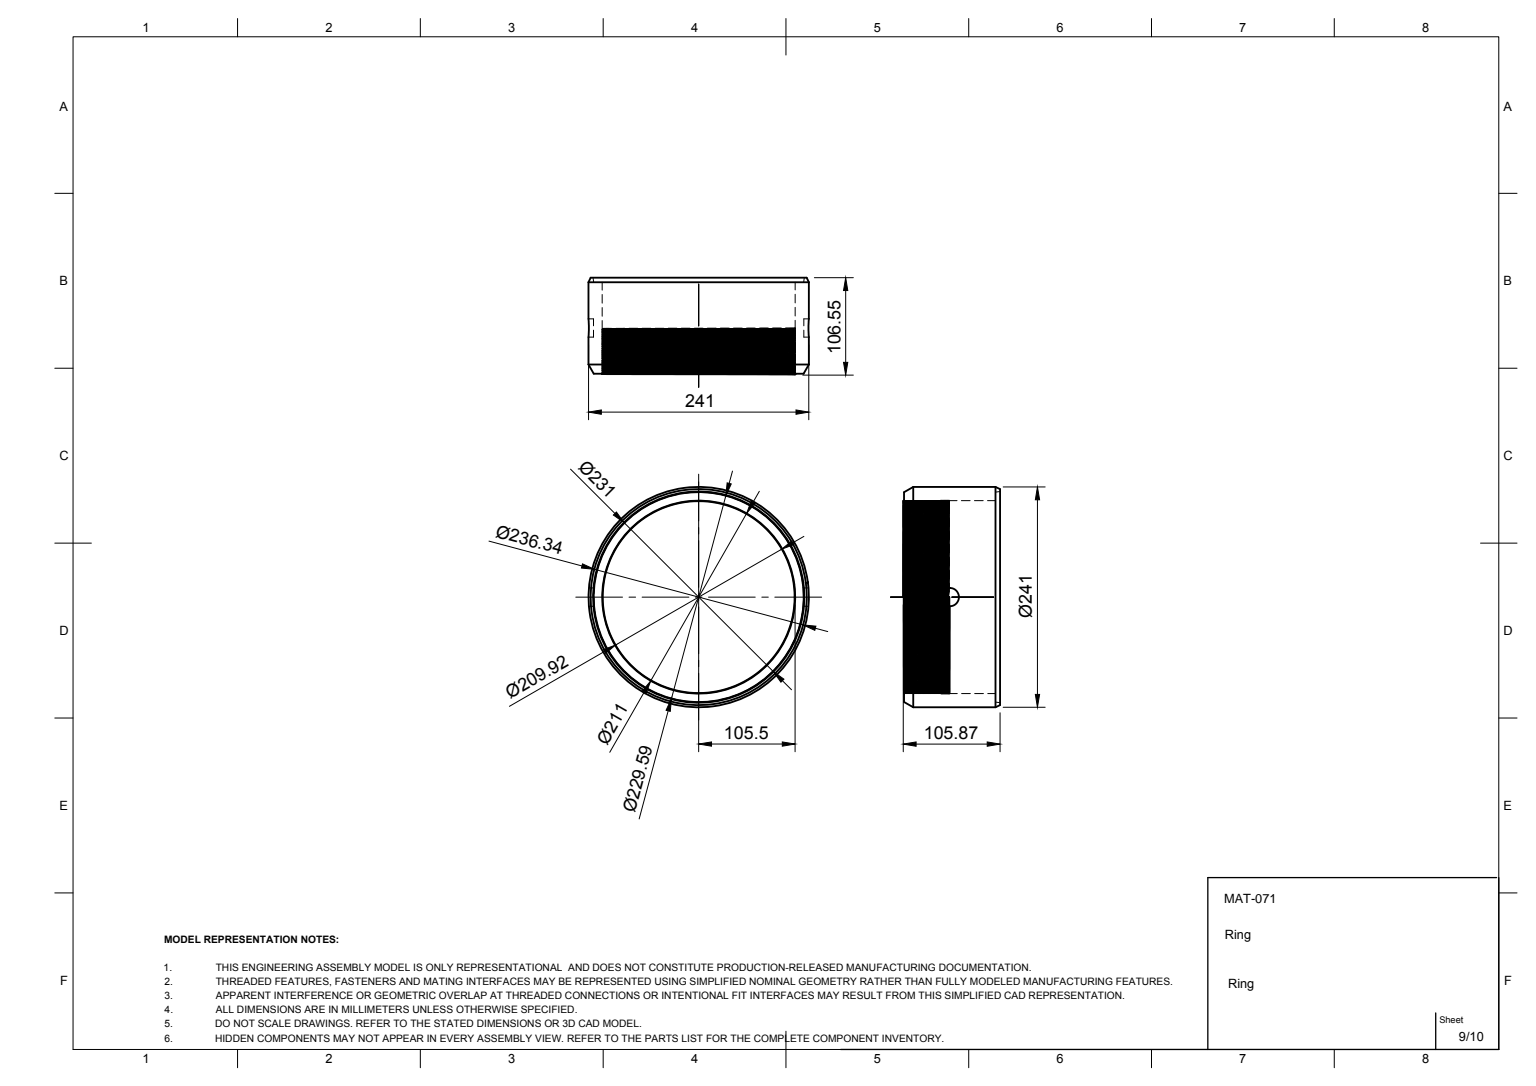
ISO-10303-21;
HEADER;
/* Generated by software containing ST-Developer
 * from STEP Tools, Inc. (www.steptools.com) 
 */

FILE_DESCRIPTION(
/* description */ (''),
/* implementation_level */ '2;1');

FILE_NAME(
/* name */ 'Ring.step',
/* time_stamp */ '2026-10-24T12:24:47-07:00',
/* author */ (''),
/* organization */ (''),
/* preprocessor_version */ 'ST-DEVELOPER v20.2',
/* originating_system */ 'Autodesk Translation Framework v15.15.0.0',
/* authorisation */ '');

FILE_SCHEMA (('AUTOMOTIVE_DESIGN { 1 0 10303 214 3 1 1 }'));
ENDSEC;

DATA;
#10=MECHANICAL_DESIGN_GEOMETRIC_PRESENTATION_REPRESENTATION('',(#57),#13594);
#45=SHAPE_REPRESENTATION_RELATIONSHIP('SRR','None',#13625,#51);
#51=ADVANCED_BREP_SHAPE_REPRESENTATION('',(#63),#13588);
#57=STYLED_ITEM('',(#13667),#63);
#63=MANIFOLD_SOLID_BREP('Ring',#2964);
#69=(
BOUNDED_SURFACE()
B_SPLINE_SURFACE(1,2,((#7782,#7783,#7784,#7785,#7786,#7787,#7788,#7789,
#7790,#7791,#7792,#7793,#7794,#7795,#7796,#7797,#7798,#7799,#7800,#7801,
#7802,#7803,#7804,#7805,#7806,#7807,#7808,#7809,#7810,#7811,#7812,#7813,
#7814,#7815,#7816,#7817,#7818,#7819,#7820,#7821,#7822,#7823,#7824,#7825,
#7826,#7827,#7828,#7829,#7830,#7831,#7832,#7833,#7834,#7835,#7836,#7837,
#7838,#7839,#7840,#7841,#7842,#7843,#7844,#7845,#7846,#7847,#7848,#7849,
#7850,#7851,#7852,#7853,#7854,#7855,#7856,#7857,#7858,#7859,#7860,#7861,
#7862,#7863,#7864,#7865,#7866,#7867,#7868,#7869,#7870,#7871,#7872,#7873,
#7874,#7875,#7876,#7877,#7878,#7879,#7880,#7881,#7882,#7883,#7884,#7885,
#7886,#7887,#7888,#7889,#7890,#7891,#7892,#7893,#7894,#7895,#7896,#7897,
#7898,#7899,#7900,#7901,#7902,#7903,#7904,#7905,#7906,#7907,#7908,#7909,
#7910,#7911,#7912,#7913,#7914,#7915,#7916,#7917,#7918,#7919,#7920,#7921,
#7922,#7923,#7924,#7925,#7926,#7927,#7928,#7929,#7930,#7931,#7932,#7933,
#7934,#7935,#7936,#7937,#7938,#7939,#7940,#7941,#7942,#7943,#7944,#7945,
#7946,#7947,#7948,#7949,#7950,#7951,#7952,#7953,#7954,#7955,#7956,#7957,
#7958,#7959,#7960,#7961,#7962,#7963,#7964,#7965,#7966,#7967,#7968,#7969,
#7970,#7971,#7972,#7973,#7974,#7975,#7976,#7977,#7978,#7979,#7980,#7981,
#7982,#7983,#7984,#7985,#7986,#7987,#7988,#7989,#7990,#7991,#7992,#7993,
#7994,#7995,#7996,#7997,#7998,#7999,#8000,#8001,#8002,#8003,#8004,#8005,
#8006,#8007,#8008,#8009,#8010,#8011,#8012,#8013,#8014,#8015,#8016,#8017,
#8018,#8019,#8020,#8021,#8022,#8023,#8024,#8025,#8026,#8027,#8028,#8029,
#8030,#8031,#8032,#8033,#8034,#8035,#8036,#8037,#8038,#8039,#8040,#8041,
#8042,#8043,#8044,#8045,#8046,#8047,#8048,#8049,#8050,#8051,#8052,#8053,
#8054,#8055,#8056,#8057,#8058,#8059,#8060,#8061,#8062,#8063,#8064,#8065,
#8066,#8067,#8068,#8069,#8070,#8071,#8072,#8073,#8074,#8075,#8076,#8077,
#8078,#8079,#8080,#8081,#8082,#8083,#8084,#8085,#8086,#8087,#8088,#8089,
#8090,#8091,#8092,#8093,#8094,#8095,#8096,#8097,#8098,#8099,#8100,#8101,
#8102,#8103,#8104,#8105,#8106,#8107,#8108,#8109,#8110,#8111,#8112,#8113,
#8114,#8115,#8116,#8117,#8118,#8119,#8120,#8121,#8122,#8123,#8124,#8125,
#8126,#8127,#8128,#8129,#8130,#8131,#8132,#8133,#8134,#8135,#8136,#8137,
#8138,#8139,#8140,#8141,#8142,#8143,#8144,#8145,#8146,#8147,#8148,#8149,
#8150,#8151,#8152,#8153,#8154,#8155,#8156,#8157,#8158,#8159,#8160,#8161,
#8162,#8163,#8164,#8165,#8166,#8167,#8168,#8169,#8170,#8171,#8172,#8173,
#8174,#8175,#8176,#8177,#8178,#8179,#8180,#8181,#8182,#8183,#8184,#8185,
#8186,#8187,#8188,#8189,#8190,#8191,#8192,#8193,#8194,#8195,#8196,#8197,
#8198,#8199,#8200,#8201,#8202,#8203,#8204,#8205,#8206,#8207,#8208,#8209,
#8210,#8211,#8212,#8213,#8214,#8215,#8216,#8217,#8218,#8219,#8220,#8221,
#8222,#8223,#8224,#8225,#8226,#8227,#8228,#8229,#8230,#8231,#8232,#8233,
#8234,#8235,#8236,#8237,#8238,#8239,#8240,#8241,#8242,#8243,#8244,#8245,
#8246,#8247,#8248,#8249,#8250,#8251,#8252,#8253,#8254,#8255,#8256,#8257,
#8258,#8259,#8260,#8261,#8262,#8263,#8264,#8265,#8266,#8267,#8268,#8269,
#8270,#8271,#8272,#8273,#8274,#8275,#8276,#8277,#8278,#8279,#8280,#8281,
#8282,#8283,#8284,#8285,#8286,#8287,#8288,#8289,#8290,#8291,#8292,#8293,
#8294,#8295,#8296,#8297,#8298,#8299,#8300,#8301,#8302,#8303,#8304,#8305,
#8306,#8307,#8308,#8309,#8310,#8311,#8312,#8313,#8314,#8315,#8316,#8317,
#8318,#8319,#8320,#8321,#8322,#8323,#8324,#8325,#8326,#8327,#8328,#8329,
#8330,#8331,#8332,#8333,#8334,#8335,#8336,#8337,#8338,#8339,#8340,#8341,
#8342,#8343,#8344,#8345,#8346,#8347,#8348,#8349,#8350,#8351,#8352,#8353,
#8354,#8355,#8356,#8357,#8358,#8359,#8360,#8361,#8362,#8363,#8364,#8365,
#8366,#8367,#8368,#8369,#8370,#8371,#8372,#8373,#8374,#8375,#8376,#8377,
#8378,#8379,#8380,#8381,#8382,#8383,#8384,#8385,#8386,#8387,#8388,#8389,
#8390,#8391,#8392,#8393,#8394,#8395,#8396,#8397,#8398,#8399,#8400,#8401,
#8402,#8403,#8404,#8405,#8406,#8407,#8408,#8409,#8410,#8411,#8412,#8413,
#8414,#8415,#8416,#8417,#8418,#8419,#8420,#8421,#8422,#8423,#8424,#8425,
#8426,#8427,#8428,#8429,#8430,#8431,#8432,#8433,#8434,#8435,#8436,#8437,
#8438,#8439,#8440,#8441,#8442,#8443,#8444,#8445,#8446,#8447,#8448,#8449,
#8450,#8451,#8452,#8453,#8454,#8455,#8456,#8457,#8458,#8459,#8460,#8461,
#8462,#8463,#8464,#8465,#8466,#8467,#8468,#8469,#8470,#8471,#8472,#8473,
#8474,#8475,#8476,#8477,#8478,#8479,#8480,#8481,#8482,#8483,#8484,#8485,
#8486,#8487,#8488,#8489,#8490,#8491,#8492,#8493,#8494,#8495,#8496,#8497,
#8498,#8499,#8500,#8501,#8502,#8503,#8504,#8505,#8506,#8507,#8508,#8509,
#8510,#8511,#8512,#8513,#8514,#8515,#8516,#8517,#8518,#8519,#8520,#8521,
#8522,#8523,#8524,#8525,#8526,#8527,#8528,#8529,#8530,#8531,#8532,#8533,
#8534,#8535,#8536,#8537,#8538,#8539,#8540,#8541,#8542,#8543,#8544,#8545,
#8546,#8547,#8548,#8549,#8550,#8551,#8552,#8553,#8554,#8555,#8556,#8557,
#8558,#8559,#8560,#8561,#8562,#8563,#8564,#8565,#8566,#8567,#8568,#8569,
#8570,#8571,#8572,#8573,#8574,#8575,#8576,#8577,#8578,#8579,#8580,#8581,
#8582),(#8583,#8584,#8585,#8586,#8587,#8588,#8589,#8590,#8591,#8592,#8593,
#8594,#8595,#8596,#8597,#8598,#8599,#8600,#8601,#8602,#8603,#8604,#8605,
#8606,#8607,#8608,#8609,#8610,#8611,#8612,#8613,#8614,#8615,#8616,#8617,
#8618,#8619,#8620,#8621,#8622,#8623,#8624,#8625,#8626,#8627,#8628,#8629,
#8630,#8631,#8632,#8633,#8634,#8635,#8636,#8637,#8638,#8639,#8640,#8641,
#8642,#8643,#8644,#8645,#8646,#8647,#8648,#8649,#8650,#8651,#8652,#8653,
#8654,#8655,#8656,#8657,#8658,#8659,#8660,#8661,#8662,#8663,#8664,#8665,
#8666,#8667,#8668,#8669,#8670,#8671,#8672,#8673,#8674,#8675,#8676,#8677,
#8678,#8679,#8680,#8681,#8682,#8683,#8684,#8685,#8686,#8687,#8688,#8689,
#8690,#8691,#8692,#8693,#8694,#8695,#8696,#8697,#8698,#8699,#8700,#8701,
#8702,#8703,#8704,#8705,#8706,#8707,#8708,#8709,#8710,#8711,#8712,#8713,
#8714,#8715,#8716,#8717,#8718,#8719,#8720,#8721,#8722,#8723,#8724,#8725,
#8726,#8727,#8728,#8729,#8730,#8731,#8732,#8733,#8734,#8735,#8736,#8737,
#8738,#8739,#8740,#8741,#8742,#8743,#8744,#8745,#8746,#8747,#8748,#8749,
#8750,#8751,#8752,#8753,#8754,#8755,#8756,#8757,#8758,#8759,#8760,#8761,
#8762,#8763,#8764,#8765,#8766,#8767,#8768,#8769,#8770,#8771,#8772,#8773,
#8774,#8775,#8776,#8777,#8778,#8779,#8780,#8781,#8782,#8783,#8784,#8785,
#8786,#8787,#8788,#8789,#8790,#8791,#8792,#8793,#8794,#8795,#8796,#8797,
#8798,#8799,#8800,#8801,#8802,#8803,#8804,#8805,#8806,#8807,#8808,#8809,
#8810,#8811,#8812,#8813,#8814,#8815,#8816,#8817,#8818,#8819,#8820,#8821,
#8822,#8823,#8824,#8825,#8826,#8827,#8828,#8829,#8830,#8831,#8832,#8833,
#8834,#8835,#8836,#8837,#8838,#8839,#8840,#8841,#8842,#8843,#8844,#8845,
#8846,#8847,#8848,#8849,#8850,#8851,#8852,#8853,#8854,#8855,#8856,#8857,
#8858,#8859,#8860,#8861,#8862,#8863,#8864,#8865,#8866,#8867,#8868,#8869,
#8870,#8871,#8872,#8873,#8874,#8875,#8876,#8877,#8878,#8879,#8880,#8881,
#8882,#8883,#8884,#8885,#8886,#8887,#8888,#8889,#8890,#8891,#8892,#8893,
#8894,#8895,#8896,#8897,#8898,#8899,#8900,#8901,#8902,#8903,#8904,#8905,
#8906,#8907,#8908,#8909,#8910,#8911,#8912,#8913,#8914,#8915,#8916,#8917,
#8918,#8919,#8920,#8921,#8922,#8923,#8924,#8925,#8926,#8927,#8928,#8929,
#8930,#8931,#8932,#8933,#8934,#8935,#8936,#8937,#8938,#8939,#8940,#8941,
#8942,#8943,#8944,#8945,#8946,#8947,#8948,#8949,#8950,#8951,#8952,#8953,
#8954,#8955,#8956,#8957,#8958,#8959,#8960,#8961,#8962,#8963,#8964,#8965,
#8966,#8967,#8968,#8969,#8970,#8971,#8972,#8973,#8974,#8975,#8976,#8977,
#8978,#8979,#8980,#8981,#8982,#8983,#8984,#8985,#8986,#8987,#8988,#8989,
#8990,#8991,#8992,#8993,#8994,#8995,#8996,#8997,#8998,#8999,#9000,#9001,
#9002,#9003,#9004,#9005,#9006,#9007,#9008,#9009,#9010,#9011,#9012,#9013,
#9014,#9015,#9016,#9017,#9018,#9019,#9020,#9021,#9022,#9023,#9024,#9025,
#9026,#9027,#9028,#9029,#9030,#9031,#9032,#9033,#9034,#9035,#9036,#9037,
#9038,#9039,#9040,#9041,#9042,#9043,#9044,#9045,#9046,#9047,#9048,#9049,
#9050,#9051,#9052,#9053,#9054,#9055,#9056,#9057,#9058,#9059,#9060,#9061,
#9062,#9063,#9064,#9065,#9066,#9067,#9068,#9069,#9070,#9071,#9072,#9073,
#9074,#9075,#9076,#9077,#9078,#9079,#9080,#9081,#9082,#9083,#9084,#9085,
#9086,#9087,#9088,#9089,#9090,#9091,#9092,#9093,#9094,#9095,#9096,#9097,
#9098,#9099,#9100,#9101,#9102,#9103,#9104,#9105,#9106,#9107,#9108,#9109,
#9110,#9111,#9112,#9113,#9114,#9115,#9116,#9117,#9118,#9119,#9120,#9121,
#9122,#9123,#9124,#9125,#9126,#9127,#9128,#9129,#9130,#9131,#9132,#9133,
#9134,#9135,#9136,#9137,#9138,#9139,#9140,#9141,#9142,#9143,#9144,#9145,
#9146,#9147,#9148,#9149,#9150,#9151,#9152,#9153,#9154,#9155,#9156,#9157,
#9158,#9159,#9160,#9161,#9162,#9163,#9164,#9165,#9166,#9167,#9168,#9169,
#9170,#9171,#9172,#9173,#9174,#9175,#9176,#9177,#9178,#9179,#9180,#9181,
#9182,#9183,#9184,#9185,#9186,#9187,#9188,#9189,#9190,#9191,#9192,#9193,
#9194,#9195,#9196,#9197,#9198,#9199,#9200,#9201,#9202,#9203,#9204,#9205,
#9206,#9207,#9208,#9209,#9210,#9211,#9212,#9213,#9214,#9215,#9216,#9217,
#9218,#9219,#9220,#9221,#9222,#9223,#9224,#9225,#9226,#9227,#9228,#9229,
#9230,#9231,#9232,#9233,#9234,#9235,#9236,#9237,#9238,#9239,#9240,#9241,
#9242,#9243,#9244,#9245,#9246,#9247,#9248,#9249,#9250,#9251,#9252,#9253,
#9254,#9255,#9256,#9257,#9258,#9259,#9260,#9261,#9262,#9263,#9264,#9265,
#9266,#9267,#9268,#9269,#9270,#9271,#9272,#9273,#9274,#9275,#9276,#9277,
#9278,#9279,#9280,#9281,#9282,#9283,#9284,#9285,#9286,#9287,#9288,#9289,
#9290,#9291,#9292,#9293,#9294,#9295,#9296,#9297,#9298,#9299,#9300,#9301,
#9302,#9303,#9304,#9305,#9306,#9307,#9308,#9309,#9310,#9311,#9312,#9313,
#9314,#9315,#9316,#9317,#9318,#9319,#9320,#9321,#9322,#9323,#9324,#9325,
#9326,#9327,#9328,#9329,#9330,#9331,#9332,#9333,#9334,#9335,#9336,#9337,
#9338,#9339,#9340,#9341,#9342,#9343,#9344,#9345,#9346,#9347,#9348,#9349,
#9350,#9351,#9352,#9353,#9354,#9355,#9356,#9357,#9358,#9359,#9360,#9361,
#9362,#9363,#9364,#9365,#9366,#9367,#9368,#9369,#9370,#9371,#9372,#9373,
#9374,#9375,#9376,#9377,#9378,#9379,#9380,#9381,#9382,#9383)),
 .UNSPECIFIED.,.F.,.F.,.F.)
B_SPLINE_SURFACE_WITH_KNOTS((2,2),(3,2,2,2,2,2,2,2,2,2,2,2,2,2,2,2,2,2,
2,2,2,2,2,2,2,2,2,2,2,2,2,2,2,2,2,2,2,2,2,2,2,2,2,2,2,2,2,2,2,2,2,2,2,2,
2,2,2,2,2,2,2,2,2,2,2,2,2,2,2,2,2,2,2,2,2,2,2,2,2,2,2,2,2,2,2,2,2,2,2,2,
2,2,2,2,2,2,2,2,2,2,2,2,2,2,2,2,2,2,2,2,2,2,2,2,2,2,2,2,2,2,2,2,2,2,2,2,
2,2,2,2,2,2,2,2,2,2,2,2,2,2,2,2,2,2,2,2,2,2,2,2,2,2,2,2,2,2,2,2,2,2,2,2,
2,2,2,2,2,2,2,2,2,2,2,2,2,2,2,2,2,2,2,2,2,2,2,2,2,2,2,2,2,2,2,2,2,2,2,2,
2,2,2,2,2,2,2,2,2,2,2,2,2,2,2,2,2,2,2,2,2,2,2,2,2,2,2,2,2,2,2,2,2,2,2,2,
2,2,2,2,2,2,2,2,2,2,2,2,2,2,2,2,2,2,2,2,2,2,2,2,2,2,2,2,2,2,2,2,2,2,2,2,
2,2,2,2,2,2,2,2,2,2,2,2,2,2,2,2,2,2,2,2,2,2,2,2,2,2,2,2,2,2,2,2,2,2,2,2,
2,2,2,2,2,2,2,2,2,2,2,2,2,2,2,2,2,2,2,2,2,2,2,2,2,2,2,2,2,2,2,2,2,2,2,2,
2,2,2,2,2,2,2,2,2,2,2,2,2,2,2,2,2,2,2,2,2,2,2,2,2,2,2,2,2,2,2,2,2,2,2,2,
2,2,2,2,2,2,2,2,2,2,2,2,2,2,2,2,2,2,2,2,2,2,3),(0.,1.),(0.,0.0025,0.005,
0.0075,0.01,0.0125,0.015,0.0175,0.02,0.0225,0.025,0.0275,0.03,0.0325,0.035,
0.0375,0.04,0.0425,0.045,0.0475,0.05,0.0525,0.055,0.0575,0.06,0.0625,0.065,
0.0675,0.07,0.0725,0.075,0.0775,0.08,0.0825,0.085,0.0875,0.09,0.0925,0.095,
0.0975,0.1,0.1025,0.105,0.1075,0.11,0.1125,0.115,0.1175,0.12,0.1225,0.125,
0.1275,0.13,0.1325,0.135,0.1375,0.14,0.1425,0.145,0.1475,0.15,0.1525,0.155,
0.1575,0.16,0.1625,0.165,0.1675,0.17,0.1725,0.175,0.1775,0.18,0.1825,0.185,
0.1875,0.19,0.1925,0.195,0.1975,0.2,0.2025,0.205,0.2075,0.21,0.2125,0.215,
0.2175,0.22,0.2225,0.225,0.2275,0.23,0.2325,0.235,0.2375,0.24,0.2425,0.245,
0.2475,0.25,0.2525,0.255,0.2575,0.26,0.2625,0.265,0.2675,0.27,0.2725,0.275,
0.2775,0.28,0.2825,0.285,0.2875,0.29,0.2925,0.295,0.2975,0.3,0.3025,0.305,
0.3075,0.31,0.3125,0.315,0.3175,0.32,0.3225,0.325,0.3275,0.33,0.3325,0.335,
0.3375,0.34,0.3425,0.345,0.3475,0.35,0.3525,0.355,0.3575,0.36,0.3625,0.365,
0.3675,0.37,0.3725,0.375,0.3775,0.38,0.3825,0.385,0.3875,0.39,0.3925,0.395,
0.3975,0.4,0.4025,0.405,0.4075,0.41,0.4125,0.415,0.4175,0.42,0.4225,0.425,
0.4275,0.43,0.4325,0.435,0.4375,0.44,0.4425,0.445,0.4475,0.45,0.4525,0.455,
0.4575,0.46,0.4625,0.465,0.4675,0.47,0.4725,0.475,0.4775,0.48,0.4825,0.485,
0.4875,0.49,0.4925,0.495,0.4975,0.5,0.5025,0.505,0.5075,0.51,0.5125,0.515,
0.5175,0.52,0.5225,0.525,0.5275,0.53,0.5325,0.535,0.5375,0.54,0.5425,0.545,
0.5475,0.55,0.5525,0.555,0.5575,0.56,0.5625,0.565,0.5675,0.57,0.5725,0.575,
0.5775,0.58,0.5825,0.585,0.5875,0.59,0.5925,0.595,0.5975,0.6,0.6025,0.605,
0.6075,0.61,0.6125,0.615,0.6175,0.62,0.6225,0.625,0.6275,0.63,0.6325,0.635,
0.6375,0.64,0.6425,0.645,0.6475,0.65,0.6525,0.655,0.6575,0.66,0.6625,0.665,
0.6675,0.67,0.6725,0.675,0.6775,0.68,0.6825,0.685,0.6875,0.69,0.6925,0.695,
0.6975,0.7,0.7025,0.705,0.7075,0.71,0.7125,0.715,0.7175,0.72,0.7225,0.725,
0.7275,0.73,0.7325,0.735,0.7375,0.74,0.7425,0.745,0.7475,0.75,0.7525,0.755,
0.7575,0.76,0.7625,0.765,0.7675,0.77,0.7725,0.775,0.7775,0.78,0.7825,0.785,
0.7875,0.79,0.7925,0.795,0.7975,0.8,0.8025,0.805,0.8075,0.81,0.8125,0.815,
0.8175,0.82,0.8225,0.825,0.8275,0.83,0.8325,0.835,0.8375,0.84,0.8425,0.845,
0.8475,0.85,0.8525,0.855,0.8575,0.86,0.8625,0.865,0.8675,0.87,0.8725,0.875,
0.8775,0.88,0.8825,0.885,0.8875,0.89,0.8925,0.895,0.8975,0.9,0.9025,0.905,
0.9075,0.91,0.9125,0.915,0.9175,0.92,0.9225,0.925,0.9275,0.93,0.9325,0.935,
0.9375,0.94,0.9425,0.945,0.9475,0.95,0.9525,0.955,0.9575,0.96,0.9625,0.965,
0.9675,0.97,0.9725,0.975,0.9775,0.98,0.9825,0.985,0.9875,0.99,0.9925,0.995,
0.9975,1.),.UNSPECIFIED.)
GEOMETRIC_REPRESENTATION_ITEM()
RATIONAL_B_SPLINE_SURFACE(((1.,0.923879532511287,1.,0.923879532511287,1.,
0.923879532511287,1.,0.923879532511287,1.,0.923879532511287,1.,0.923879532511287,
1.,0.923879532511287,1.,0.923879532511287,1.,0.923879532511287,1.,0.923879532511287,
1.,0.923879532511287,1.,0.923879532511287,1.,0.923879532511287,1.,0.923879532511287,
1.,0.923879532511287,1.,0.923879532511287,1.,0.923879532511287,1.,0.923879532511287,
1.,0.923879532511287,1.,0.923879532511287,1.,0.923879532511287,1.,0.923879532511287,
1.,0.923879532511287,1.,0.923879532511287,1.,0.923879532511287,1.,0.923879532511287,
1.,0.923879532511287,1.,0.923879532511287,1.,0.923879532511287,1.,0.923879532511287,
1.,0.923879532511287,1.,0.923879532511287,1.,0.923879532511287,1.,0.923879532511287,
1.,0.923879532511287,1.,0.923879532511287,1.,0.923879532511287,1.,0.923879532511287,
1.,0.923879532511287,1.,0.923879532511287,1.,0.923879532511287,1.,0.923879532511287,
1.,0.923879532511287,1.,0.923879532511287,1.,0.923879532511287,1.,0.923879532511287,
1.,0.923879532511287,1.,0.923879532511287,1.,0.923879532511287,1.,0.923879532511287,
1.,0.923879532511287,1.,0.923879532511287,1.,0.923879532511287,1.,0.923879532511287,
1.,0.923879532511287,1.,0.923879532511287,1.,0.923879532511287,1.,0.923879532511287,
1.,0.923879532511287,1.,0.923879532511287,1.,0.923879532511287,1.,0.923879532511287,
1.,0.923879532511287,1.,0.923879532511287,1.,0.923879532511287,1.,0.923879532511287,
1.,0.923879532511287,1.,0.923879532511287,1.,0.923879532511287,1.,0.923879532511287,
1.,0.923879532511287,1.,0.923879532511287,1.,0.923879532511287,1.,0.923879532511287,
1.,0.923879532511287,1.,0.923879532511287,1.,0.923879532511287,1.,0.923879532511287,
1.,0.923879532511287,1.,0.923879532511287,1.,0.923879532511287,1.,0.923879532511287,
1.,0.923879532511287,1.,0.923879532511287,1.,0.923879532511287,1.,0.923879532511287,
1.,0.923879532511287,1.,0.923879532511287,1.,0.923879532511287,1.,0.923879532511287,
1.,0.923879532511287,1.,0.923879532511287,1.,0.923879532511287,1.,0.923879532511287,
1.,0.923879532511287,1.,0.923879532511287,1.,0.923879532511287,1.,0.923879532511287,
1.,0.923879532511287,1.,0.923879532511287,1.,0.923879532511287,1.,0.923879532511287,
1.,0.923879532511287,1.,0.923879532511287,1.,0.923879532511287,1.,0.923879532511287,
1.,0.923879532511287,1.,0.923879532511287,1.,0.923879532511287,1.,0.923879532511287,
1.,0.923879532511287,1.,0.923879532511287,1.,0.923879532511287,1.,0.923879532511287,
1.,0.923879532511287,1.,0.923879532511287,1.,0.923879532511287,1.,0.923879532511287,
1.,0.923879532511287,1.,0.923879532511287,1.,0.923879532511287,1.,0.923879532511287,
1.,0.923879532511287,1.,0.923879532511287,1.,0.923879532511287,1.,0.923879532511287,
1.,0.923879532511287,1.,0.923879532511287,1.,0.923879532511287,1.,0.923879532511287,
1.,0.923879532511287,1.,0.923879532511287,1.,0.923879532511287,1.,0.923879532511287,
1.,0.923879532511287,1.,0.923879532511287,1.,0.923879532511287,1.,0.923879532511287,
1.,0.923879532511287,1.,0.923879532511287,1.,0.923879532511287,1.,0.923879532511287,
1.,0.923879532511287,1.,0.923879532511287,1.,0.923879532511287,1.,0.923879532511287,
1.,0.923879532511287,1.,0.923879532511287,1.,0.923879532511287,1.,0.923879532511287,
1.,0.923879532511287,1.,0.923879532511287,1.,0.923879532511287,1.,0.923879532511287,
1.,0.923879532511287,1.,0.923879532511287,1.,0.923879532511287,1.,0.923879532511287,
1.,0.923879532511287,1.,0.923879532511287,1.,0.923879532511287,1.,0.923879532511287,
1.,0.923879532511287,1.,0.923879532511287,1.,0.923879532511287,1.,0.923879532511287,
1.,0.923879532511287,1.,0.923879532511287,1.,0.923879532511287,1.,0.923879532511287,
1.,0.923879532511287,1.,0.923879532511287,1.,0.923879532511287,1.,0.923879532511287,
1.,0.923879532511287,1.,0.923879532511287,1.,0.923879532511287,1.,0.923879532511287,
1.,0.923879532511287,1.,0.923879532511287,1.,0.923879532511287,1.,0.923879532511287,
1.,0.923879532511287,1.,0.923879532511287,1.,0.923879532511287,1.,0.923879532511287,
1.,0.923879532511287,1.,0.923879532511287,1.,0.923879532511287,1.,0.923879532511287,
1.,0.923879532511287,1.,0.923879532511287,1.,0.923879532511287,1.,0.923879532511287,
1.,0.923879532511287,1.,0.923879532511287,1.,0.923879532511287,1.,0.923879532511287,
1.,0.923879532511287,1.,0.923879532511287,1.,0.923879532511287,1.,0.923879532511287,
1.,0.923879532511287,1.,0.923879532511287,1.,0.923879532511287,1.,0.923879532511287,
1.,0.923879532511287,1.,0.923879532511287,1.,0.923879532511287,1.,0.923879532511287,
1.,0.923879532511287,1.,0.923879532511287,1.,0.923879532511287,1.,0.923879532511287,
1.,0.923879532511287,1.,0.923879532511287,1.,0.923879532511287,1.,0.923879532511287,
1.,0.923879532511287,1.,0.923879532511287,1.,0.923879532511287,1.,0.923879532511287,
1.,0.923879532511287,1.,0.923879532511287,1.,0.923879532511287,1.,0.923879532511287,
1.,0.923879532511287,1.,0.923879532511287,1.,0.923879532511287,1.,0.923879532511287,
1.,0.923879532511287,1.,0.923879532511287,1.,0.923879532511287,1.,0.923879532511287,
1.,0.923879532511287,1.,0.923879532511287,1.,0.923879532511287,1.,0.923879532511287,
1.,0.923879532511287,1.,0.923879532511287,1.,0.923879532511287,1.,0.923879532511287,
1.,0.923879532511287,1.,0.923879532511287,1.,0.923879532511287,1.,0.923879532511287,
1.,0.923879532511287,1.,0.923879532511287,1.,0.923879532511287,1.,0.923879532511287,
1.,0.923879532511287,1.,0.923879532511287,1.,0.923879532511287,1.,0.923879532511287,
1.,0.923879532511287,1.,0.923879532511287,1.,0.923879532511287,1.,0.923879532511287,
1.,0.923879532511287,1.,0.923879532511287,1.,0.923879532511287,1.,0.923879532511287,
1.,0.923879532511287,1.,0.923879532511287,1.,0.923879532511287,1.,0.923879532511287,
1.,0.923879532511287,1.,0.923879532511287,1.,0.923879532511287,1.,0.923879532511287,
1.,0.923879532511287,1.,0.923879532511287,1.,0.923879532511287,1.,0.923879532511287,
1.,0.923879532511287,1.,0.923879532511287,1.,0.923879532511287,1.,0.923879532511287,
1.,0.923879532511287,1.,0.923879532511287,1.,0.923879532511287,1.,0.923879532511287,
1.,0.923879532511287,1.,0.923879532511287,1.,0.923879532511287,1.,0.923879532511287,
1.,0.923879532511287,1.,0.923879532511287,1.,0.923879532511287,1.,0.923879532511287,
1.,0.923879532511287,1.,0.923879532511287,1.,0.923879532511287,1.,0.923879532511287,
1.,0.923879532511287,1.,0.923879532511287,1.,0.923879532511287,1.,0.923879532511287,
1.,0.923879532511287,1.,0.923879532511287,1.,0.923879532511287,1.,0.923879532511287,
1.,0.923879532511287,1.,0.923879532511287,1.,0.923879532511287,1.,0.923879532511287,
1.,0.923879532511287,1.,0.923879532511287,1.,0.923879532511287,1.,0.923879532511287,
1.,0.923879532511287,1.,0.923879532511287,1.,0.923879532511287,1.,0.923879532511287,
1.,0.923879532511287,1.,0.923879532511287,1.,0.923879532511287,1.,0.923879532511287,
1.,0.923879532511287,1.,0.923879532511287,1.,0.923879532511287,1.,0.923879532511287,
1.,0.923879532511287,1.,0.923879532511287,1.,0.923879532511287,1.,0.923879532511287,
1.,0.923879532511287,1.,0.923879532511287,1.,0.923879532511287,1.,0.923879532511287,
1.,0.923879532511287,1.,0.923879532511287,1.,0.923879532511287,1.,0.923879532511287,
1.,0.923879532511287,1.,0.923879532511287,1.,0.923879532511287,1.,0.923879532511287,
1.,0.923879532511287,1.,0.923879532511287,1.,0.923879532511287,1.,0.923879532511287,
1.,0.923879532511287,1.,0.923879532511287,1.,0.923879532511287,1.,0.923879532511287,
1.,0.923879532511287,1.,0.923879532511287,1.,0.923879532511287,1.,0.923879532511287,
1.,0.923879532511287,1.,0.923879532511287,1.,0.923879532511287,1.,0.923879532511287,
1.,0.923879532511287,1.,0.923879532511287,1.,0.923879532511287,1.,0.923879532511287,
1.,0.923879532511287,1.,0.923879532511287,1.,0.923879532511287,1.,0.923879532511287,
1.,0.923879532511287,1.,0.923879532511287,1.,0.923879532511287,1.,0.923879532511287,
1.,0.923879532511287,1.,0.923879532511287,1.,0.923879532511287,1.,0.923879532511287,
1.,0.923879532511287,1.,0.923879532511287,1.,0.923879532511287,1.,0.923879532511287,
1.,0.923879532511287,1.,0.923879532511287,1.,0.923879532511287,1.,0.923879532511287,
1.,0.923879532511287,1.,0.923879532511287,1.,0.923879532511287,1.,0.923879532511287,
1.,0.923879532511287,1.,0.923879532511287,1.,0.923879532511287,1.,0.923879532511287,
1.,0.923879532511287,1.,0.923879532511287,1.,0.923879532511287,1.,0.923879532511287,
1.,0.923879532511287,1.,0.923879532511287,1.,0.923879532511287,1.,0.923879532511287,
1.,0.923879532511287,1.,0.923879532511287,1.,0.923879532511287,1.,0.923879532511287,
1.,0.923879532511287,1.,0.923879532511287,1.),(1.,0.923879532511287,1.,
0.923879532511287,1.,0.923879532511287,1.,0.923879532511287,1.,0.923879532511287,
1.,0.923879532511287,1.,0.923879532511287,1.,0.923879532511287,1.,0.923879532511287,
1.,0.923879532511287,1.,0.923879532511287,1.,0.923879532511287,1.,0.923879532511287,
1.,0.923879532511287,1.,0.923879532511287,1.,0.923879532511287,1.,0.923879532511287,
1.,0.923879532511287,1.,0.923879532511287,1.,0.923879532511287,1.,0.923879532511287,
1.,0.923879532511287,1.,0.923879532511287,1.,0.923879532511287,1.,0.923879532511287,
1.,0.923879532511287,1.,0.923879532511287,1.,0.923879532511287,1.,0.923879532511287,
1.,0.923879532511287,1.,0.923879532511287,1.,0.923879532511287,1.,0.923879532511287,
1.,0.923879532511287,1.,0.923879532511287,1.,0.923879532511287,1.,0.923879532511287,
1.,0.923879532511287,1.,0.923879532511287,1.,0.923879532511287,1.,0.923879532511287,
1.,0.923879532511287,1.,0.923879532511287,1.,0.923879532511287,1.,0.923879532511287,
1.,0.923879532511287,1.,0.923879532511287,1.,0.923879532511287,1.,0.923879532511287,
1.,0.923879532511287,1.,0.923879532511287,1.,0.923879532511287,1.,0.923879532511287,
1.,0.923879532511287,1.,0.923879532511287,1.,0.923879532511287,1.,0.923879532511287,
1.,0.923879532511287,1.,0.923879532511287,1.,0.923879532511287,1.,0.923879532511287,
1.,0.923879532511287,1.,0.923879532511287,1.,0.923879532511287,1.,0.923879532511287,
1.,0.923879532511287,1.,0.923879532511287,1.,0.923879532511287,1.,0.923879532511287,
1.,0.923879532511287,1.,0.923879532511287,1.,0.923879532511287,1.,0.923879532511287,
1.,0.923879532511287,1.,0.923879532511287,1.,0.923879532511287,1.,0.923879532511287,
1.,0.923879532511287,1.,0.923879532511287,1.,0.923879532511287,1.,0.923879532511287,
1.,0.923879532511287,1.,0.923879532511287,1.,0.923879532511287,1.,0.923879532511287,
1.,0.923879532511287,1.,0.923879532511287,1.,0.923879532511287,1.,0.923879532511287,
1.,0.923879532511287,1.,0.923879532511287,1.,0.923879532511287,1.,0.923879532511287,
1.,0.923879532511287,1.,0.923879532511287,1.,0.923879532511287,1.,0.923879532511287,
1.,0.923879532511287,1.,0.923879532511287,1.,0.923879532511287,1.,0.923879532511287,
1.,0.923879532511287,1.,0.923879532511287,1.,0.923879532511287,1.,0.923879532511287,
1.,0.923879532511287,1.,0.923879532511287,1.,0.923879532511287,1.,0.923879532511287,
1.,0.923879532511287,1.,0.923879532511287,1.,0.923879532511287,1.,0.923879532511287,
1.,0.923879532511287,1.,0.923879532511287,1.,0.923879532511287,1.,0.923879532511287,
1.,0.923879532511287,1.,0.923879532511287,1.,0.923879532511287,1.,0.923879532511287,
1.,0.923879532511287,1.,0.923879532511287,1.,0.923879532511287,1.,0.923879532511287,
1.,0.923879532511287,1.,0.923879532511287,1.,0.923879532511287,1.,0.923879532511287,
1.,0.923879532511287,1.,0.923879532511287,1.,0.923879532511287,1.,0.923879532511287,
1.,0.923879532511287,1.,0.923879532511287,1.,0.923879532511287,1.,0.923879532511287,
1.,0.923879532511287,1.,0.923879532511287,1.,0.923879532511287,1.,0.923879532511287,
1.,0.923879532511287,1.,0.923879532511287,1.,0.923879532511287,1.,0.923879532511287,
1.,0.923879532511287,1.,0.923879532511287,1.,0.923879532511287,1.,0.923879532511287,
1.,0.923879532511287,1.,0.923879532511287,1.,0.923879532511287,1.,0.923879532511287,
1.,0.923879532511287,1.,0.923879532511287,1.,0.923879532511287,1.,0.923879532511287,
1.,0.923879532511287,1.,0.923879532511287,1.,0.923879532511287,1.,0.923879532511287,
1.,0.923879532511287,1.,0.923879532511287,1.,0.923879532511287,1.,0.923879532511287,
1.,0.923879532511287,1.,0.923879532511287,1.,0.923879532511287,1.,0.923879532511287,
1.,0.923879532511287,1.,0.923879532511287,1.,0.923879532511287,1.,0.923879532511287,
1.,0.923879532511287,1.,0.923879532511287,1.,0.923879532511287,1.,0.923879532511287,
1.,0.923879532511287,1.,0.923879532511287,1.,0.923879532511287,1.,0.923879532511287,
1.,0.923879532511287,1.,0.923879532511287,1.,0.923879532511287,1.,0.923879532511287,
1.,0.923879532511287,1.,0.923879532511287,1.,0.923879532511287,1.,0.923879532511287,
1.,0.923879532511287,1.,0.923879532511287,1.,0.923879532511287,1.,0.923879532511287,
1.,0.923879532511287,1.,0.923879532511287,1.,0.923879532511287,1.,0.923879532511287,
1.,0.923879532511287,1.,0.923879532511287,1.,0.923879532511287,1.,0.923879532511287,
1.,0.923879532511287,1.,0.923879532511287,1.,0.923879532511287,1.,0.923879532511287,
1.,0.923879532511287,1.,0.923879532511287,1.,0.923879532511287,1.,0.923879532511287,
1.,0.923879532511287,1.,0.923879532511287,1.,0.923879532511287,1.,0.923879532511287,
1.,0.923879532511287,1.,0.923879532511287,1.,0.923879532511287,1.,0.923879532511287,
1.,0.923879532511287,1.,0.923879532511287,1.,0.923879532511287,1.,0.923879532511287,
1.,0.923879532511287,1.,0.923879532511287,1.,0.923879532511287,1.,0.923879532511287,
1.,0.923879532511287,1.,0.923879532511287,1.,0.923879532511287,1.,0.923879532511287,
1.,0.923879532511287,1.,0.923879532511287,1.,0.923879532511287,1.,0.923879532511287,
1.,0.923879532511287,1.,0.923879532511287,1.,0.923879532511287,1.,0.923879532511287,
1.,0.923879532511287,1.,0.923879532511287,1.,0.923879532511287,1.,0.923879532511287,
1.,0.923879532511287,1.,0.923879532511287,1.,0.923879532511287,1.,0.923879532511287,
1.,0.923879532511287,1.,0.923879532511287,1.,0.923879532511287,1.,0.923879532511287,
1.,0.923879532511287,1.,0.923879532511287,1.,0.923879532511287,1.,0.923879532511287,
1.,0.923879532511287,1.,0.923879532511287,1.,0.923879532511287,1.,0.923879532511287,
1.,0.923879532511287,1.,0.923879532511287,1.,0.923879532511287,1.,0.923879532511287,
1.,0.923879532511287,1.,0.923879532511287,1.,0.923879532511287,1.,0.923879532511287,
1.,0.923879532511287,1.,0.923879532511287,1.,0.923879532511287,1.,0.923879532511287,
1.,0.923879532511287,1.,0.923879532511287,1.,0.923879532511287,1.,0.923879532511287,
1.,0.923879532511287,1.,0.923879532511287,1.,0.923879532511287,1.,0.923879532511287,
1.,0.923879532511287,1.,0.923879532511287,1.,0.923879532511287,1.,0.923879532511287,
1.,0.923879532511287,1.,0.923879532511287,1.,0.923879532511287,1.,0.923879532511287,
1.,0.923879532511287,1.,0.923879532511287,1.,0.923879532511287,1.,0.923879532511287,
1.,0.923879532511287,1.,0.923879532511287,1.,0.923879532511287,1.,0.923879532511287,
1.,0.923879532511287,1.,0.923879532511287,1.,0.923879532511287,1.,0.923879532511287,
1.,0.923879532511287,1.,0.923879532511287,1.,0.923879532511287,1.,0.923879532511287,
1.,0.923879532511287,1.,0.923879532511287,1.,0.923879532511287,1.,0.923879532511287,
1.,0.923879532511287,1.,0.923879532511287,1.,0.923879532511287,1.,0.923879532511287,
1.,0.923879532511287,1.,0.923879532511287,1.,0.923879532511287,1.,0.923879532511287,
1.,0.923879532511287,1.,0.923879532511287,1.,0.923879532511287,1.,0.923879532511287,
1.,0.923879532511287,1.,0.923879532511287,1.,0.923879532511287,1.,0.923879532511287,
1.,0.923879532511287,1.,0.923879532511287,1.,0.923879532511287,1.,0.923879532511287,
1.,0.923879532511287,1.,0.923879532511287,1.,0.923879532511287,1.,0.923879532511287,
1.,0.923879532511287,1.,0.923879532511287,1.,0.923879532511287,1.,0.923879532511287,
1.,0.923879532511287,1.,0.923879532511287,1.,0.923879532511287,1.,0.923879532511287,
1.,0.923879532511287,1.,0.923879532511287,1.,0.923879532511287,1.,0.923879532511287,
1.,0.923879532511287,1.,0.923879532511287,1.,0.923879532511287,1.,0.923879532511287,
1.,0.923879532511287,1.,0.923879532511287,1.,0.923879532511287,1.,0.923879532511287,
1.,0.923879532511287,1.,0.923879532511287,1.,0.923879532511287,1.,0.923879532511287,
1.,0.923879532511287,1.,0.923879532511287,1.,0.923879532511287,1.,0.923879532511287,
1.,0.923879532511287,1.,0.923879532511287,1.,0.923879532511287,1.,0.923879532511287,
1.,0.923879532511287,1.,0.923879532511287,1.,0.923879532511287,1.,0.923879532511287,
1.,0.923879532511287,1.,0.923879532511287,1.,0.923879532511287,1.,0.923879532511287,
1.,0.923879532511287,1.,0.923879532511287,1.,0.923879532511287,1.,0.923879532511287,
1.,0.923879532511287,1.,0.923879532511287,1.,0.923879532511287,1.,0.923879532511287,
1.,0.923879532511287,1.,0.923879532511287,1.,0.923879532511287,1.,0.923879532511287,
1.,0.923879532511287,1.,0.923879532511287,1.,0.923879532511287,1.,0.923879532511287,
1.,0.923879532511287,1.,0.923879532511287,1.,0.923879532511287,1.,0.923879532511287,
1.,0.923879532511287,1.,0.923879532511287,1.,0.923879532511287,1.,0.923879532511287,
1.,0.923879532511287,1.,0.923879532511287,1.,0.923879532511287,1.,0.923879532511287,
1.,0.923879532511287,1.,0.923879532511287,1.,0.923879532511287,1.)))
REPRESENTATION_ITEM('')
SURFACE()
);
#70=(
BOUNDED_SURFACE()
B_SPLINE_SURFACE(1,2,((#9419,#9420,#9421,#9422,#9423,#9424,#9425,#9426,
#9427,#9428,#9429,#9430,#9431,#9432,#9433,#9434,#9435,#9436,#9437,#9438,
#9439,#9440,#9441,#9442,#9443,#9444,#9445,#9446,#9447,#9448,#9449,#9450,
#9451,#9452,#9453,#9454,#9455,#9456,#9457,#9458,#9459,#9460,#9461,#9462,
#9463,#9464,#9465,#9466,#9467,#9468,#9469,#9470,#9471,#9472,#9473,#9474,
#9475,#9476,#9477,#9478,#9479,#9480,#9481,#9482,#9483,#9484,#9485,#9486,
#9487,#9488,#9489,#9490,#9491,#9492,#9493,#9494,#9495,#9496,#9497,#9498,
#9499,#9500,#9501,#9502,#9503,#9504,#9505,#9506,#9507,#9508,#9509,#9510,
#9511,#9512,#9513,#9514,#9515,#9516,#9517,#9518,#9519,#9520,#9521,#9522,
#9523,#9524,#9525,#9526,#9527,#9528,#9529,#9530,#9531,#9532,#9533,#9534,
#9535,#9536,#9537,#9538,#9539,#9540,#9541,#9542,#9543,#9544,#9545,#9546,
#9547,#9548,#9549,#9550,#9551,#9552,#9553,#9554,#9555,#9556,#9557,#9558,
#9559,#9560,#9561,#9562,#9563,#9564,#9565,#9566,#9567,#9568,#9569,#9570,
#9571,#9572,#9573,#9574,#9575,#9576,#9577,#9578,#9579,#9580,#9581,#9582,
#9583,#9584,#9585,#9586,#9587,#9588,#9589,#9590,#9591,#9592,#9593,#9594,
#9595,#9596,#9597,#9598,#9599,#9600,#9601,#9602,#9603,#9604,#9605,#9606,
#9607,#9608,#9609,#9610,#9611,#9612,#9613,#9614,#9615,#9616,#9617,#9618,
#9619,#9620,#9621,#9622,#9623,#9624,#9625,#9626,#9627,#9628,#9629,#9630,
#9631,#9632,#9633,#9634,#9635,#9636,#9637,#9638,#9639,#9640,#9641,#9642,
#9643,#9644,#9645,#9646,#9647,#9648,#9649,#9650,#9651,#9652,#9653,#9654,
#9655,#9656,#9657,#9658,#9659,#9660,#9661,#9662,#9663,#9664,#9665,#9666,
#9667,#9668,#9669,#9670,#9671,#9672,#9673,#9674,#9675,#9676,#9677,#9678,
#9679,#9680,#9681,#9682,#9683,#9684,#9685,#9686,#9687,#9688,#9689,#9690,
#9691,#9692,#9693,#9694,#9695,#9696,#9697,#9698,#9699,#9700,#9701,#9702,
#9703,#9704,#9705,#9706,#9707,#9708,#9709,#9710,#9711,#9712,#9713,#9714,
#9715,#9716,#9717,#9718,#9719,#9720,#9721,#9722,#9723,#9724,#9725,#9726,
#9727,#9728,#9729,#9730,#9731,#9732,#9733,#9734,#9735,#9736,#9737,#9738,
#9739,#9740,#9741,#9742,#9743,#9744,#9745,#9746,#9747,#9748,#9749,#9750,
#9751,#9752,#9753,#9754,#9755,#9756,#9757,#9758,#9759,#9760,#9761,#9762,
#9763,#9764,#9765,#9766,#9767,#9768,#9769,#9770,#9771,#9772,#9773,#9774,
#9775,#9776,#9777,#9778,#9779,#9780,#9781,#9782,#9783,#9784,#9785,#9786,
#9787,#9788,#9789,#9790,#9791,#9792,#9793,#9794,#9795,#9796,#9797,#9798,
#9799,#9800,#9801,#9802,#9803,#9804,#9805,#9806,#9807,#9808,#9809,#9810,
#9811,#9812,#9813,#9814,#9815,#9816,#9817,#9818,#9819,#9820,#9821,#9822,
#9823,#9824,#9825,#9826,#9827,#9828,#9829,#9830,#9831,#9832,#9833,#9834,
#9835,#9836,#9837,#9838,#9839,#9840,#9841,#9842,#9843,#9844,#9845,#9846,
#9847,#9848,#9849,#9850,#9851,#9852,#9853,#9854,#9855,#9856,#9857,#9858,
#9859,#9860,#9861,#9862,#9863,#9864,#9865,#9866,#9867,#9868,#9869,#9870,
#9871,#9872,#9873,#9874,#9875,#9876,#9877,#9878,#9879,#9880,#9881,#9882,
#9883,#9884,#9885,#9886,#9887,#9888,#9889,#9890,#9891,#9892,#9893,#9894,
#9895,#9896,#9897,#9898,#9899,#9900,#9901,#9902,#9903,#9904,#9905,#9906,
#9907,#9908,#9909,#9910,#9911,#9912,#9913,#9914,#9915,#9916,#9917,#9918,
#9919,#9920,#9921,#9922,#9923,#9924,#9925,#9926,#9927,#9928,#9929,#9930,
#9931,#9932,#9933,#9934,#9935,#9936,#9937,#9938,#9939,#9940,#9941,#9942,
#9943,#9944,#9945,#9946,#9947,#9948,#9949,#9950,#9951,#9952,#9953,#9954,
#9955,#9956,#9957,#9958,#9959,#9960,#9961,#9962,#9963,#9964,#9965,#9966,
#9967,#9968,#9969,#9970,#9971,#9972,#9973,#9974,#9975,#9976,#9977,#9978,
#9979,#9980,#9981,#9982,#9983,#9984,#9985,#9986,#9987,#9988,#9989,#9990,
#9991,#9992,#9993,#9994,#9995,#9996,#9997,#9998,#9999,#10000,#10001,#10002,
#10003,#10004,#10005,#10006,#10007,#10008,#10009,#10010,#10011,#10012,#10013,
#10014,#10015,#10016,#10017,#10018,#10019,#10020,#10021,#10022,#10023,#10024,
#10025,#10026,#10027,#10028,#10029,#10030,#10031,#10032,#10033,#10034,#10035,
#10036,#10037,#10038,#10039,#10040,#10041,#10042,#10043,#10044,#10045,#10046,
#10047,#10048,#10049,#10050,#10051,#10052,#10053,#10054,#10055,#10056,#10057,
#10058,#10059,#10060,#10061,#10062,#10063,#10064,#10065,#10066,#10067,#10068,
#10069,#10070,#10071,#10072,#10073,#10074,#10075,#10076,#10077,#10078,#10079,
#10080,#10081,#10082,#10083,#10084,#10085,#10086,#10087,#10088,#10089,#10090,
#10091,#10092,#10093,#10094,#10095,#10096,#10097,#10098,#10099,#10100,#10101,
#10102,#10103,#10104,#10105,#10106,#10107,#10108,#10109,#10110,#10111,#10112,
#10113,#10114,#10115,#10116,#10117,#10118,#10119,#10120,#10121,#10122,#10123,
#10124,#10125,#10126,#10127,#10128,#10129,#10130,#10131,#10132,#10133,#10134,
#10135,#10136,#10137,#10138,#10139,#10140,#10141,#10142,#10143,#10144,#10145,
#10146,#10147,#10148,#10149,#10150,#10151,#10152,#10153,#10154,#10155,#10156,
#10157,#10158,#10159,#10160,#10161,#10162,#10163,#10164,#10165,#10166,#10167,
#10168,#10169,#10170,#10171,#10172,#10173,#10174,#10175,#10176,#10177,#10178,
#10179,#10180,#10181,#10182,#10183,#10184,#10185,#10186,#10187,#10188,#10189,
#10190,#10191,#10192,#10193,#10194,#10195,#10196,#10197,#10198,#10199,#10200,
#10201,#10202,#10203,#10204,#10205,#10206,#10207,#10208,#10209,#10210,#10211,
#10212,#10213,#10214,#10215,#10216,#10217,#10218,#10219),(#10220,#10221,
#10222,#10223,#10224,#10225,#10226,#10227,#10228,#10229,#10230,#10231,#10232,
#10233,#10234,#10235,#10236,#10237,#10238,#10239,#10240,#10241,#10242,#10243,
#10244,#10245,#10246,#10247,#10248,#10249,#10250,#10251,#10252,#10253,#10254,
#10255,#10256,#10257,#10258,#10259,#10260,#10261,#10262,#10263,#10264,#10265,
#10266,#10267,#10268,#10269,#10270,#10271,#10272,#10273,#10274,#10275,#10276,
#10277,#10278,#10279,#10280,#10281,#10282,#10283,#10284,#10285,#10286,#10287,
#10288,#10289,#10290,#10291,#10292,#10293,#10294,#10295,#10296,#10297,#10298,
#10299,#10300,#10301,#10302,#10303,#10304,#10305,#10306,#10307,#10308,#10309,
#10310,#10311,#10312,#10313,#10314,#10315,#10316,#10317,#10318,#10319,#10320,
#10321,#10322,#10323,#10324,#10325,#10326,#10327,#10328,#10329,#10330,#10331,
#10332,#10333,#10334,#10335,#10336,#10337,#10338,#10339,#10340,#10341,#10342,
#10343,#10344,#10345,#10346,#10347,#10348,#10349,#10350,#10351,#10352,#10353,
#10354,#10355,#10356,#10357,#10358,#10359,#10360,#10361,#10362,#10363,#10364,
#10365,#10366,#10367,#10368,#10369,#10370,#10371,#10372,#10373,#10374,#10375,
#10376,#10377,#10378,#10379,#10380,#10381,#10382,#10383,#10384,#10385,#10386,
#10387,#10388,#10389,#10390,#10391,#10392,#10393,#10394,#10395,#10396,#10397,
#10398,#10399,#10400,#10401,#10402,#10403,#10404,#10405,#10406,#10407,#10408,
#10409,#10410,#10411,#10412,#10413,#10414,#10415,#10416,#10417,#10418,#10419,
#10420,#10421,#10422,#10423,#10424,#10425,#10426,#10427,#10428,#10429,#10430,
#10431,#10432,#10433,#10434,#10435,#10436,#10437,#10438,#10439,#10440,#10441,
#10442,#10443,#10444,#10445,#10446,#10447,#10448,#10449,#10450,#10451,#10452,
#10453,#10454,#10455,#10456,#10457,#10458,#10459,#10460,#10461,#10462,#10463,
#10464,#10465,#10466,#10467,#10468,#10469,#10470,#10471,#10472,#10473,#10474,
#10475,#10476,#10477,#10478,#10479,#10480,#10481,#10482,#10483,#10484,#10485,
#10486,#10487,#10488,#10489,#10490,#10491,#10492,#10493,#10494,#10495,#10496,
#10497,#10498,#10499,#10500,#10501,#10502,#10503,#10504,#10505,#10506,#10507,
#10508,#10509,#10510,#10511,#10512,#10513,#10514,#10515,#10516,#10517,#10518,
#10519,#10520,#10521,#10522,#10523,#10524,#10525,#10526,#10527,#10528,#10529,
#10530,#10531,#10532,#10533,#10534,#10535,#10536,#10537,#10538,#10539,#10540,
#10541,#10542,#10543,#10544,#10545,#10546,#10547,#10548,#10549,#10550,#10551,
#10552,#10553,#10554,#10555,#10556,#10557,#10558,#10559,#10560,#10561,#10562,
#10563,#10564,#10565,#10566,#10567,#10568,#10569,#10570,#10571,#10572,#10573,
#10574,#10575,#10576,#10577,#10578,#10579,#10580,#10581,#10582,#10583,#10584,
#10585,#10586,#10587,#10588,#10589,#10590,#10591,#10592,#10593,#10594,#10595,
#10596,#10597,#10598,#10599,#10600,#10601,#10602,#10603,#10604,#10605,#10606,
#10607,#10608,#10609,#10610,#10611,#10612,#10613,#10614,#10615,#10616,#10617,
#10618,#10619,#10620,#10621,#10622,#10623,#10624,#10625,#10626,#10627,#10628,
#10629,#10630,#10631,#10632,#10633,#10634,#10635,#10636,#10637,#10638,#10639,
#10640,#10641,#10642,#10643,#10644,#10645,#10646,#10647,#10648,#10649,#10650,
#10651,#10652,#10653,#10654,#10655,#10656,#10657,#10658,#10659,#10660,#10661,
#10662,#10663,#10664,#10665,#10666,#10667,#10668,#10669,#10670,#10671,#10672,
#10673,#10674,#10675,#10676,#10677,#10678,#10679,#10680,#10681,#10682,#10683,
#10684,#10685,#10686,#10687,#10688,#10689,#10690,#10691,#10692,#10693,#10694,
#10695,#10696,#10697,#10698,#10699,#10700,#10701,#10702,#10703,#10704,#10705,
#10706,#10707,#10708,#10709,#10710,#10711,#10712,#10713,#10714,#10715,#10716,
#10717,#10718,#10719,#10720,#10721,#10722,#10723,#10724,#10725,#10726,#10727,
#10728,#10729,#10730,#10731,#10732,#10733,#10734,#10735,#10736,#10737,#10738,
#10739,#10740,#10741,#10742,#10743,#10744,#10745,#10746,#10747,#10748,#10749,
#10750,#10751,#10752,#10753,#10754,#10755,#10756,#10757,#10758,#10759,#10760,
#10761,#10762,#10763,#10764,#10765,#10766,#10767,#10768,#10769,#10770,#10771,
#10772,#10773,#10774,#10775,#10776,#10777,#10778,#10779,#10780,#10781,#10782,
#10783,#10784,#10785,#10786,#10787,#10788,#10789,#10790,#10791,#10792,#10793,
#10794,#10795,#10796,#10797,#10798,#10799,#10800,#10801,#10802,#10803,#10804,
#10805,#10806,#10807,#10808,#10809,#10810,#10811,#10812,#10813,#10814,#10815,
#10816,#10817,#10818,#10819,#10820,#10821,#10822,#10823,#10824,#10825,#10826,
#10827,#10828,#10829,#10830,#10831,#10832,#10833,#10834,#10835,#10836,#10837,
#10838,#10839,#10840,#10841,#10842,#10843,#10844,#10845,#10846,#10847,#10848,
#10849,#10850,#10851,#10852,#10853,#10854,#10855,#10856,#10857,#10858,#10859,
#10860,#10861,#10862,#10863,#10864,#10865,#10866,#10867,#10868,#10869,#10870,
#10871,#10872,#10873,#10874,#10875,#10876,#10877,#10878,#10879,#10880,#10881,
#10882,#10883,#10884,#10885,#10886,#10887,#10888,#10889,#10890,#10891,#10892,
#10893,#10894,#10895,#10896,#10897,#10898,#10899,#10900,#10901,#10902,#10903,
#10904,#10905,#10906,#10907,#10908,#10909,#10910,#10911,#10912,#10913,#10914,
#10915,#10916,#10917,#10918,#10919,#10920,#10921,#10922,#10923,#10924,#10925,
#10926,#10927,#10928,#10929,#10930,#10931,#10932,#10933,#10934,#10935,#10936,
#10937,#10938,#10939,#10940,#10941,#10942,#10943,#10944,#10945,#10946,#10947,
#10948,#10949,#10950,#10951,#10952,#10953,#10954,#10955,#10956,#10957,#10958,
#10959,#10960,#10961,#10962,#10963,#10964,#10965,#10966,#10967,#10968,#10969,
#10970,#10971,#10972,#10973,#10974,#10975,#10976,#10977,#10978,#10979,#10980,
#10981,#10982,#10983,#10984,#10985,#10986,#10987,#10988,#10989,#10990,#10991,
#10992,#10993,#10994,#10995,#10996,#10997,#10998,#10999,#11000,#11001,#11002,
#11003,#11004,#11005,#11006,#11007,#11008,#11009,#11010,#11011,#11012,#11013,
#11014,#11015,#11016,#11017,#11018,#11019,#11020)),.UNSPECIFIED.,.F.,.F.,
 .F.)
B_SPLINE_SURFACE_WITH_KNOTS((2,2),(3,2,2,2,2,2,2,2,2,2,2,2,2,2,2,2,2,2,
2,2,2,2,2,2,2,2,2,2,2,2,2,2,2,2,2,2,2,2,2,2,2,2,2,2,2,2,2,2,2,2,2,2,2,2,
2,2,2,2,2,2,2,2,2,2,2,2,2,2,2,2,2,2,2,2,2,2,2,2,2,2,2,2,2,2,2,2,2,2,2,2,
2,2,2,2,2,2,2,2,2,2,2,2,2,2,2,2,2,2,2,2,2,2,2,2,2,2,2,2,2,2,2,2,2,2,2,2,
2,2,2,2,2,2,2,2,2,2,2,2,2,2,2,2,2,2,2,2,2,2,2,2,2,2,2,2,2,2,2,2,2,2,2,2,
2,2,2,2,2,2,2,2,2,2,2,2,2,2,2,2,2,2,2,2,2,2,2,2,2,2,2,2,2,2,2,2,2,2,2,2,
2,2,2,2,2,2,2,2,2,2,2,2,2,2,2,2,2,2,2,2,2,2,2,2,2,2,2,2,2,2,2,2,2,2,2,2,
2,2,2,2,2,2,2,2,2,2,2,2,2,2,2,2,2,2,2,2,2,2,2,2,2,2,2,2,2,2,2,2,2,2,2,2,
2,2,2,2,2,2,2,2,2,2,2,2,2,2,2,2,2,2,2,2,2,2,2,2,2,2,2,2,2,2,2,2,2,2,2,2,
2,2,2,2,2,2,2,2,2,2,2,2,2,2,2,2,2,2,2,2,2,2,2,2,2,2,2,2,2,2,2,2,2,2,2,2,
2,2,2,2,2,2,2,2,2,2,2,2,2,2,2,2,2,2,2,2,2,2,2,2,2,2,2,2,2,2,2,2,2,2,2,2,
2,2,2,2,2,2,2,2,2,2,2,2,2,2,2,2,2,2,2,2,2,2,3),(0.,1.),(0.,0.0025,0.005,
0.0075,0.01,0.0125,0.015,0.0175,0.02,0.0225,0.025,0.0275,0.03,0.0325,0.035,
0.0375,0.04,0.0425,0.045,0.0475,0.05,0.0525,0.055,0.0575,0.06,0.0625,0.065,
0.0675,0.07,0.0725,0.075,0.0775,0.08,0.0825,0.085,0.0875,0.09,0.0925,0.095,
0.0975,0.1,0.1025,0.105,0.1075,0.11,0.1125,0.115,0.1175,0.12,0.1225,0.125,
0.1275,0.13,0.1325,0.135,0.1375,0.14,0.1425,0.145,0.1475,0.15,0.1525,0.155,
0.1575,0.16,0.1625,0.165,0.1675,0.17,0.1725,0.175,0.1775,0.18,0.1825,0.185,
0.1875,0.19,0.1925,0.195,0.1975,0.2,0.2025,0.205,0.2075,0.21,0.2125,0.215,
0.2175,0.22,0.2225,0.225,0.2275,0.23,0.2325,0.235,0.2375,0.24,0.2425,0.245,
0.2475,0.25,0.2525,0.255,0.2575,0.26,0.2625,0.265,0.2675,0.27,0.2725,0.275,
0.2775,0.28,0.2825,0.285,0.2875,0.29,0.2925,0.295,0.2975,0.3,0.3025,0.305,
0.3075,0.31,0.3125,0.315,0.3175,0.32,0.3225,0.325,0.3275,0.33,0.3325,0.335,
0.3375,0.34,0.3425,0.345,0.3475,0.35,0.3525,0.355,0.3575,0.36,0.3625,0.365,
0.3675,0.37,0.3725,0.375,0.3775,0.38,0.3825,0.385,0.3875,0.39,0.3925,0.395,
0.3975,0.4,0.4025,0.405,0.4075,0.41,0.4125,0.415,0.4175,0.42,0.4225,0.425,
0.4275,0.43,0.4325,0.435,0.4375,0.44,0.4425,0.445,0.4475,0.45,0.4525,0.455,
0.4575,0.46,0.4625,0.465,0.4675,0.47,0.4725,0.475,0.4775,0.48,0.4825,0.485,
0.4875,0.49,0.4925,0.495,0.4975,0.5,0.5025,0.505,0.5075,0.51,0.5125,0.515,
0.5175,0.52,0.5225,0.525,0.5275,0.53,0.5325,0.535,0.5375,0.54,0.5425,0.545,
0.5475,0.55,0.5525,0.555,0.5575,0.56,0.5625,0.565,0.5675,0.57,0.5725,0.575,
0.5775,0.58,0.5825,0.585,0.5875,0.59,0.5925,0.595,0.5975,0.6,0.6025,0.605,
0.6075,0.61,0.6125,0.615,0.6175,0.62,0.6225,0.625,0.6275,0.63,0.6325,0.635,
0.6375,0.64,0.6425,0.645,0.6475,0.65,0.6525,0.655,0.6575,0.66,0.6625,0.665,
0.6675,0.67,0.6725,0.675,0.6775,0.68,0.6825,0.685,0.6875,0.69,0.6925,0.695,
0.6975,0.7,0.7025,0.705,0.7075,0.71,0.7125,0.715,0.7175,0.72,0.7225,0.725,
0.7275,0.73,0.7325,0.735,0.7375,0.74,0.7425,0.745,0.7475,0.75,0.7525,0.755,
0.7575,0.76,0.7625,0.765,0.7675,0.77,0.7725,0.775,0.7775,0.78,0.7825,0.785,
0.7875,0.79,0.7925,0.795,0.7975,0.8,0.8025,0.805,0.8075,0.81,0.8125,0.815,
0.8175,0.82,0.8225,0.825,0.8275,0.83,0.8325,0.835,0.8375,0.84,0.8425,0.845,
0.8475,0.85,0.8525,0.855,0.8575,0.86,0.8625,0.865,0.8675,0.87,0.8725,0.875,
0.8775,0.88,0.8825,0.885,0.8875,0.89,0.8925,0.895,0.8975,0.9,0.9025,0.905,
0.9075,0.91,0.9125,0.915,0.9175,0.92,0.9225,0.925,0.9275,0.93,0.9325,0.935,
0.9375,0.94,0.9425,0.945,0.9475,0.95,0.9525,0.955,0.9575,0.96,0.9625,0.965,
0.9675,0.97,0.9725,0.975,0.9775,0.98,0.9825,0.985,0.9875,0.99,0.9925,0.995,
0.9975,1.),.UNSPECIFIED.)
GEOMETRIC_REPRESENTATION_ITEM()
RATIONAL_B_SPLINE_SURFACE(((1.,0.923879532511287,1.,0.923879532511287,1.,
0.923879532511287,1.,0.923879532511287,1.,0.923879532511287,1.,0.923879532511287,
1.,0.923879532511287,1.,0.923879532511287,1.,0.923879532511287,1.,0.923879532511287,
1.,0.923879532511287,1.,0.923879532511287,1.,0.923879532511287,1.,0.923879532511287,
1.,0.923879532511287,1.,0.923879532511287,1.,0.923879532511287,1.,0.923879532511287,
1.,0.923879532511287,1.,0.923879532511287,1.,0.923879532511287,1.,0.923879532511287,
1.,0.923879532511287,1.,0.923879532511287,1.,0.923879532511287,1.,0.923879532511287,
1.,0.923879532511287,1.,0.923879532511287,1.,0.923879532511287,1.,0.923879532511287,
1.,0.923879532511287,1.,0.923879532511287,1.,0.923879532511287,1.,0.923879532511287,
1.,0.923879532511287,1.,0.923879532511287,1.,0.923879532511287,1.,0.923879532511287,
1.,0.923879532511287,1.,0.923879532511287,1.,0.923879532511287,1.,0.923879532511287,
1.,0.923879532511287,1.,0.923879532511287,1.,0.923879532511287,1.,0.923879532511287,
1.,0.923879532511287,1.,0.923879532511287,1.,0.923879532511287,1.,0.923879532511287,
1.,0.923879532511287,1.,0.923879532511287,1.,0.923879532511287,1.,0.923879532511287,
1.,0.923879532511287,1.,0.923879532511287,1.,0.923879532511287,1.,0.923879532511287,
1.,0.923879532511287,1.,0.923879532511287,1.,0.923879532511287,1.,0.923879532511287,
1.,0.923879532511287,1.,0.923879532511287,1.,0.923879532511287,1.,0.923879532511287,
1.,0.923879532511287,1.,0.923879532511287,1.,0.923879532511287,1.,0.923879532511287,
1.,0.923879532511287,1.,0.923879532511287,1.,0.923879532511287,1.,0.923879532511287,
1.,0.923879532511287,1.,0.923879532511287,1.,0.923879532511287,1.,0.923879532511287,
1.,0.923879532511287,1.,0.923879532511287,1.,0.923879532511287,1.,0.923879532511287,
1.,0.923879532511287,1.,0.923879532511287,1.,0.923879532511287,1.,0.923879532511287,
1.,0.923879532511287,1.,0.923879532511287,1.,0.923879532511287,1.,0.923879532511287,
1.,0.923879532511287,1.,0.923879532511287,1.,0.923879532511287,1.,0.923879532511287,
1.,0.923879532511287,1.,0.923879532511287,1.,0.923879532511287,1.,0.923879532511287,
1.,0.923879532511287,1.,0.923879532511287,1.,0.923879532511287,1.,0.923879532511287,
1.,0.923879532511287,1.,0.923879532511287,1.,0.923879532511287,1.,0.923879532511287,
1.,0.923879532511287,1.,0.923879532511287,1.,0.923879532511287,1.,0.923879532511287,
1.,0.923879532511287,1.,0.923879532511287,1.,0.923879532511287,1.,0.923879532511287,
1.,0.923879532511287,1.,0.923879532511287,1.,0.923879532511287,1.,0.923879532511287,
1.,0.923879532511287,1.,0.923879532511287,1.,0.923879532511287,1.,0.923879532511287,
1.,0.923879532511287,1.,0.923879532511287,1.,0.923879532511287,1.,0.923879532511287,
1.,0.923879532511287,1.,0.923879532511287,1.,0.923879532511287,1.,0.923879532511287,
1.,0.923879532511287,1.,0.923879532511287,1.,0.923879532511287,1.,0.923879532511287,
1.,0.923879532511287,1.,0.923879532511287,1.,0.923879532511287,1.,0.923879532511287,
1.,0.923879532511287,1.,0.923879532511287,1.,0.923879532511287,1.,0.923879532511287,
1.,0.923879532511287,1.,0.923879532511287,1.,0.923879532511287,1.,0.923879532511287,
1.,0.923879532511287,1.,0.923879532511287,1.,0.923879532511287,1.,0.923879532511287,
1.,0.923879532511287,1.,0.923879532511287,1.,0.923879532511287,1.,0.923879532511287,
1.,0.923879532511287,1.,0.923879532511287,1.,0.923879532511287,1.,0.923879532511287,
1.,0.923879532511287,1.,0.923879532511287,1.,0.923879532511287,1.,0.923879532511287,
1.,0.923879532511287,1.,0.923879532511287,1.,0.923879532511287,1.,0.923879532511287,
1.,0.923879532511287,1.,0.923879532511287,1.,0.923879532511287,1.,0.923879532511287,
1.,0.923879532511287,1.,0.923879532511287,1.,0.923879532511287,1.,0.923879532511287,
1.,0.923879532511287,1.,0.923879532511287,1.,0.923879532511287,1.,0.923879532511287,
1.,0.923879532511287,1.,0.923879532511287,1.,0.923879532511287,1.,0.923879532511287,
1.,0.923879532511287,1.,0.923879532511287,1.,0.923879532511287,1.,0.923879532511287,
1.,0.923879532511287,1.,0.923879532511287,1.,0.923879532511287,1.,0.923879532511287,
1.,0.923879532511287,1.,0.923879532511287,1.,0.923879532511287,1.,0.923879532511287,
1.,0.923879532511287,1.,0.923879532511287,1.,0.923879532511287,1.,0.923879532511287,
1.,0.923879532511287,1.,0.923879532511287,1.,0.923879532511287,1.,0.923879532511287,
1.,0.923879532511287,1.,0.923879532511287,1.,0.923879532511287,1.,0.923879532511287,
1.,0.923879532511287,1.,0.923879532511287,1.,0.923879532511287,1.,0.923879532511287,
1.,0.923879532511287,1.,0.923879532511287,1.,0.923879532511287,1.,0.923879532511287,
1.,0.923879532511287,1.,0.923879532511287,1.,0.923879532511287,1.,0.923879532511287,
1.,0.923879532511287,1.,0.923879532511287,1.,0.923879532511287,1.,0.923879532511287,
1.,0.923879532511287,1.,0.923879532511287,1.,0.923879532511287,1.,0.923879532511287,
1.,0.923879532511287,1.,0.923879532511287,1.,0.923879532511287,1.,0.923879532511287,
1.,0.923879532511287,1.,0.923879532511287,1.,0.923879532511287,1.,0.923879532511287,
1.,0.923879532511287,1.,0.923879532511287,1.,0.923879532511287,1.,0.923879532511287,
1.,0.923879532511287,1.,0.923879532511287,1.,0.923879532511287,1.,0.923879532511287,
1.,0.923879532511287,1.,0.923879532511287,1.,0.923879532511287,1.,0.923879532511287,
1.,0.923879532511287,1.,0.923879532511287,1.,0.923879532511287,1.,0.923879532511287,
1.,0.923879532511287,1.,0.923879532511287,1.,0.923879532511287,1.,0.923879532511287,
1.,0.923879532511287,1.,0.923879532511287,1.,0.923879532511287,1.,0.923879532511287,
1.,0.923879532511287,1.,0.923879532511287,1.,0.923879532511287,1.,0.923879532511287,
1.,0.923879532511287,1.,0.923879532511287,1.,0.923879532511287,1.,0.923879532511287,
1.,0.923879532511287,1.,0.923879532511287,1.,0.923879532511287,1.,0.923879532511287,
1.,0.923879532511287,1.,0.923879532511287,1.,0.923879532511287,1.,0.923879532511287,
1.,0.923879532511287,1.,0.923879532511287,1.,0.923879532511287,1.,0.923879532511287,
1.,0.923879532511287,1.,0.923879532511287,1.,0.923879532511287,1.,0.923879532511287,
1.,0.923879532511287,1.,0.923879532511287,1.,0.923879532511287,1.,0.923879532511287,
1.,0.923879532511287,1.,0.923879532511287,1.,0.923879532511287,1.,0.923879532511287,
1.,0.923879532511287,1.,0.923879532511287,1.,0.923879532511287,1.,0.923879532511287,
1.,0.923879532511287,1.,0.923879532511287,1.,0.923879532511287,1.,0.923879532511287,
1.,0.923879532511287,1.,0.923879532511287,1.,0.923879532511287,1.,0.923879532511287,
1.,0.923879532511287,1.,0.923879532511287,1.,0.923879532511287,1.,0.923879532511287,
1.,0.923879532511287,1.,0.923879532511287,1.,0.923879532511287,1.,0.923879532511287,
1.,0.923879532511287,1.,0.923879532511287,1.,0.923879532511287,1.,0.923879532511287,
1.,0.923879532511287,1.,0.923879532511287,1.,0.923879532511287,1.,0.923879532511287,
1.,0.923879532511287,1.,0.923879532511287,1.,0.923879532511287,1.,0.923879532511287,
1.,0.923879532511287,1.,0.923879532511287,1.,0.923879532511287,1.,0.923879532511287,
1.,0.923879532511287,1.,0.923879532511287,1.,0.923879532511287,1.,0.923879532511287,
1.,0.923879532511287,1.,0.923879532511287,1.,0.923879532511287,1.,0.923879532511287,
1.,0.923879532511287,1.,0.923879532511287,1.,0.923879532511287,1.,0.923879532511287,
1.,0.923879532511287,1.,0.923879532511287,1.,0.923879532511287,1.,0.923879532511287,
1.,0.923879532511287,1.,0.923879532511287,1.,0.923879532511287,1.,0.923879532511287,
1.,0.923879532511287,1.,0.923879532511287,1.,0.923879532511287,1.,0.923879532511287,
1.,0.923879532511287,1.,0.923879532511287,1.,0.923879532511287,1.,0.923879532511287,
1.,0.923879532511287,1.,0.923879532511287,1.,0.923879532511287,1.,0.923879532511287,
1.,0.923879532511287,1.,0.923879532511287,1.,0.923879532511287,1.,0.923879532511287,
1.,0.923879532511287,1.,0.923879532511287,1.,0.923879532511287,1.,0.923879532511287,
1.,0.923879532511287,1.,0.923879532511287,1.,0.923879532511287,1.,0.923879532511287,
1.,0.923879532511287,1.,0.923879532511287,1.,0.923879532511287,1.,0.923879532511287,
1.,0.923879532511287,1.,0.923879532511287,1.,0.923879532511287,1.,0.923879532511287,
1.,0.923879532511287,1.,0.923879532511287,1.,0.923879532511287,1.,0.923879532511287,
1.,0.923879532511287,1.,0.923879532511287,1.,0.923879532511287,1.,0.923879532511287,
1.,0.923879532511287,1.,0.923879532511287,1.,0.923879532511287,1.,0.923879532511287,
1.,0.923879532511287,1.,0.923879532511287,1.,0.923879532511287,1.,0.923879532511287,
1.,0.923879532511287,1.,0.923879532511287,1.,0.923879532511287,1.,0.923879532511287,
1.,0.923879532511287,1.,0.923879532511287,1.),(1.,0.923879532511287,1.,
0.923879532511287,1.,0.923879532511287,1.,0.923879532511287,1.,0.923879532511287,
1.,0.923879532511287,1.,0.923879532511287,1.,0.923879532511287,1.,0.923879532511287,
1.,0.923879532511287,1.,0.923879532511287,1.,0.923879532511287,1.,0.923879532511287,
1.,0.923879532511287,1.,0.923879532511287,1.,0.923879532511287,1.,0.923879532511287,
1.,0.923879532511287,1.,0.923879532511287,1.,0.923879532511287,1.,0.923879532511287,
1.,0.923879532511287,1.,0.923879532511287,1.,0.923879532511287,1.,0.923879532511287,
1.,0.923879532511287,1.,0.923879532511287,1.,0.923879532511287,1.,0.923879532511287,
1.,0.923879532511287,1.,0.923879532511287,1.,0.923879532511287,1.,0.923879532511287,
1.,0.923879532511287,1.,0.923879532511287,1.,0.923879532511287,1.,0.923879532511287,
1.,0.923879532511287,1.,0.923879532511287,1.,0.923879532511287,1.,0.923879532511287,
1.,0.923879532511287,1.,0.923879532511287,1.,0.923879532511287,1.,0.923879532511287,
1.,0.923879532511287,1.,0.923879532511287,1.,0.923879532511287,1.,0.923879532511287,
1.,0.923879532511287,1.,0.923879532511287,1.,0.923879532511287,1.,0.923879532511287,
1.,0.923879532511287,1.,0.923879532511287,1.,0.923879532511287,1.,0.923879532511287,
1.,0.923879532511287,1.,0.923879532511287,1.,0.923879532511287,1.,0.923879532511287,
1.,0.923879532511287,1.,0.923879532511287,1.,0.923879532511287,1.,0.923879532511287,
1.,0.923879532511287,1.,0.923879532511287,1.,0.923879532511287,1.,0.923879532511287,
1.,0.923879532511287,1.,0.923879532511287,1.,0.923879532511287,1.,0.923879532511287,
1.,0.923879532511287,1.,0.923879532511287,1.,0.923879532511287,1.,0.923879532511287,
1.,0.923879532511287,1.,0.923879532511287,1.,0.923879532511287,1.,0.923879532511287,
1.,0.923879532511287,1.,0.923879532511287,1.,0.923879532511287,1.,0.923879532511287,
1.,0.923879532511287,1.,0.923879532511287,1.,0.923879532511287,1.,0.923879532511287,
1.,0.923879532511287,1.,0.923879532511287,1.,0.923879532511287,1.,0.923879532511287,
1.,0.923879532511287,1.,0.923879532511287,1.,0.923879532511287,1.,0.923879532511287,
1.,0.923879532511287,1.,0.923879532511287,1.,0.923879532511287,1.,0.923879532511287,
1.,0.923879532511287,1.,0.923879532511287,1.,0.923879532511287,1.,0.923879532511287,
1.,0.923879532511287,1.,0.923879532511287,1.,0.923879532511287,1.,0.923879532511287,
1.,0.923879532511287,1.,0.923879532511287,1.,0.923879532511287,1.,0.923879532511287,
1.,0.923879532511287,1.,0.923879532511287,1.,0.923879532511287,1.,0.923879532511287,
1.,0.923879532511287,1.,0.923879532511287,1.,0.923879532511287,1.,0.923879532511287,
1.,0.923879532511287,1.,0.923879532511287,1.,0.923879532511287,1.,0.923879532511287,
1.,0.923879532511287,1.,0.923879532511287,1.,0.923879532511287,1.,0.923879532511287,
1.,0.923879532511287,1.,0.923879532511287,1.,0.923879532511287,1.,0.923879532511287,
1.,0.923879532511287,1.,0.923879532511287,1.,0.923879532511287,1.,0.923879532511287,
1.,0.923879532511287,1.,0.923879532511287,1.,0.923879532511287,1.,0.923879532511287,
1.,0.923879532511287,1.,0.923879532511287,1.,0.923879532511287,1.,0.923879532511287,
1.,0.923879532511287,1.,0.923879532511287,1.,0.923879532511287,1.,0.923879532511287,
1.,0.923879532511287,1.,0.923879532511287,1.,0.923879532511287,1.,0.923879532511287,
1.,0.923879532511287,1.,0.923879532511287,1.,0.923879532511287,1.,0.923879532511287,
1.,0.923879532511287,1.,0.923879532511287,1.,0.923879532511287,1.,0.923879532511287,
1.,0.923879532511287,1.,0.923879532511287,1.,0.923879532511287,1.,0.923879532511287,
1.,0.923879532511287,1.,0.923879532511287,1.,0.923879532511287,1.,0.923879532511287,
1.,0.923879532511287,1.,0.923879532511287,1.,0.923879532511287,1.,0.923879532511287,
1.,0.923879532511287,1.,0.923879532511287,1.,0.923879532511287,1.,0.923879532511287,
1.,0.923879532511287,1.,0.923879532511287,1.,0.923879532511287,1.,0.923879532511287,
1.,0.923879532511287,1.,0.923879532511287,1.,0.923879532511287,1.,0.923879532511287,
1.,0.923879532511287,1.,0.923879532511287,1.,0.923879532511287,1.,0.923879532511287,
1.,0.923879532511287,1.,0.923879532511287,1.,0.923879532511287,1.,0.923879532511287,
1.,0.923879532511287,1.,0.923879532511287,1.,0.923879532511287,1.,0.923879532511287,
1.,0.923879532511287,1.,0.923879532511287,1.,0.923879532511287,1.,0.923879532511287,
1.,0.923879532511287,1.,0.923879532511287,1.,0.923879532511287,1.,0.923879532511287,
1.,0.923879532511287,1.,0.923879532511287,1.,0.923879532511287,1.,0.923879532511287,
1.,0.923879532511287,1.,0.923879532511287,1.,0.923879532511287,1.,0.923879532511287,
1.,0.923879532511287,1.,0.923879532511287,1.,0.923879532511287,1.,0.923879532511287,
1.,0.923879532511287,1.,0.923879532511287,1.,0.923879532511287,1.,0.923879532511287,
1.,0.923879532511287,1.,0.923879532511287,1.,0.923879532511287,1.,0.923879532511287,
1.,0.923879532511287,1.,0.923879532511287,1.,0.923879532511287,1.,0.923879532511287,
1.,0.923879532511287,1.,0.923879532511287,1.,0.923879532511287,1.,0.923879532511287,
1.,0.923879532511287,1.,0.923879532511287,1.,0.923879532511287,1.,0.923879532511287,
1.,0.923879532511287,1.,0.923879532511287,1.,0.923879532511287,1.,0.923879532511287,
1.,0.923879532511287,1.,0.923879532511287,1.,0.923879532511287,1.,0.923879532511287,
1.,0.923879532511287,1.,0.923879532511287,1.,0.923879532511287,1.,0.923879532511287,
1.,0.923879532511287,1.,0.923879532511287,1.,0.923879532511287,1.,0.923879532511287,
1.,0.923879532511287,1.,0.923879532511287,1.,0.923879532511287,1.,0.923879532511287,
1.,0.923879532511287,1.,0.923879532511287,1.,0.923879532511287,1.,0.923879532511287,
1.,0.923879532511287,1.,0.923879532511287,1.,0.923879532511287,1.,0.923879532511287,
1.,0.923879532511287,1.,0.923879532511287,1.,0.923879532511287,1.,0.923879532511287,
1.,0.923879532511287,1.,0.923879532511287,1.,0.923879532511287,1.,0.923879532511287,
1.,0.923879532511287,1.,0.923879532511287,1.,0.923879532511287,1.,0.923879532511287,
1.,0.923879532511287,1.,0.923879532511287,1.,0.923879532511287,1.,0.923879532511287,
1.,0.923879532511287,1.,0.923879532511287,1.,0.923879532511287,1.,0.923879532511287,
1.,0.923879532511287,1.,0.923879532511287,1.,0.923879532511287,1.,0.923879532511287,
1.,0.923879532511287,1.,0.923879532511287,1.,0.923879532511287,1.,0.923879532511287,
1.,0.923879532511287,1.,0.923879532511287,1.,0.923879532511287,1.,0.923879532511287,
1.,0.923879532511287,1.,0.923879532511287,1.,0.923879532511287,1.,0.923879532511287,
1.,0.923879532511287,1.,0.923879532511287,1.,0.923879532511287,1.,0.923879532511287,
1.,0.923879532511287,1.,0.923879532511287,1.,0.923879532511287,1.,0.923879532511287,
1.,0.923879532511287,1.,0.923879532511287,1.,0.923879532511287,1.,0.923879532511287,
1.,0.923879532511287,1.,0.923879532511287,1.,0.923879532511287,1.,0.923879532511287,
1.,0.923879532511287,1.,0.923879532511287,1.,0.923879532511287,1.,0.923879532511287,
1.,0.923879532511287,1.,0.923879532511287,1.,0.923879532511287,1.,0.923879532511287,
1.,0.923879532511287,1.,0.923879532511287,1.,0.923879532511287,1.,0.923879532511287,
1.,0.923879532511287,1.,0.923879532511287,1.,0.923879532511287,1.,0.923879532511287,
1.,0.923879532511287,1.,0.923879532511287,1.,0.923879532511287,1.,0.923879532511287,
1.,0.923879532511287,1.,0.923879532511287,1.,0.923879532511287,1.,0.923879532511287,
1.,0.923879532511287,1.,0.923879532511287,1.,0.923879532511287,1.,0.923879532511287,
1.,0.923879532511287,1.,0.923879532511287,1.,0.923879532511287,1.,0.923879532511287,
1.,0.923879532511287,1.,0.923879532511287,1.,0.923879532511287,1.,0.923879532511287,
1.,0.923879532511287,1.,0.923879532511287,1.,0.923879532511287,1.,0.923879532511287,
1.,0.923879532511287,1.,0.923879532511287,1.,0.923879532511287,1.,0.923879532511287,
1.,0.923879532511287,1.,0.923879532511287,1.,0.923879532511287,1.,0.923879532511287,
1.,0.923879532511287,1.,0.923879532511287,1.,0.923879532511287,1.,0.923879532511287,
1.,0.923879532511287,1.,0.923879532511287,1.,0.923879532511287,1.,0.923879532511287,
1.,0.923879532511287,1.,0.923879532511287,1.,0.923879532511287,1.,0.923879532511287,
1.,0.923879532511287,1.,0.923879532511287,1.,0.923879532511287,1.,0.923879532511287,
1.,0.923879532511287,1.,0.923879532511287,1.,0.923879532511287,1.,0.923879532511287,
1.,0.923879532511287,1.,0.923879532511287,1.,0.923879532511287,1.,0.923879532511287,
1.,0.923879532511287,1.,0.923879532511287,1.,0.923879532511287,1.,0.923879532511287,
1.,0.923879532511287,1.,0.923879532511287,1.,0.923879532511287,1.,0.923879532511287,
1.,0.923879532511287,1.,0.923879532511287,1.,0.923879532511287,1.)))
REPRESENTATION_ITEM('')
SURFACE()
);
#74=CONICAL_SURFACE('',#3154,118.168461709225,0.436332312998584);
#75=CONICAL_SURFACE('',#3165,114.797295826488,0.139626340159547);
#76=CONICAL_SURFACE('',#3166,120.5,0.523598775598293);
#80=PLANE('',#3146);
#81=PLANE('',#3149);
#82=PLANE('',#3152);
#83=PLANE('',#3155);
#84=PLANE('',#3156);
#85=PLANE('',#3161);
#86=PLANE('',#3164);
#112=FACE_BOUND('',#477,.T.);
#113=FACE_BOUND('',#478,.T.);
#114=FACE_BOUND('',#481,.T.);
#115=FACE_BOUND('',#483,.T.);
#116=FACE_BOUND('',#485,.T.);
#135=B_SPLINE_CURVE_WITH_KNOTS('',3,(#7651,#7652,#7653,#7654,#7655,#7656,
#7657,#7658,#7659,#7660,#7661,#7662,#7663,#7664,#7665,#7666,#7667,#7668),
 .UNSPECIFIED.,.F.,.F.,(4,2,2,2,2,2,2,2,4),(3.01498157723135,3.39185457770905,
3.76872757818674,4.14559997201688,4.52247236584703,4.89934475967718,5.27621715350733,
5.65309015398502,6.02996315446271),.UNSPECIFIED.);
#136=B_SPLINE_CURVE_WITH_KNOTS('',3,(#7669,#7670,#7671,#7672,#7673,#7674,
#7675,#7676,#7677,#7678,#7679,#7680,#7681,#7682,#7683,#7684,#7685,#7686),
 .UNSPECIFIED.,.F.,.F.,(4,2,2,2,2,2,2,2,4),(6.02996315446271,6.4068361549404,
6.78370915541809,7.16058154924824,7.53745394307838,7.91432633690853,8.29119873073868,
8.66807173121637,9.04494473169406),.UNSPECIFIED.);
#137=B_SPLINE_CURVE_WITH_KNOTS('',3,(#7689,#7690,#7691,#7692,#7693,#7694,
#7695,#7696,#7697,#7698,#7699,#7700,#7701,#7702,#7703,#7704,#7705,#7706),
 .UNSPECIFIED.,.F.,.F.,(4,2,2,2,2,2,2,2,4),(0.,0.376873000477691,0.753746000955381,
1.13061839478553,1.50749078861568,1.88436318244582,2.26123557627597,2.63810857675366,
3.01498157723135),.UNSPECIFIED.);
#138=B_SPLINE_CURVE_WITH_KNOTS('',3,(#7707,#7708,#7709,#7710,#7711,#7712,
#7713,#7714,#7715,#7716,#7717,#7718,#7719,#7720,#7721,#7722,#7723,#7724),
 .UNSPECIFIED.,.F.,.F.,(4,2,2,2,2,2,2,2,4),(3.01498157723135,3.39185457770904,
3.76872757818674,4.14559997201688,4.52247236584703,4.89934475967718,5.27621715350733,
5.65309015398502,6.02996315446271),.UNSPECIFIED.);
#149=CIRCLE('',#3091,105.5);
#150=CIRCLE('',#3140,105.5);
#151=CIRCLE('',#3142,120.5);
#152=CIRCLE('',#3143,120.5);
#153=CIRCLE('',#3144,120.5);
#154=CIRCLE('',#3147,118.168461709225);
#155=CIRCLE('',#3148,115.5);
#156=CIRCLE('',#3150,114.726497308104);
#157=CIRCLE('',#3151,105.5);
#158=CIRCLE('',#3153,114.797295826488);
#159=CIRCLE('',#3160,10.);
#160=CIRCLE('',#3163,10.);
#207=FACE_OUTER_BOUND('',#377,.T.);
#208=FACE_OUTER_BOUND('',#378,.T.);
#209=FACE_OUTER_BOUND('',#379,.T.);
#210=FACE_OUTER_BOUND('',#380,.T.);
#211=FACE_OUTER_BOUND('',#381,.T.);
#212=FACE_OUTER_BOUND('',#382,.T.);
#213=FACE_OUTER_BOUND('',#383,.T.);
#214=FACE_OUTER_BOUND('',#384,.T.);
#215=FACE_OUTER_BOUND('',#385,.T.);
#216=FACE_OUTER_BOUND('',#386,.T.);
#217=FACE_OUTER_BOUND('',#387,.T.);
#218=FACE_OUTER_BOUND('',#388,.T.);
#219=FACE_OUTER_BOUND('',#389,.T.);
#220=FACE_OUTER_BOUND('',#390,.T.);
#221=FACE_OUTER_BOUND('',#391,.T.);
#222=FACE_OUTER_BOUND('',#392,.T.);
#223=FACE_OUTER_BOUND('',#393,.T.);
#224=FACE_OUTER_BOUND('',#394,.T.);
#225=FACE_OUTER_BOUND('',#395,.T.);
#226=FACE_OUTER_BOUND('',#396,.T.);
#227=FACE_OUTER_BOUND('',#397,.T.);
#228=FACE_OUTER_BOUND('',#398,.T.);
#229=FACE_OUTER_BOUND('',#399,.T.);
#230=FACE_OUTER_BOUND('',#400,.T.);
#231=FACE_OUTER_BOUND('',#401,.T.);
#232=FACE_OUTER_BOUND('',#402,.T.);
#233=FACE_OUTER_BOUND('',#403,.T.);
#234=FACE_OUTER_BOUND('',#404,.T.);
#235=FACE_OUTER_BOUND('',#405,.T.);
#236=FACE_OUTER_BOUND('',#406,.T.);
#237=FACE_OUTER_BOUND('',#407,.T.);
#238=FACE_OUTER_BOUND('',#408,.T.);
#239=FACE_OUTER_BOUND('',#409,.T.);
#240=FACE_OUTER_BOUND('',#410,.T.);
#241=FACE_OUTER_BOUND('',#411,.T.);
#242=FACE_OUTER_BOUND('',#412,.T.);
#243=FACE_OUTER_BOUND('',#413,.T.);
#244=FACE_OUTER_BOUND('',#414,.T.);
#245=FACE_OUTER_BOUND('',#415,.T.);
#246=FACE_OUTER_BOUND('',#416,.T.);
#247=FACE_OUTER_BOUND('',#417,.T.);
#248=FACE_OUTER_BOUND('',#418,.T.);
#249=FACE_OUTER_BOUND('',#419,.T.);
#250=FACE_OUTER_BOUND('',#420,.T.);
#251=FACE_OUTER_BOUND('',#421,.T.);
#252=FACE_OUTER_BOUND('',#422,.T.);
#253=FACE_OUTER_BOUND('',#423,.T.);
#254=FACE_OUTER_BOUND('',#424,.T.);
#255=FACE_OUTER_BOUND('',#425,.T.);
#256=FACE_OUTER_BOUND('',#426,.T.);
#257=FACE_OUTER_BOUND('',#427,.T.);
#258=FACE_OUTER_BOUND('',#428,.T.);
#259=FACE_OUTER_BOUND('',#429,.T.);
#260=FACE_OUTER_BOUND('',#430,.T.);
#261=FACE_OUTER_BOUND('',#431,.T.);
#262=FACE_OUTER_BOUND('',#432,.T.);
#263=FACE_OUTER_BOUND('',#433,.T.);
#264=FACE_OUTER_BOUND('',#434,.T.);
#265=FACE_OUTER_BOUND('',#435,.T.);
#266=FACE_OUTER_BOUND('',#436,.T.);
#267=FACE_OUTER_BOUND('',#437,.T.);
#268=FACE_OUTER_BOUND('',#438,.T.);
#269=FACE_OUTER_BOUND('',#439,.T.);
#270=FACE_OUTER_BOUND('',#440,.T.);
#271=FACE_OUTER_BOUND('',#441,.T.);
#272=FACE_OUTER_BOUND('',#442,.T.);
#273=FACE_OUTER_BOUND('',#443,.T.);
#274=FACE_OUTER_BOUND('',#444,.T.);
#275=FACE_OUTER_BOUND('',#445,.T.);
#276=FACE_OUTER_BOUND('',#446,.T.);
#277=FACE_OUTER_BOUND('',#447,.T.);
#278=FACE_OUTER_BOUND('',#448,.T.);
#279=FACE_OUTER_BOUND('',#449,.T.);
#280=FACE_OUTER_BOUND('',#450,.T.);
#281=FACE_OUTER_BOUND('',#451,.T.);
#282=FACE_OUTER_BOUND('',#452,.T.);
#283=FACE_OUTER_BOUND('',#453,.T.);
#284=FACE_OUTER_BOUND('',#454,.T.);
#285=FACE_OUTER_BOUND('',#455,.T.);
#286=FACE_OUTER_BOUND('',#456,.T.);
#287=FACE_OUTER_BOUND('',#457,.T.);
#288=FACE_OUTER_BOUND('',#458,.T.);
#289=FACE_OUTER_BOUND('',#459,.T.);
#290=FACE_OUTER_BOUND('',#460,.T.);
#291=FACE_OUTER_BOUND('',#461,.T.);
#292=FACE_OUTER_BOUND('',#462,.T.);
#293=FACE_OUTER_BOUND('',#463,.T.);
#294=FACE_OUTER_BOUND('',#464,.T.);
#295=FACE_OUTER_BOUND('',#465,.T.);
#296=FACE_OUTER_BOUND('',#466,.T.);
#297=FACE_OUTER_BOUND('',#467,.T.);
#298=FACE_OUTER_BOUND('',#468,.T.);
#299=FACE_OUTER_BOUND('',#469,.T.);
#300=FACE_OUTER_BOUND('',#470,.T.);
#301=FACE_OUTER_BOUND('',#471,.T.);
#302=FACE_OUTER_BOUND('',#472,.T.);
#303=FACE_OUTER_BOUND('',#473,.T.);
#304=FACE_OUTER_BOUND('',#474,.T.);
#305=FACE_OUTER_BOUND('',#475,.T.);
#306=FACE_OUTER_BOUND('',#476,.T.);
#307=FACE_OUTER_BOUND('',#479,.T.);
#308=FACE_OUTER_BOUND('',#480,.T.);
#309=FACE_OUTER_BOUND('',#482,.T.);
#310=FACE_OUTER_BOUND('',#484,.T.);
#311=FACE_OUTER_BOUND('',#486,.T.);
#312=FACE_OUTER_BOUND('',#487,.T.);
#313=FACE_OUTER_BOUND('',#488,.T.);
#314=FACE_OUTER_BOUND('',#489,.T.);
#315=FACE_OUTER_BOUND('',#490,.T.);
#316=FACE_OUTER_BOUND('',#491,.T.);
#317=FACE_OUTER_BOUND('',#492,.T.);
#318=FACE_OUTER_BOUND('',#493,.T.);
#319=FACE_OUTER_BOUND('',#494,.T.);
#320=FACE_OUTER_BOUND('',#495,.T.);
#321=FACE_OUTER_BOUND('',#496,.T.);
#322=FACE_OUTER_BOUND('',#497,.T.);
#323=FACE_OUTER_BOUND('',#498,.T.);
#377=EDGE_LOOP('',(#1803,#1804,#1805,#1806));
#378=EDGE_LOOP('',(#1807,#1808,#1809,#1810));
#379=EDGE_LOOP('',(#1811,#1812,#1813,#1814));
#380=EDGE_LOOP('',(#1815,#1816,#1817,#1818));
#381=EDGE_LOOP('',(#1819,#1820,#1821,#1822));
#382=EDGE_LOOP('',(#1823,#1824,#1825,#1826));
#383=EDGE_LOOP('',(#1827,#1828,#1829,#1830));
#384=EDGE_LOOP('',(#1831,#1832,#1833,#1834));
#385=EDGE_LOOP('',(#1835,#1836,#1837,#1838));
#386=EDGE_LOOP('',(#1839,#1840,#1841,#1842));
#387=EDGE_LOOP('',(#1843,#1844,#1845,#1846));
#388=EDGE_LOOP('',(#1847,#1848,#1849,#1850));
#389=EDGE_LOOP('',(#1851,#1852,#1853,#1854));
#390=EDGE_LOOP('',(#1855,#1856,#1857,#1858));
#391=EDGE_LOOP('',(#1859,#1860,#1861,#1862));
#392=EDGE_LOOP('',(#1863,#1864,#1865,#1866));
#393=EDGE_LOOP('',(#1867,#1868,#1869,#1870));
#394=EDGE_LOOP('',(#1871,#1872,#1873,#1874));
#395=EDGE_LOOP('',(#1875,#1876,#1877,#1878));
#396=EDGE_LOOP('',(#1879,#1880,#1881,#1882));
#397=EDGE_LOOP('',(#1883,#1884,#1885,#1886));
#398=EDGE_LOOP('',(#1887,#1888,#1889,#1890));
#399=EDGE_LOOP('',(#1891,#1892,#1893,#1894));
#400=EDGE_LOOP('',(#1895,#1896,#1897,#1898));
#401=EDGE_LOOP('',(#1899,#1900,#1901,#1902));
#402=EDGE_LOOP('',(#1903,#1904,#1905,#1906));
#403=EDGE_LOOP('',(#1907,#1908,#1909,#1910));
#404=EDGE_LOOP('',(#1911,#1912,#1913,#1914));
#405=EDGE_LOOP('',(#1915,#1916,#1917,#1918));
#406=EDGE_LOOP('',(#1919,#1920,#1921,#1922));
#407=EDGE_LOOP('',(#1923,#1924,#1925,#1926));
#408=EDGE_LOOP('',(#1927,#1928,#1929,#1930));
#409=EDGE_LOOP('',(#1931,#1932,#1933,#1934));
#410=EDGE_LOOP('',(#1935,#1936,#1937,#1938));
#411=EDGE_LOOP('',(#1939,#1940,#1941,#1942));
#412=EDGE_LOOP('',(#1943,#1944,#1945,#1946));
#413=EDGE_LOOP('',(#1947,#1948,#1949,#1950));
#414=EDGE_LOOP('',(#1951,#1952,#1953,#1954));
#415=EDGE_LOOP('',(#1955,#1956,#1957,#1958));
#416=EDGE_LOOP('',(#1959,#1960,#1961,#1962));
#417=EDGE_LOOP('',(#1963,#1964,#1965,#1966));
#418=EDGE_LOOP('',(#1967,#1968,#1969,#1970));
#419=EDGE_LOOP('',(#1971,#1972,#1973,#1974));
#420=EDGE_LOOP('',(#1975,#1976,#1977,#1978));
#421=EDGE_LOOP('',(#1979,#1980,#1981,#1982));
#422=EDGE_LOOP('',(#1983,#1984,#1985,#1986));
#423=EDGE_LOOP('',(#1987,#1988,#1989,#1990));
#424=EDGE_LOOP('',(#1991,#1992,#1993,#1994));
#425=EDGE_LOOP('',(#1995,#1996,#1997,#1998));
#426=EDGE_LOOP('',(#1999,#2000,#2001,#2002));
#427=EDGE_LOOP('',(#2003,#2004,#2005,#2006));
#428=EDGE_LOOP('',(#2007,#2008,#2009,#2010));
#429=EDGE_LOOP('',(#2011,#2012,#2013,#2014));
#430=EDGE_LOOP('',(#2015,#2016,#2017,#2018));
#431=EDGE_LOOP('',(#2019,#2020,#2021,#2022));
#432=EDGE_LOOP('',(#2023,#2024,#2025,#2026));
#433=EDGE_LOOP('',(#2027,#2028,#2029,#2030));
#434=EDGE_LOOP('',(#2031,#2032,#2033,#2034));
#435=EDGE_LOOP('',(#2035,#2036,#2037,#2038));
#436=EDGE_LOOP('',(#2039,#2040,#2041,#2042));
#437=EDGE_LOOP('',(#2043,#2044,#2045,#2046));
#438=EDGE_LOOP('',(#2047,#2048,#2049,#2050));
#439=EDGE_LOOP('',(#2051,#2052,#2053,#2054));
#440=EDGE_LOOP('',(#2055,#2056,#2057,#2058));
#441=EDGE_LOOP('',(#2059,#2060,#2061,#2062));
#442=EDGE_LOOP('',(#2063,#2064,#2065,#2066));
#443=EDGE_LOOP('',(#2067,#2068,#2069,#2070));
#444=EDGE_LOOP('',(#2071,#2072,#2073,#2074));
#445=EDGE_LOOP('',(#2075,#2076,#2077,#2078));
#446=EDGE_LOOP('',(#2079,#2080,#2081,#2082));
#447=EDGE_LOOP('',(#2083,#2084,#2085,#2086));
#448=EDGE_LOOP('',(#2087,#2088,#2089,#2090));
#449=EDGE_LOOP('',(#2091,#2092,#2093,#2094));
#450=EDGE_LOOP('',(#2095,#2096,#2097,#2098));
#451=EDGE_LOOP('',(#2099,#2100,#2101,#2102));
#452=EDGE_LOOP('',(#2103,#2104,#2105,#2106));
#453=EDGE_LOOP('',(#2107,#2108,#2109,#2110));
#454=EDGE_LOOP('',(#2111,#2112,#2113,#2114));
#455=EDGE_LOOP('',(#2115,#2116,#2117,#2118));
#456=EDGE_LOOP('',(#2119,#2120,#2121,#2122));
#457=EDGE_LOOP('',(#2123,#2124,#2125,#2126));
#458=EDGE_LOOP('',(#2127,#2128,#2129,#2130));
#459=EDGE_LOOP('',(#2131,#2132,#2133,#2134));
#460=EDGE_LOOP('',(#2135,#2136,#2137,#2138));
#461=EDGE_LOOP('',(#2139,#2140,#2141,#2142));
#462=EDGE_LOOP('',(#2143,#2144,#2145,#2146));
#463=EDGE_LOOP('',(#2147,#2148,#2149,#2150));
#464=EDGE_LOOP('',(#2151,#2152,#2153,#2154));
#465=EDGE_LOOP('',(#2155,#2156,#2157,#2158));
#466=EDGE_LOOP('',(#2159,#2160,#2161,#2162));
#467=EDGE_LOOP('',(#2163,#2164,#2165,#2166));
#468=EDGE_LOOP('',(#2167,#2168,#2169,#2170));
#469=EDGE_LOOP('',(#2171,#2172,#2173,#2174));
#470=EDGE_LOOP('',(#2175,#2176,#2177,#2178));
#471=EDGE_LOOP('',(#2179,#2180,#2181,#2182));
#472=EDGE_LOOP('',(#2183,#2184,#2185,#2186));
#473=EDGE_LOOP('',(#2187,#2188,#2189,#2190));
#474=EDGE_LOOP('',(#2191,#2192,#2193,#2194));
#475=EDGE_LOOP('',(#2195,#2196,#2197,#2198,#2199,#2200,#2201,#2202));
#476=EDGE_LOOP('',(#2203,#2204,#2205,#2206,#2207));
#477=EDGE_LOOP('',(#2208,#2209));
#478=EDGE_LOOP('',(#2210,#2211));
#479=EDGE_LOOP('',(#2212,#2213,#2214,#2215));
#480=EDGE_LOOP('',(#2216));
#481=EDGE_LOOP('',(#2217));
#482=EDGE_LOOP('',(#2218));
#483=EDGE_LOOP('',(#2219,#2220));
#484=EDGE_LOOP('',(#2221));
#485=EDGE_LOOP('',(#2222));
#486=EDGE_LOOP('',(#2223,#2224,#2225,#2226));
#487=EDGE_LOOP('',(#2227,#2228,#2229,#2230));
#488=EDGE_LOOP('',(#2231,#2232,#2233,#2234));
#489=EDGE_LOOP('',(#2235,#2236,#2237,#2238,#2239,#2240,#2241,#2242,#2243,
#2244,#2245,#2246,#2247,#2248,#2249,#2250,#2251,#2252,#2253,#2254,#2255,
#2256,#2257,#2258,#2259,#2260,#2261,#2262,#2263,#2264,#2265,#2266,#2267,
#2268,#2269,#2270,#2271,#2272,#2273,#2274,#2275,#2276,#2277,#2278,#2279,
#2280,#2281,#2282,#2283,#2284,#2285,#2286,#2287,#2288,#2289,#2290,#2291,
#2292,#2293,#2294,#2295,#2296,#2297,#2298,#2299,#2300,#2301,#2302,#2303,
#2304,#2305,#2306,#2307,#2308,#2309,#2310,#2311,#2312,#2313,#2314,#2315,
#2316,#2317,#2318,#2319,#2320,#2321,#2322,#2323,#2324,#2325,#2326,#2327,
#2328,#2329,#2330,#2331,#2332,#2333,#2334,#2335,#2336,#2337,#2338));
#490=EDGE_LOOP('',(#2339,#2340,#2341,#2342));
#491=EDGE_LOOP('',(#2343,#2344,#2345,#2346,#2347,#2348,#2349,#2350,#2351,
#2352,#2353,#2354,#2355,#2356,#2357,#2358,#2359,#2360,#2361,#2362,#2363,
#2364,#2365,#2366,#2367,#2368,#2369,#2370,#2371,#2372,#2373,#2374,#2375,
#2376,#2377,#2378,#2379,#2380,#2381,#2382,#2383,#2384,#2385,#2386,#2387,
#2388,#2389,#2390,#2391,#2392,#2393,#2394,#2395,#2396,#2397,#2398,#2399,
#2400,#2401,#2402,#2403,#2404,#2405,#2406,#2407,#2408,#2409,#2410,#2411,
#2412,#2413,#2414,#2415,#2416,#2417,#2418,#2419,#2420,#2421,#2422,#2423,
#2424,#2425,#2426,#2427,#2428,#2429,#2430,#2431,#2432,#2433,#2434,#2435,
#2436,#2437,#2438,#2439,#2440,#2441,#2442,#2443,#2444,#2445,#2446));
#492=EDGE_LOOP('',(#2447,#2448,#2449));
#493=EDGE_LOOP('',(#2450,#2451,#2452,#2453,#2454));
#494=EDGE_LOOP('',(#2455));
#495=EDGE_LOOP('',(#2456,#2457,#2458,#2459,#2460));
#496=EDGE_LOOP('',(#2461));
#497=EDGE_LOOP('',(#2462,#2463,#2464,#2465));
#498=EDGE_LOOP('',(#2466,#2467,#2468,#2469,#2470));
#570=(
BOUNDED_CURVE()
B_SPLINE_CURVE(2,(#3913,#3914,#3915,#3916,#3917,#3918,#3919,#3920,#3921),
 .UNSPECIFIED.,.F.,.F.)
B_SPLINE_CURVE_WITH_KNOTS((3,2,2,2,3),(0.99,0.9925,0.995,0.9975,1.),
 .UNSPECIFIED.)
CURVE()
GEOMETRIC_REPRESENTATION_ITEM()
RATIONAL_B_SPLINE_CURVE((1.,0.923879532511287,1.,0.923879532511287,1.,0.923879532511287,
1.,0.923879532511287,1.))
REPRESENTATION_ITEM('')
);
#571=(
BOUNDED_CURVE()
B_SPLINE_CURVE(2,(#3924,#3925,#3926,#3927,#3928,#3929,#3930,#3931,#3932),
 .UNSPECIFIED.,.F.,.F.)
B_SPLINE_CURVE_WITH_KNOTS((3,2,2,2,3),(0.99,0.9925,0.995,0.9975,1.),
 .UNSPECIFIED.)
CURVE()
GEOMETRIC_REPRESENTATION_ITEM()
RATIONAL_B_SPLINE_CURVE((1.,0.923879532511287,1.,0.923879532511287,1.,0.923879532511287,
1.,0.923879532511287,1.))
REPRESENTATION_ITEM('')
);
#572=(
BOUNDED_CURVE()
B_SPLINE_CURVE(2,(#3937,#3938,#3939,#3940,#3941,#3942,#3943,#3944,#3945,
#3946,#3947,#3948,#3949,#3950,#3951,#3952,#3953),.UNSPECIFIED.,.F.,.F.)
B_SPLINE_CURVE_WITH_KNOTS((3,2,2,2,2,2,2,2,3),(0.97,0.9725,0.975,0.9775,
0.98,0.9825,0.985,0.9875,0.99),.UNSPECIFIED.)
CURVE()
GEOMETRIC_REPRESENTATION_ITEM()
RATIONAL_B_SPLINE_CURVE((1.,0.923879532511287,1.,0.923879532511287,1.,0.923879532511287,
1.,0.923879532511287,1.,0.923879532511287,1.,0.923879532511287,1.,0.923879532511287,
1.,0.923879532511287,1.))
REPRESENTATION_ITEM('')
);
#573=(
BOUNDED_CURVE()
B_SPLINE_CURVE(2,(#3954,#3955,#3956,#3957,#3958,#3959,#3960,#3961,#3962,
#3963,#3964,#3965,#3966,#3967,#3968,#3969,#3970),.UNSPECIFIED.,.F.,.F.)
B_SPLINE_CURVE_WITH_KNOTS((3,2,2,2,2,2,2,2,3),(0.97,0.9725,0.975,0.9775,
0.98,0.9825,0.985,0.9875,0.99),.UNSPECIFIED.)
CURVE()
GEOMETRIC_REPRESENTATION_ITEM()
RATIONAL_B_SPLINE_CURVE((1.,0.923879532511287,1.,0.923879532511287,1.,0.923879532511287,
1.,0.923879532511287,1.,0.923879532511287,1.,0.923879532511287,1.,0.923879532511287,
1.,0.923879532511287,1.))
REPRESENTATION_ITEM('')
);
#574=(
BOUNDED_CURVE()
B_SPLINE_CURVE(2,(#3975,#3976,#3977,#3978,#3979,#3980,#3981,#3982,#3983,
#3984,#3985,#3986,#3987,#3988,#3989,#3990,#3991),.UNSPECIFIED.,.F.,.F.)
B_SPLINE_CURVE_WITH_KNOTS((3,2,2,2,2,2,2,2,3),(0.95,0.9525,0.955,0.9575,
0.96,0.9625,0.965,0.9675,0.97),.UNSPECIFIED.)
CURVE()
GEOMETRIC_REPRESENTATION_ITEM()
RATIONAL_B_SPLINE_CURVE((1.,0.923879532511287,1.,0.923879532511287,1.,0.923879532511287,
1.,0.923879532511287,1.,0.923879532511287,1.,0.923879532511287,1.,0.923879532511287,
1.,0.923879532511287,1.))
REPRESENTATION_ITEM('')
);
#575=(
BOUNDED_CURVE()
B_SPLINE_CURVE(2,(#3992,#3993,#3994,#3995,#3996,#3997,#3998,#3999,#4000,
#4001,#4002,#4003,#4004,#4005,#4006,#4007,#4008),.UNSPECIFIED.,.F.,.F.)
B_SPLINE_CURVE_WITH_KNOTS((3,2,2,2,2,2,2,2,3),(0.95,0.9525,0.955,0.9575,
0.96,0.9625,0.965,0.9675,0.97),.UNSPECIFIED.)
CURVE()
GEOMETRIC_REPRESENTATION_ITEM()
RATIONAL_B_SPLINE_CURVE((1.,0.923879532511287,1.,0.923879532511287,1.,0.923879532511287,
1.,0.923879532511287,1.,0.923879532511287,1.,0.923879532511287,1.,0.923879532511287,
1.,0.923879532511287,1.))
REPRESENTATION_ITEM('')
);
#576=(
BOUNDED_CURVE()
B_SPLINE_CURVE(2,(#4013,#4014,#4015,#4016,#4017,#4018,#4019,#4020,#4021,
#4022,#4023,#4024,#4025,#4026,#4027,#4028,#4029),.UNSPECIFIED.,.F.,.F.)
B_SPLINE_CURVE_WITH_KNOTS((3,2,2,2,2,2,2,2,3),(0.93,0.9325,0.935,0.9375,
0.94,0.9425,0.945,0.9475,0.95),.UNSPECIFIED.)
CURVE()
GEOMETRIC_REPRESENTATION_ITEM()
RATIONAL_B_SPLINE_CURVE((1.,0.923879532511287,1.,0.923879532511287,1.,0.923879532511287,
1.,0.923879532511287,1.,0.923879532511287,1.,0.923879532511287,1.,0.923879532511287,
1.,0.923879532511287,1.))
REPRESENTATION_ITEM('')
);
#577=(
BOUNDED_CURVE()
B_SPLINE_CURVE(2,(#4030,#4031,#4032,#4033,#4034,#4035,#4036,#4037,#4038,
#4039,#4040,#4041,#4042,#4043,#4044,#4045,#4046),.UNSPECIFIED.,.F.,.F.)
B_SPLINE_CURVE_WITH_KNOTS((3,2,2,2,2,2,2,2,3),(0.93,0.9325,0.935,0.9375,
0.94,0.9425,0.945,0.9475,0.95),.UNSPECIFIED.)
CURVE()
GEOMETRIC_REPRESENTATION_ITEM()
RATIONAL_B_SPLINE_CURVE((1.,0.923879532511287,1.,0.923879532511287,1.,0.923879532511287,
1.,0.923879532511287,1.,0.923879532511287,1.,0.923879532511287,1.,0.923879532511287,
1.,0.923879532511287,1.))
REPRESENTATION_ITEM('')
);
#578=(
BOUNDED_CURVE()
B_SPLINE_CURVE(2,(#4051,#4052,#4053,#4054,#4055,#4056,#4057,#4058,#4059,
#4060,#4061,#4062,#4063,#4064,#4065,#4066,#4067),.UNSPECIFIED.,.F.,.F.)
B_SPLINE_CURVE_WITH_KNOTS((3,2,2,2,2,2,2,2,3),(0.91,0.9125,0.915,0.9175,
0.92,0.9225,0.925,0.9275,0.93),.UNSPECIFIED.)
CURVE()
GEOMETRIC_REPRESENTATION_ITEM()
RATIONAL_B_SPLINE_CURVE((1.,0.923879532511287,1.,0.923879532511287,1.,0.923879532511287,
1.,0.923879532511287,1.,0.923879532511287,1.,0.923879532511287,1.,0.923879532511287,
1.,0.923879532511287,1.))
REPRESENTATION_ITEM('')
);
#579=(
BOUNDED_CURVE()
B_SPLINE_CURVE(2,(#4068,#4069,#4070,#4071,#4072,#4073,#4074,#4075,#4076,
#4077,#4078,#4079,#4080,#4081,#4082,#4083,#4084),.UNSPECIFIED.,.F.,.F.)
B_SPLINE_CURVE_WITH_KNOTS((3,2,2,2,2,2,2,2,3),(0.91,0.9125,0.915,0.9175,
0.92,0.9225,0.925,0.9275,0.93),.UNSPECIFIED.)
CURVE()
GEOMETRIC_REPRESENTATION_ITEM()
RATIONAL_B_SPLINE_CURVE((1.,0.923879532511287,1.,0.923879532511287,1.,0.923879532511287,
1.,0.923879532511287,1.,0.923879532511287,1.,0.923879532511287,1.,0.923879532511287,
1.,0.923879532511287,1.))
REPRESENTATION_ITEM('')
);
#580=(
BOUNDED_CURVE()
B_SPLINE_CURVE(2,(#4089,#4090,#4091,#4092,#4093,#4094,#4095,#4096,#4097,
#4098,#4099,#4100,#4101,#4102,#4103,#4104,#4105),.UNSPECIFIED.,.F.,.F.)
B_SPLINE_CURVE_WITH_KNOTS((3,2,2,2,2,2,2,2,3),(0.89,0.8925,0.895,0.8975,
0.9,0.9025,0.905,0.9075,0.91),.UNSPECIFIED.)
CURVE()
GEOMETRIC_REPRESENTATION_ITEM()
RATIONAL_B_SPLINE_CURVE((1.,0.923879532511287,1.,0.923879532511287,1.,0.923879532511287,
1.,0.923879532511287,1.,0.923879532511287,1.,0.923879532511287,1.,0.923879532511287,
1.,0.923879532511287,1.))
REPRESENTATION_ITEM('')
);
#581=(
BOUNDED_CURVE()
B_SPLINE_CURVE(2,(#4106,#4107,#4108,#4109,#4110,#4111,#4112,#4113,#4114,
#4115,#4116,#4117,#4118,#4119,#4120,#4121,#4122),.UNSPECIFIED.,.F.,.F.)
B_SPLINE_CURVE_WITH_KNOTS((3,2,2,2,2,2,2,2,3),(0.89,0.8925,0.895,0.8975,
0.9,0.9025,0.905,0.9075,0.91),.UNSPECIFIED.)
CURVE()
GEOMETRIC_REPRESENTATION_ITEM()
RATIONAL_B_SPLINE_CURVE((1.,0.923879532511287,1.,0.923879532511287,1.,0.923879532511287,
1.,0.923879532511287,1.,0.923879532511287,1.,0.923879532511287,1.,0.923879532511287,
1.,0.923879532511287,1.))
REPRESENTATION_ITEM('')
);
#582=(
BOUNDED_CURVE()
B_SPLINE_CURVE(2,(#4127,#4128,#4129,#4130,#4131,#4132,#4133,#4134,#4135,
#4136,#4137,#4138,#4139,#4140,#4141,#4142,#4143),.UNSPECIFIED.,.F.,.F.)
B_SPLINE_CURVE_WITH_KNOTS((3,2,2,2,2,2,2,2,3),(0.87,0.8725,0.875,0.8775,
0.88,0.8825,0.885,0.8875,0.89),.UNSPECIFIED.)
CURVE()
GEOMETRIC_REPRESENTATION_ITEM()
RATIONAL_B_SPLINE_CURVE((1.,0.923879532511287,1.,0.923879532511287,1.,0.923879532511287,
1.,0.923879532511287,1.,0.923879532511287,1.,0.923879532511287,1.,0.923879532511287,
1.,0.923879532511287,1.))
REPRESENTATION_ITEM('')
);
#583=(
BOUNDED_CURVE()
B_SPLINE_CURVE(2,(#4144,#4145,#4146,#4147,#4148,#4149,#4150,#4151,#4152,
#4153,#4154,#4155,#4156,#4157,#4158,#4159,#4160),.UNSPECIFIED.,.F.,.F.)
B_SPLINE_CURVE_WITH_KNOTS((3,2,2,2,2,2,2,2,3),(0.87,0.8725,0.875,0.8775,
0.88,0.8825,0.885,0.8875,0.89),.UNSPECIFIED.)
CURVE()
GEOMETRIC_REPRESENTATION_ITEM()
RATIONAL_B_SPLINE_CURVE((1.,0.923879532511287,1.,0.923879532511287,1.,0.923879532511287,
1.,0.923879532511287,1.,0.923879532511287,1.,0.923879532511287,1.,0.923879532511287,
1.,0.923879532511287,1.))
REPRESENTATION_ITEM('')
);
#584=(
BOUNDED_CURVE()
B_SPLINE_CURVE(2,(#4165,#4166,#4167,#4168,#4169,#4170,#4171,#4172,#4173,
#4174,#4175,#4176,#4177,#4178,#4179,#4180,#4181),.UNSPECIFIED.,.F.,.F.)
B_SPLINE_CURVE_WITH_KNOTS((3,2,2,2,2,2,2,2,3),(0.85,0.8525,0.855,0.8575,
0.86,0.8625,0.865,0.8675,0.87),.UNSPECIFIED.)
CURVE()
GEOMETRIC_REPRESENTATION_ITEM()
RATIONAL_B_SPLINE_CURVE((1.,0.923879532511287,1.,0.923879532511287,1.,0.923879532511287,
1.,0.923879532511287,1.,0.923879532511287,1.,0.923879532511287,1.,0.923879532511287,
1.,0.923879532511287,1.))
REPRESENTATION_ITEM('')
);
#585=(
BOUNDED_CURVE()
B_SPLINE_CURVE(2,(#4182,#4183,#4184,#4185,#4186,#4187,#4188,#4189,#4190,
#4191,#4192,#4193,#4194,#4195,#4196,#4197,#4198),.UNSPECIFIED.,.F.,.F.)
B_SPLINE_CURVE_WITH_KNOTS((3,2,2,2,2,2,2,2,3),(0.85,0.8525,0.855,0.8575,
0.86,0.8625,0.865,0.8675,0.87),.UNSPECIFIED.)
CURVE()
GEOMETRIC_REPRESENTATION_ITEM()
RATIONAL_B_SPLINE_CURVE((1.,0.923879532511287,1.,0.923879532511287,1.,0.923879532511287,
1.,0.923879532511287,1.,0.923879532511287,1.,0.923879532511287,1.,0.923879532511287,
1.,0.923879532511287,1.))
REPRESENTATION_ITEM('')
);
#586=(
BOUNDED_CURVE()
B_SPLINE_CURVE(2,(#4203,#4204,#4205,#4206,#4207,#4208,#4209,#4210,#4211,
#4212,#4213,#4214,#4215,#4216,#4217,#4218,#4219),.UNSPECIFIED.,.F.,.F.)
B_SPLINE_CURVE_WITH_KNOTS((3,2,2,2,2,2,2,2,3),(0.83,0.8325,0.835,0.8375,
0.84,0.8425,0.845,0.8475,0.85),.UNSPECIFIED.)
CURVE()
GEOMETRIC_REPRESENTATION_ITEM()
RATIONAL_B_SPLINE_CURVE((1.,0.923879532511287,1.,0.923879532511287,1.,0.923879532511287,
1.,0.923879532511287,1.,0.923879532511287,1.,0.923879532511287,1.,0.923879532511287,
1.,0.923879532511287,1.))
REPRESENTATION_ITEM('')
);
#587=(
BOUNDED_CURVE()
B_SPLINE_CURVE(2,(#4220,#4221,#4222,#4223,#4224,#4225,#4226,#4227,#4228,
#4229,#4230,#4231,#4232,#4233,#4234,#4235,#4236),.UNSPECIFIED.,.F.,.F.)
B_SPLINE_CURVE_WITH_KNOTS((3,2,2,2,2,2,2,2,3),(0.83,0.8325,0.835,0.8375,
0.84,0.8425,0.845,0.8475,0.85),.UNSPECIFIED.)
CURVE()
GEOMETRIC_REPRESENTATION_ITEM()
RATIONAL_B_SPLINE_CURVE((1.,0.923879532511287,1.,0.923879532511287,1.,0.923879532511287,
1.,0.923879532511287,1.,0.923879532511287,1.,0.923879532511287,1.,0.923879532511287,
1.,0.923879532511287,1.))
REPRESENTATION_ITEM('')
);
#588=(
BOUNDED_CURVE()
B_SPLINE_CURVE(2,(#4241,#4242,#4243,#4244,#4245,#4246,#4247,#4248,#4249,
#4250,#4251,#4252,#4253,#4254,#4255,#4256,#4257),.UNSPECIFIED.,.F.,.F.)
B_SPLINE_CURVE_WITH_KNOTS((3,2,2,2,2,2,2,2,3),(0.81,0.8125,0.815,0.8175,
0.82,0.8225,0.825,0.8275,0.83),.UNSPECIFIED.)
CURVE()
GEOMETRIC_REPRESENTATION_ITEM()
RATIONAL_B_SPLINE_CURVE((1.,0.923879532511287,1.,0.923879532511287,1.,0.923879532511287,
1.,0.923879532511287,1.,0.923879532511287,1.,0.923879532511287,1.,0.923879532511287,
1.,0.923879532511287,1.))
REPRESENTATION_ITEM('')
);
#589=(
BOUNDED_CURVE()
B_SPLINE_CURVE(2,(#4258,#4259,#4260,#4261,#4262,#4263,#4264,#4265,#4266,
#4267,#4268,#4269,#4270,#4271,#4272,#4273,#4274),.UNSPECIFIED.,.F.,.F.)
B_SPLINE_CURVE_WITH_KNOTS((3,2,2,2,2,2,2,2,3),(0.81,0.8125,0.815,0.8175,
0.82,0.8225,0.825,0.8275,0.83),.UNSPECIFIED.)
CURVE()
GEOMETRIC_REPRESENTATION_ITEM()
RATIONAL_B_SPLINE_CURVE((1.,0.923879532511287,1.,0.923879532511287,1.,0.923879532511287,
1.,0.923879532511287,1.,0.923879532511287,1.,0.923879532511287,1.,0.923879532511287,
1.,0.923879532511287,1.))
REPRESENTATION_ITEM('')
);
#590=(
BOUNDED_CURVE()
B_SPLINE_CURVE(2,(#4279,#4280,#4281,#4282,#4283,#4284,#4285,#4286,#4287,
#4288,#4289,#4290,#4291,#4292,#4293,#4294,#4295),.UNSPECIFIED.,.F.,.F.)
B_SPLINE_CURVE_WITH_KNOTS((3,2,2,2,2,2,2,2,3),(0.79,0.7925,0.795,0.7975,
0.8,0.8025,0.805,0.8075,0.81),.UNSPECIFIED.)
CURVE()
GEOMETRIC_REPRESENTATION_ITEM()
RATIONAL_B_SPLINE_CURVE((1.,0.923879532511287,1.,0.923879532511287,1.,0.923879532511287,
1.,0.923879532511287,1.,0.923879532511287,1.,0.923879532511287,1.,0.923879532511287,
1.,0.923879532511287,1.))
REPRESENTATION_ITEM('')
);
#591=(
BOUNDED_CURVE()
B_SPLINE_CURVE(2,(#4296,#4297,#4298,#4299,#4300,#4301,#4302,#4303,#4304,
#4305,#4306,#4307,#4308,#4309,#4310,#4311,#4312),.UNSPECIFIED.,.F.,.F.)
B_SPLINE_CURVE_WITH_KNOTS((3,2,2,2,2,2,2,2,3),(0.79,0.7925,0.795,0.7975,
0.8,0.8025,0.805,0.8075,0.81),.UNSPECIFIED.)
CURVE()
GEOMETRIC_REPRESENTATION_ITEM()
RATIONAL_B_SPLINE_CURVE((1.,0.923879532511287,1.,0.923879532511287,1.,0.923879532511287,
1.,0.923879532511287,1.,0.923879532511287,1.,0.923879532511287,1.,0.923879532511287,
1.,0.923879532511287,1.))
REPRESENTATION_ITEM('')
);
#592=(
BOUNDED_CURVE()
B_SPLINE_CURVE(2,(#4317,#4318,#4319,#4320,#4321,#4322,#4323,#4324,#4325,
#4326,#4327,#4328,#4329,#4330,#4331,#4332,#4333),.UNSPECIFIED.,.F.,.F.)
B_SPLINE_CURVE_WITH_KNOTS((3,2,2,2,2,2,2,2,3),(0.77,0.7725,0.775,0.7775,
0.78,0.7825,0.785,0.7875,0.79),.UNSPECIFIED.)
CURVE()
GEOMETRIC_REPRESENTATION_ITEM()
RATIONAL_B_SPLINE_CURVE((1.,0.923879532511287,1.,0.923879532511287,1.,0.923879532511287,
1.,0.923879532511287,1.,0.923879532511287,1.,0.923879532511287,1.,0.923879532511287,
1.,0.923879532511287,1.))
REPRESENTATION_ITEM('')
);
#593=(
BOUNDED_CURVE()
B_SPLINE_CURVE(2,(#4334,#4335,#4336,#4337,#4338,#4339,#4340,#4341,#4342,
#4343,#4344,#4345,#4346,#4347,#4348,#4349,#4350),.UNSPECIFIED.,.F.,.F.)
B_SPLINE_CURVE_WITH_KNOTS((3,2,2,2,2,2,2,2,3),(0.77,0.7725,0.775,0.7775,
0.78,0.7825,0.785,0.7875,0.79),.UNSPECIFIED.)
CURVE()
GEOMETRIC_REPRESENTATION_ITEM()
RATIONAL_B_SPLINE_CURVE((1.,0.923879532511287,1.,0.923879532511287,1.,0.923879532511287,
1.,0.923879532511287,1.,0.923879532511287,1.,0.923879532511287,1.,0.923879532511287,
1.,0.923879532511287,1.))
REPRESENTATION_ITEM('')
);
#594=(
BOUNDED_CURVE()
B_SPLINE_CURVE(2,(#4355,#4356,#4357,#4358,#4359,#4360,#4361,#4362,#4363,
#4364,#4365,#4366,#4367,#4368,#4369,#4370,#4371),.UNSPECIFIED.,.F.,.F.)
B_SPLINE_CURVE_WITH_KNOTS((3,2,2,2,2,2,2,2,3),(0.75,0.7525,0.755,0.7575,
0.76,0.7625,0.765,0.7675,0.77),.UNSPECIFIED.)
CURVE()
GEOMETRIC_REPRESENTATION_ITEM()
RATIONAL_B_SPLINE_CURVE((1.,0.923879532511287,1.,0.923879532511287,1.,0.923879532511287,
1.,0.923879532511287,1.,0.923879532511287,1.,0.923879532511287,1.,0.923879532511287,
1.,0.923879532511287,1.))
REPRESENTATION_ITEM('')
);
#595=(
BOUNDED_CURVE()
B_SPLINE_CURVE(2,(#4372,#4373,#4374,#4375,#4376,#4377,#4378,#4379,#4380,
#4381,#4382,#4383,#4384,#4385,#4386,#4387,#4388),.UNSPECIFIED.,.F.,.F.)
B_SPLINE_CURVE_WITH_KNOTS((3,2,2,2,2,2,2,2,3),(0.75,0.7525,0.755,0.7575,
0.76,0.7625,0.765,0.7675,0.77),.UNSPECIFIED.)
CURVE()
GEOMETRIC_REPRESENTATION_ITEM()
RATIONAL_B_SPLINE_CURVE((1.,0.923879532511287,1.,0.923879532511287,1.,0.923879532511287,
1.,0.923879532511287,1.,0.923879532511287,1.,0.923879532511287,1.,0.923879532511287,
1.,0.923879532511287,1.))
REPRESENTATION_ITEM('')
);
#596=(
BOUNDED_CURVE()
B_SPLINE_CURVE(2,(#4393,#4394,#4395,#4396,#4397,#4398,#4399,#4400,#4401,
#4402,#4403,#4404,#4405,#4406,#4407,#4408,#4409),.UNSPECIFIED.,.F.,.F.)
B_SPLINE_CURVE_WITH_KNOTS((3,2,2,2,2,2,2,2,3),(0.73,0.7325,0.735,0.7375,
0.74,0.7425,0.745,0.7475,0.75),.UNSPECIFIED.)
CURVE()
GEOMETRIC_REPRESENTATION_ITEM()
RATIONAL_B_SPLINE_CURVE((1.,0.923879532511287,1.,0.923879532511287,1.,0.923879532511287,
1.,0.923879532511287,1.,0.923879532511287,1.,0.923879532511287,1.,0.923879532511287,
1.,0.923879532511287,1.))
REPRESENTATION_ITEM('')
);
#597=(
BOUNDED_CURVE()
B_SPLINE_CURVE(2,(#4410,#4411,#4412,#4413,#4414,#4415,#4416,#4417,#4418,
#4419,#4420,#4421,#4422,#4423,#4424,#4425,#4426),.UNSPECIFIED.,.F.,.F.)
B_SPLINE_CURVE_WITH_KNOTS((3,2,2,2,2,2,2,2,3),(0.73,0.7325,0.735,0.7375,
0.74,0.7425,0.745,0.7475,0.75),.UNSPECIFIED.)
CURVE()
GEOMETRIC_REPRESENTATION_ITEM()
RATIONAL_B_SPLINE_CURVE((1.,0.923879532511287,1.,0.923879532511287,1.,0.923879532511287,
1.,0.923879532511287,1.,0.923879532511287,1.,0.923879532511287,1.,0.923879532511287,
1.,0.923879532511287,1.))
REPRESENTATION_ITEM('')
);
#598=(
BOUNDED_CURVE()
B_SPLINE_CURVE(2,(#4431,#4432,#4433,#4434,#4435,#4436,#4437,#4438,#4439,
#4440,#4441,#4442,#4443,#4444,#4445,#4446,#4447),.UNSPECIFIED.,.F.,.F.)
B_SPLINE_CURVE_WITH_KNOTS((3,2,2,2,2,2,2,2,3),(0.71,0.7125,0.715,0.7175,
0.72,0.7225,0.725,0.7275,0.73),.UNSPECIFIED.)
CURVE()
GEOMETRIC_REPRESENTATION_ITEM()
RATIONAL_B_SPLINE_CURVE((1.,0.923879532511287,1.,0.923879532511287,1.,0.923879532511287,
1.,0.923879532511287,1.,0.923879532511287,1.,0.923879532511287,1.,0.923879532511287,
1.,0.923879532511287,1.))
REPRESENTATION_ITEM('')
);
#599=(
BOUNDED_CURVE()
B_SPLINE_CURVE(2,(#4448,#4449,#4450,#4451,#4452,#4453,#4454,#4455,#4456,
#4457,#4458,#4459,#4460,#4461,#4462,#4463,#4464),.UNSPECIFIED.,.F.,.F.)
B_SPLINE_CURVE_WITH_KNOTS((3,2,2,2,2,2,2,2,3),(0.71,0.7125,0.715,0.7175,
0.72,0.7225,0.725,0.7275,0.73),.UNSPECIFIED.)
CURVE()
GEOMETRIC_REPRESENTATION_ITEM()
RATIONAL_B_SPLINE_CURVE((1.,0.923879532511287,1.,0.923879532511287,1.,0.923879532511287,
1.,0.923879532511287,1.,0.923879532511287,1.,0.923879532511287,1.,0.923879532511287,
1.,0.923879532511287,1.))
REPRESENTATION_ITEM('')
);
#600=(
BOUNDED_CURVE()
B_SPLINE_CURVE(2,(#4469,#4470,#4471,#4472,#4473,#4474,#4475,#4476,#4477,
#4478,#4479,#4480,#4481,#4482,#4483,#4484,#4485),.UNSPECIFIED.,.F.,.F.)
B_SPLINE_CURVE_WITH_KNOTS((3,2,2,2,2,2,2,2,3),(0.69,0.6925,0.695,0.6975,
0.7,0.7025,0.705,0.7075,0.71),.UNSPECIFIED.)
CURVE()
GEOMETRIC_REPRESENTATION_ITEM()
RATIONAL_B_SPLINE_CURVE((1.,0.923879532511287,1.,0.923879532511287,1.,0.923879532511287,
1.,0.923879532511287,1.,0.923879532511287,1.,0.923879532511287,1.,0.923879532511287,
1.,0.923879532511287,1.))
REPRESENTATION_ITEM('')
);
#601=(
BOUNDED_CURVE()
B_SPLINE_CURVE(2,(#4486,#4487,#4488,#4489,#4490,#4491,#4492,#4493,#4494,
#4495,#4496,#4497,#4498,#4499,#4500,#4501,#4502),.UNSPECIFIED.,.F.,.F.)
B_SPLINE_CURVE_WITH_KNOTS((3,2,2,2,2,2,2,2,3),(0.69,0.6925,0.695,0.6975,
0.7,0.7025,0.705,0.7075,0.71),.UNSPECIFIED.)
CURVE()
GEOMETRIC_REPRESENTATION_ITEM()
RATIONAL_B_SPLINE_CURVE((1.,0.923879532511287,1.,0.923879532511287,1.,0.923879532511287,
1.,0.923879532511287,1.,0.923879532511287,1.,0.923879532511287,1.,0.923879532511287,
1.,0.923879532511287,1.))
REPRESENTATION_ITEM('')
);
#602=(
BOUNDED_CURVE()
B_SPLINE_CURVE(2,(#4507,#4508,#4509,#4510,#4511,#4512,#4513,#4514,#4515,
#4516,#4517,#4518,#4519,#4520,#4521,#4522,#4523),.UNSPECIFIED.,.F.,.F.)
B_SPLINE_CURVE_WITH_KNOTS((3,2,2,2,2,2,2,2,3),(0.67,0.6725,0.675,0.6775,
0.68,0.6825,0.685,0.6875,0.69),.UNSPECIFIED.)
CURVE()
GEOMETRIC_REPRESENTATION_ITEM()
RATIONAL_B_SPLINE_CURVE((1.,0.923879532511287,1.,0.923879532511287,1.,0.923879532511287,
1.,0.923879532511287,1.,0.923879532511287,1.,0.923879532511287,1.,0.923879532511287,
1.,0.923879532511287,1.))
REPRESENTATION_ITEM('')
);
#603=(
BOUNDED_CURVE()
B_SPLINE_CURVE(2,(#4524,#4525,#4526,#4527,#4528,#4529,#4530,#4531,#4532,
#4533,#4534,#4535,#4536,#4537,#4538,#4539,#4540),.UNSPECIFIED.,.F.,.F.)
B_SPLINE_CURVE_WITH_KNOTS((3,2,2,2,2,2,2,2,3),(0.67,0.6725,0.675,0.6775,
0.68,0.6825,0.685,0.6875,0.69),.UNSPECIFIED.)
CURVE()
GEOMETRIC_REPRESENTATION_ITEM()
RATIONAL_B_SPLINE_CURVE((1.,0.923879532511287,1.,0.923879532511287,1.,0.923879532511287,
1.,0.923879532511287,1.,0.923879532511287,1.,0.923879532511287,1.,0.923879532511287,
1.,0.923879532511287,1.))
REPRESENTATION_ITEM('')
);
#604=(
BOUNDED_CURVE()
B_SPLINE_CURVE(2,(#4545,#4546,#4547,#4548,#4549,#4550,#4551,#4552,#4553,
#4554,#4555,#4556,#4557,#4558,#4559,#4560,#4561),.UNSPECIFIED.,.F.,.F.)
B_SPLINE_CURVE_WITH_KNOTS((3,2,2,2,2,2,2,2,3),(0.65,0.6525,0.655,0.6575,
0.66,0.6625,0.665,0.6675,0.67),.UNSPECIFIED.)
CURVE()
GEOMETRIC_REPRESENTATION_ITEM()
RATIONAL_B_SPLINE_CURVE((1.,0.923879532511287,1.,0.923879532511287,1.,0.923879532511287,
1.,0.923879532511287,1.,0.923879532511287,1.,0.923879532511287,1.,0.923879532511287,
1.,0.923879532511287,1.))
REPRESENTATION_ITEM('')
);
#605=(
BOUNDED_CURVE()
B_SPLINE_CURVE(2,(#4562,#4563,#4564,#4565,#4566,#4567,#4568,#4569,#4570,
#4571,#4572,#4573,#4574,#4575,#4576,#4577,#4578),.UNSPECIFIED.,.F.,.F.)
B_SPLINE_CURVE_WITH_KNOTS((3,2,2,2,2,2,2,2,3),(0.65,0.6525,0.655,0.6575,
0.66,0.6625,0.665,0.6675,0.67),.UNSPECIFIED.)
CURVE()
GEOMETRIC_REPRESENTATION_ITEM()
RATIONAL_B_SPLINE_CURVE((1.,0.923879532511287,1.,0.923879532511287,1.,0.923879532511287,
1.,0.923879532511287,1.,0.923879532511287,1.,0.923879532511287,1.,0.923879532511287,
1.,0.923879532511287,1.))
REPRESENTATION_ITEM('')
);
#606=(
BOUNDED_CURVE()
B_SPLINE_CURVE(2,(#4583,#4584,#4585,#4586,#4587,#4588,#4589,#4590,#4591,
#4592,#4593,#4594,#4595,#4596,#4597,#4598,#4599),.UNSPECIFIED.,.F.,.F.)
B_SPLINE_CURVE_WITH_KNOTS((3,2,2,2,2,2,2,2,3),(0.63,0.6325,0.635,0.6375,
0.64,0.6425,0.645,0.6475,0.65),.UNSPECIFIED.)
CURVE()
GEOMETRIC_REPRESENTATION_ITEM()
RATIONAL_B_SPLINE_CURVE((1.,0.923879532511287,1.,0.923879532511287,1.,0.923879532511287,
1.,0.923879532511287,1.,0.923879532511287,1.,0.923879532511287,1.,0.923879532511287,
1.,0.923879532511287,1.))
REPRESENTATION_ITEM('')
);
#607=(
BOUNDED_CURVE()
B_SPLINE_CURVE(2,(#4600,#4601,#4602,#4603,#4604,#4605,#4606,#4607,#4608,
#4609,#4610,#4611,#4612,#4613,#4614,#4615,#4616),.UNSPECIFIED.,.F.,.F.)
B_SPLINE_CURVE_WITH_KNOTS((3,2,2,2,2,2,2,2,3),(0.63,0.6325,0.635,0.6375,
0.64,0.6425,0.645,0.6475,0.65),.UNSPECIFIED.)
CURVE()
GEOMETRIC_REPRESENTATION_ITEM()
RATIONAL_B_SPLINE_CURVE((1.,0.923879532511287,1.,0.923879532511287,1.,0.923879532511287,
1.,0.923879532511287,1.,0.923879532511287,1.,0.923879532511287,1.,0.923879532511287,
1.,0.923879532511287,1.))
REPRESENTATION_ITEM('')
);
#608=(
BOUNDED_CURVE()
B_SPLINE_CURVE(2,(#4621,#4622,#4623,#4624,#4625,#4626,#4627,#4628,#4629,
#4630,#4631,#4632,#4633,#4634,#4635,#4636,#4637),.UNSPECIFIED.,.F.,.F.)
B_SPLINE_CURVE_WITH_KNOTS((3,2,2,2,2,2,2,2,3),(0.61,0.6125,0.615,0.6175,
0.62,0.6225,0.625,0.6275,0.63),.UNSPECIFIED.)
CURVE()
GEOMETRIC_REPRESENTATION_ITEM()
RATIONAL_B_SPLINE_CURVE((1.,0.923879532511287,1.,0.923879532511287,1.,0.923879532511287,
1.,0.923879532511287,1.,0.923879532511287,1.,0.923879532511287,1.,0.923879532511287,
1.,0.923879532511287,1.))
REPRESENTATION_ITEM('')
);
#609=(
BOUNDED_CURVE()
B_SPLINE_CURVE(2,(#4638,#4639,#4640,#4641,#4642,#4643,#4644,#4645,#4646,
#4647,#4648,#4649,#4650,#4651,#4652,#4653,#4654),.UNSPECIFIED.,.F.,.F.)
B_SPLINE_CURVE_WITH_KNOTS((3,2,2,2,2,2,2,2,3),(0.61,0.6125,0.615,0.6175,
0.62,0.6225,0.625,0.6275,0.63),.UNSPECIFIED.)
CURVE()
GEOMETRIC_REPRESENTATION_ITEM()
RATIONAL_B_SPLINE_CURVE((1.,0.923879532511287,1.,0.923879532511287,1.,0.923879532511287,
1.,0.923879532511287,1.,0.923879532511287,1.,0.923879532511287,1.,0.923879532511287,
1.,0.923879532511287,1.))
REPRESENTATION_ITEM('')
);
#610=(
BOUNDED_CURVE()
B_SPLINE_CURVE(2,(#4659,#4660,#4661,#4662,#4663,#4664,#4665,#4666,#4667,
#4668,#4669,#4670,#4671,#4672,#4673,#4674,#4675),.UNSPECIFIED.,.F.,.F.)
B_SPLINE_CURVE_WITH_KNOTS((3,2,2,2,2,2,2,2,3),(0.59,0.5925,0.595,0.5975,
0.6,0.6025,0.605,0.6075,0.61),.UNSPECIFIED.)
CURVE()
GEOMETRIC_REPRESENTATION_ITEM()
RATIONAL_B_SPLINE_CURVE((1.,0.923879532511287,1.,0.923879532511287,1.,0.923879532511287,
1.,0.923879532511287,1.,0.923879532511287,1.,0.923879532511287,1.,0.923879532511287,
1.,0.923879532511287,1.))
REPRESENTATION_ITEM('')
);
#611=(
BOUNDED_CURVE()
B_SPLINE_CURVE(2,(#4676,#4677,#4678,#4679,#4680,#4681,#4682,#4683,#4684,
#4685,#4686,#4687,#4688,#4689,#4690,#4691,#4692),.UNSPECIFIED.,.F.,.F.)
B_SPLINE_CURVE_WITH_KNOTS((3,2,2,2,2,2,2,2,3),(0.59,0.5925,0.595,0.5975,
0.6,0.6025,0.605,0.6075,0.61),.UNSPECIFIED.)
CURVE()
GEOMETRIC_REPRESENTATION_ITEM()
RATIONAL_B_SPLINE_CURVE((1.,0.923879532511287,1.,0.923879532511287,1.,0.923879532511287,
1.,0.923879532511287,1.,0.923879532511287,1.,0.923879532511287,1.,0.923879532511287,
1.,0.923879532511287,1.))
REPRESENTATION_ITEM('')
);
#612=(
BOUNDED_CURVE()
B_SPLINE_CURVE(2,(#4697,#4698,#4699,#4700,#4701,#4702,#4703,#4704,#4705,
#4706,#4707,#4708,#4709,#4710,#4711,#4712,#4713),.UNSPECIFIED.,.F.,.F.)
B_SPLINE_CURVE_WITH_KNOTS((3,2,2,2,2,2,2,2,3),(0.57,0.5725,0.575,0.5775,
0.58,0.5825,0.585,0.5875,0.59),.UNSPECIFIED.)
CURVE()
GEOMETRIC_REPRESENTATION_ITEM()
RATIONAL_B_SPLINE_CURVE((1.,0.923879532511287,1.,0.923879532511287,1.,0.923879532511287,
1.,0.923879532511287,1.,0.923879532511287,1.,0.923879532511287,1.,0.923879532511287,
1.,0.923879532511287,1.))
REPRESENTATION_ITEM('')
);
#613=(
BOUNDED_CURVE()
B_SPLINE_CURVE(2,(#4714,#4715,#4716,#4717,#4718,#4719,#4720,#4721,#4722,
#4723,#4724,#4725,#4726,#4727,#4728,#4729,#4730),.UNSPECIFIED.,.F.,.F.)
B_SPLINE_CURVE_WITH_KNOTS((3,2,2,2,2,2,2,2,3),(0.57,0.5725,0.575,0.5775,
0.58,0.5825,0.585,0.5875,0.59),.UNSPECIFIED.)
CURVE()
GEOMETRIC_REPRESENTATION_ITEM()
RATIONAL_B_SPLINE_CURVE((1.,0.923879532511287,1.,0.923879532511287,1.,0.923879532511287,
1.,0.923879532511287,1.,0.923879532511287,1.,0.923879532511287,1.,0.923879532511287,
1.,0.923879532511287,1.))
REPRESENTATION_ITEM('')
);
#614=(
BOUNDED_CURVE()
B_SPLINE_CURVE(2,(#4735,#4736,#4737,#4738,#4739,#4740,#4741,#4742,#4743,
#4744,#4745,#4746,#4747,#4748,#4749,#4750,#4751),.UNSPECIFIED.,.F.,.F.)
B_SPLINE_CURVE_WITH_KNOTS((3,2,2,2,2,2,2,2,3),(0.55,0.5525,0.555,0.5575,
0.56,0.5625,0.565,0.5675,0.57),.UNSPECIFIED.)
CURVE()
GEOMETRIC_REPRESENTATION_ITEM()
RATIONAL_B_SPLINE_CURVE((1.,0.923879532511287,1.,0.923879532511287,1.,0.923879532511287,
1.,0.923879532511287,1.,0.923879532511287,1.,0.923879532511287,1.,0.923879532511287,
1.,0.923879532511287,1.))
REPRESENTATION_ITEM('')
);
#615=(
BOUNDED_CURVE()
B_SPLINE_CURVE(2,(#4752,#4753,#4754,#4755,#4756,#4757,#4758,#4759,#4760,
#4761,#4762,#4763,#4764,#4765,#4766,#4767,#4768),.UNSPECIFIED.,.F.,.F.)
B_SPLINE_CURVE_WITH_KNOTS((3,2,2,2,2,2,2,2,3),(0.55,0.5525,0.555,0.5575,
0.56,0.5625,0.565,0.5675,0.57),.UNSPECIFIED.)
CURVE()
GEOMETRIC_REPRESENTATION_ITEM()
RATIONAL_B_SPLINE_CURVE((1.,0.923879532511287,1.,0.923879532511287,1.,0.923879532511287,
1.,0.923879532511287,1.,0.923879532511287,1.,0.923879532511287,1.,0.923879532511287,
1.,0.923879532511287,1.))
REPRESENTATION_ITEM('')
);
#616=(
BOUNDED_CURVE()
B_SPLINE_CURVE(2,(#4773,#4774,#4775,#4776,#4777,#4778,#4779,#4780,#4781,
#4782,#4783,#4784,#4785,#4786,#4787,#4788,#4789),.UNSPECIFIED.,.F.,.F.)
B_SPLINE_CURVE_WITH_KNOTS((3,2,2,2,2,2,2,2,3),(0.53,0.5325,0.535,0.5375,
0.54,0.5425,0.545,0.5475,0.55),.UNSPECIFIED.)
CURVE()
GEOMETRIC_REPRESENTATION_ITEM()
RATIONAL_B_SPLINE_CURVE((1.,0.923879532511287,1.,0.923879532511287,1.,0.923879532511287,
1.,0.923879532511287,1.,0.923879532511287,1.,0.923879532511287,1.,0.923879532511287,
1.,0.923879532511287,1.))
REPRESENTATION_ITEM('')
);
#617=(
BOUNDED_CURVE()
B_SPLINE_CURVE(2,(#4790,#4791,#4792,#4793,#4794,#4795,#4796,#4797,#4798,
#4799,#4800,#4801,#4802,#4803,#4804,#4805,#4806),.UNSPECIFIED.,.F.,.F.)
B_SPLINE_CURVE_WITH_KNOTS((3,2,2,2,2,2,2,2,3),(0.53,0.5325,0.535,0.5375,
0.54,0.5425,0.545,0.5475,0.55),.UNSPECIFIED.)
CURVE()
GEOMETRIC_REPRESENTATION_ITEM()
RATIONAL_B_SPLINE_CURVE((1.,0.923879532511287,1.,0.923879532511287,1.,0.923879532511287,
1.,0.923879532511287,1.,0.923879532511287,1.,0.923879532511287,1.,0.923879532511287,
1.,0.923879532511287,1.))
REPRESENTATION_ITEM('')
);
#618=(
BOUNDED_CURVE()
B_SPLINE_CURVE(2,(#4811,#4812,#4813,#4814,#4815,#4816,#4817,#4818,#4819,
#4820,#4821,#4822,#4823,#4824,#4825,#4826,#4827),.UNSPECIFIED.,.F.,.F.)
B_SPLINE_CURVE_WITH_KNOTS((3,2,2,2,2,2,2,2,3),(0.51,0.5125,0.515,0.5175,
0.52,0.5225,0.525,0.5275,0.53),.UNSPECIFIED.)
CURVE()
GEOMETRIC_REPRESENTATION_ITEM()
RATIONAL_B_SPLINE_CURVE((1.,0.923879532511287,1.,0.923879532511287,1.,0.923879532511287,
1.,0.923879532511287,1.,0.923879532511287,1.,0.923879532511287,1.,0.923879532511287,
1.,0.923879532511287,1.))
REPRESENTATION_ITEM('')
);
#619=(
BOUNDED_CURVE()
B_SPLINE_CURVE(2,(#4828,#4829,#4830,#4831,#4832,#4833,#4834,#4835,#4836,
#4837,#4838,#4839,#4840,#4841,#4842,#4843,#4844),.UNSPECIFIED.,.F.,.F.)
B_SPLINE_CURVE_WITH_KNOTS((3,2,2,2,2,2,2,2,3),(0.51,0.5125,0.515,0.5175,
0.52,0.5225,0.525,0.5275,0.53),.UNSPECIFIED.)
CURVE()
GEOMETRIC_REPRESENTATION_ITEM()
RATIONAL_B_SPLINE_CURVE((1.,0.923879532511287,1.,0.923879532511287,1.,0.923879532511287,
1.,0.923879532511287,1.,0.923879532511287,1.,0.923879532511287,1.,0.923879532511287,
1.,0.923879532511287,1.))
REPRESENTATION_ITEM('')
);
#620=(
BOUNDED_CURVE()
B_SPLINE_CURVE(2,(#4849,#4850,#4851,#4852,#4853,#4854,#4855,#4856,#4857,
#4858,#4859,#4860,#4861,#4862,#4863,#4864,#4865),.UNSPECIFIED.,.F.,.F.)
B_SPLINE_CURVE_WITH_KNOTS((3,2,2,2,2,2,2,2,3),(0.49,0.4925,0.495,0.4975,
0.5,0.5025,0.505,0.5075,0.51),.UNSPECIFIED.)
CURVE()
GEOMETRIC_REPRESENTATION_ITEM()
RATIONAL_B_SPLINE_CURVE((1.,0.923879532511287,1.,0.923879532511287,1.,0.923879532511287,
1.,0.923879532511287,1.,0.923879532511287,1.,0.923879532511287,1.,0.923879532511287,
1.,0.923879532511287,1.))
REPRESENTATION_ITEM('')
);
#621=(
BOUNDED_CURVE()
B_SPLINE_CURVE(2,(#4866,#4867,#4868,#4869,#4870,#4871,#4872,#4873,#4874,
#4875,#4876,#4877,#4878,#4879,#4880,#4881,#4882),.UNSPECIFIED.,.F.,.F.)
B_SPLINE_CURVE_WITH_KNOTS((3,2,2,2,2,2,2,2,3),(0.49,0.4925,0.495,0.4975,
0.5,0.5025,0.505,0.5075,0.51),.UNSPECIFIED.)
CURVE()
GEOMETRIC_REPRESENTATION_ITEM()
RATIONAL_B_SPLINE_CURVE((1.,0.923879532511287,1.,0.923879532511287,1.,0.923879532511287,
1.,0.923879532511287,1.,0.923879532511287,1.,0.923879532511287,1.,0.923879532511287,
1.,0.923879532511287,1.))
REPRESENTATION_ITEM('')
);
#622=(
BOUNDED_CURVE()
B_SPLINE_CURVE(2,(#4887,#4888,#4889,#4890,#4891,#4892,#4893,#4894,#4895,
#4896,#4897,#4898,#4899,#4900,#4901,#4902,#4903),.UNSPECIFIED.,.F.,.F.)
B_SPLINE_CURVE_WITH_KNOTS((3,2,2,2,2,2,2,2,3),(0.47,0.4725,0.475,0.4775,
0.48,0.4825,0.485,0.4875,0.49),.UNSPECIFIED.)
CURVE()
GEOMETRIC_REPRESENTATION_ITEM()
RATIONAL_B_SPLINE_CURVE((1.,0.923879532511287,1.,0.923879532511287,1.,0.923879532511287,
1.,0.923879532511287,1.,0.923879532511287,1.,0.923879532511287,1.,0.923879532511287,
1.,0.923879532511287,1.))
REPRESENTATION_ITEM('')
);
#623=(
BOUNDED_CURVE()
B_SPLINE_CURVE(2,(#4904,#4905,#4906,#4907,#4908,#4909,#4910,#4911,#4912,
#4913,#4914,#4915,#4916,#4917,#4918,#4919,#4920),.UNSPECIFIED.,.F.,.F.)
B_SPLINE_CURVE_WITH_KNOTS((3,2,2,2,2,2,2,2,3),(0.47,0.4725,0.475,0.4775,
0.48,0.4825,0.485,0.4875,0.49),.UNSPECIFIED.)
CURVE()
GEOMETRIC_REPRESENTATION_ITEM()
RATIONAL_B_SPLINE_CURVE((1.,0.923879532511287,1.,0.923879532511287,1.,0.923879532511287,
1.,0.923879532511287,1.,0.923879532511287,1.,0.923879532511287,1.,0.923879532511287,
1.,0.923879532511287,1.))
REPRESENTATION_ITEM('')
);
#624=(
BOUNDED_CURVE()
B_SPLINE_CURVE(2,(#4925,#4926,#4927,#4928,#4929,#4930,#4931,#4932,#4933,
#4934,#4935,#4936,#4937,#4938,#4939,#4940,#4941),.UNSPECIFIED.,.F.,.F.)
B_SPLINE_CURVE_WITH_KNOTS((3,2,2,2,2,2,2,2,3),(0.45,0.4525,0.455,0.4575,
0.46,0.4625,0.465,0.4675,0.47),.UNSPECIFIED.)
CURVE()
GEOMETRIC_REPRESENTATION_ITEM()
RATIONAL_B_SPLINE_CURVE((1.,0.923879532511287,1.,0.923879532511287,1.,0.923879532511287,
1.,0.923879532511287,1.,0.923879532511287,1.,0.923879532511287,1.,0.923879532511287,
1.,0.923879532511287,1.))
REPRESENTATION_ITEM('')
);
#625=(
BOUNDED_CURVE()
B_SPLINE_CURVE(2,(#4942,#4943,#4944,#4945,#4946,#4947,#4948,#4949,#4950,
#4951,#4952,#4953,#4954,#4955,#4956,#4957,#4958),.UNSPECIFIED.,.F.,.F.)
B_SPLINE_CURVE_WITH_KNOTS((3,2,2,2,2,2,2,2,3),(0.45,0.4525,0.455,0.4575,
0.46,0.4625,0.465,0.4675,0.47),.UNSPECIFIED.)
CURVE()
GEOMETRIC_REPRESENTATION_ITEM()
RATIONAL_B_SPLINE_CURVE((1.,0.923879532511287,1.,0.923879532511287,1.,0.923879532511287,
1.,0.923879532511287,1.,0.923879532511287,1.,0.923879532511287,1.,0.923879532511287,
1.,0.923879532511287,1.))
REPRESENTATION_ITEM('')
);
#626=(
BOUNDED_CURVE()
B_SPLINE_CURVE(2,(#4963,#4964,#4965,#4966,#4967,#4968,#4969,#4970,#4971,
#4972,#4973,#4974,#4975,#4976,#4977,#4978,#4979),.UNSPECIFIED.,.F.,.F.)
B_SPLINE_CURVE_WITH_KNOTS((3,2,2,2,2,2,2,2,3),(0.43,0.4325,0.435,0.4375,
0.44,0.4425,0.445,0.4475,0.45),.UNSPECIFIED.)
CURVE()
GEOMETRIC_REPRESENTATION_ITEM()
RATIONAL_B_SPLINE_CURVE((1.,0.923879532511287,1.,0.923879532511287,1.,0.923879532511287,
1.,0.923879532511287,1.,0.923879532511287,1.,0.923879532511287,1.,0.923879532511287,
1.,0.923879532511287,1.))
REPRESENTATION_ITEM('')
);
#627=(
BOUNDED_CURVE()
B_SPLINE_CURVE(2,(#4980,#4981,#4982,#4983,#4984,#4985,#4986,#4987,#4988,
#4989,#4990,#4991,#4992,#4993,#4994,#4995,#4996),.UNSPECIFIED.,.F.,.F.)
B_SPLINE_CURVE_WITH_KNOTS((3,2,2,2,2,2,2,2,3),(0.43,0.4325,0.435,0.4375,
0.44,0.4425,0.445,0.4475,0.45),.UNSPECIFIED.)
CURVE()
GEOMETRIC_REPRESENTATION_ITEM()
RATIONAL_B_SPLINE_CURVE((1.,0.923879532511287,1.,0.923879532511287,1.,0.923879532511287,
1.,0.923879532511287,1.,0.923879532511287,1.,0.923879532511287,1.,0.923879532511287,
1.,0.923879532511287,1.))
REPRESENTATION_ITEM('')
);
#628=(
BOUNDED_CURVE()
B_SPLINE_CURVE(2,(#5001,#5002,#5003,#5004,#5005,#5006,#5007,#5008,#5009,
#5010,#5011,#5012,#5013,#5014,#5015,#5016,#5017),.UNSPECIFIED.,.F.,.F.)
B_SPLINE_CURVE_WITH_KNOTS((3,2,2,2,2,2,2,2,3),(0.41,0.4125,0.415,0.4175,
0.42,0.4225,0.425,0.4275,0.43),.UNSPECIFIED.)
CURVE()
GEOMETRIC_REPRESENTATION_ITEM()
RATIONAL_B_SPLINE_CURVE((1.,0.923879532511287,1.,0.923879532511287,1.,0.923879532511287,
1.,0.923879532511287,1.,0.923879532511287,1.,0.923879532511287,1.,0.923879532511287,
1.,0.923879532511287,1.))
REPRESENTATION_ITEM('')
);
#629=(
BOUNDED_CURVE()
B_SPLINE_CURVE(2,(#5018,#5019,#5020,#5021,#5022,#5023,#5024,#5025,#5026,
#5027,#5028,#5029,#5030,#5031,#5032,#5033,#5034),.UNSPECIFIED.,.F.,.F.)
B_SPLINE_CURVE_WITH_KNOTS((3,2,2,2,2,2,2,2,3),(0.41,0.4125,0.415,0.4175,
0.42,0.4225,0.425,0.4275,0.43),.UNSPECIFIED.)
CURVE()
GEOMETRIC_REPRESENTATION_ITEM()
RATIONAL_B_SPLINE_CURVE((1.,0.923879532511287,1.,0.923879532511287,1.,0.923879532511287,
1.,0.923879532511287,1.,0.923879532511287,1.,0.923879532511287,1.,0.923879532511287,
1.,0.923879532511287,1.))
REPRESENTATION_ITEM('')
);
#630=(
BOUNDED_CURVE()
B_SPLINE_CURVE(2,(#5039,#5040,#5041,#5042,#5043,#5044,#5045,#5046,#5047,
#5048,#5049,#5050,#5051,#5052,#5053,#5054,#5055),.UNSPECIFIED.,.F.,.F.)
B_SPLINE_CURVE_WITH_KNOTS((3,2,2,2,2,2,2,2,3),(0.39,0.3925,0.395,0.3975,
0.4,0.4025,0.405,0.4075,0.41),.UNSPECIFIED.)
CURVE()
GEOMETRIC_REPRESENTATION_ITEM()
RATIONAL_B_SPLINE_CURVE((1.,0.923879532511287,1.,0.923879532511287,1.,0.923879532511287,
1.,0.923879532511287,1.,0.923879532511287,1.,0.923879532511287,1.,0.923879532511287,
1.,0.923879532511287,1.))
REPRESENTATION_ITEM('')
);
#631=(
BOUNDED_CURVE()
B_SPLINE_CURVE(2,(#5056,#5057,#5058,#5059,#5060,#5061,#5062,#5063,#5064,
#5065,#5066,#5067,#5068,#5069,#5070,#5071,#5072),.UNSPECIFIED.,.F.,.F.)
B_SPLINE_CURVE_WITH_KNOTS((3,2,2,2,2,2,2,2,3),(0.39,0.3925,0.395,0.3975,
0.4,0.4025,0.405,0.4075,0.41),.UNSPECIFIED.)
CURVE()
GEOMETRIC_REPRESENTATION_ITEM()
RATIONAL_B_SPLINE_CURVE((1.,0.923879532511287,1.,0.923879532511287,1.,0.923879532511287,
1.,0.923879532511287,1.,0.923879532511287,1.,0.923879532511287,1.,0.923879532511287,
1.,0.923879532511287,1.))
REPRESENTATION_ITEM('')
);
#632=(
BOUNDED_CURVE()
B_SPLINE_CURVE(2,(#5077,#5078,#5079,#5080,#5081,#5082,#5083,#5084,#5085,
#5086,#5087,#5088,#5089,#5090,#5091,#5092,#5093),.UNSPECIFIED.,.F.,.F.)
B_SPLINE_CURVE_WITH_KNOTS((3,2,2,2,2,2,2,2,3),(0.37,0.3725,0.375,0.3775,
0.38,0.3825,0.385,0.3875,0.39),.UNSPECIFIED.)
CURVE()
GEOMETRIC_REPRESENTATION_ITEM()
RATIONAL_B_SPLINE_CURVE((1.,0.923879532511287,1.,0.923879532511287,1.,0.923879532511287,
1.,0.923879532511287,1.,0.923879532511287,1.,0.923879532511287,1.,0.923879532511287,
1.,0.923879532511287,1.))
REPRESENTATION_ITEM('')
);
#633=(
BOUNDED_CURVE()
B_SPLINE_CURVE(2,(#5094,#5095,#5096,#5097,#5098,#5099,#5100,#5101,#5102,
#5103,#5104,#5105,#5106,#5107,#5108,#5109,#5110),.UNSPECIFIED.,.F.,.F.)
B_SPLINE_CURVE_WITH_KNOTS((3,2,2,2,2,2,2,2,3),(0.37,0.3725,0.375,0.3775,
0.38,0.3825,0.385,0.3875,0.39),.UNSPECIFIED.)
CURVE()
GEOMETRIC_REPRESENTATION_ITEM()
RATIONAL_B_SPLINE_CURVE((1.,0.923879532511287,1.,0.923879532511287,1.,0.923879532511287,
1.,0.923879532511287,1.,0.923879532511287,1.,0.923879532511287,1.,0.923879532511287,
1.,0.923879532511287,1.))
REPRESENTATION_ITEM('')
);
#634=(
BOUNDED_CURVE()
B_SPLINE_CURVE(2,(#5115,#5116,#5117,#5118,#5119,#5120,#5121,#5122,#5123,
#5124,#5125,#5126,#5127,#5128,#5129,#5130,#5131),.UNSPECIFIED.,.F.,.F.)
B_SPLINE_CURVE_WITH_KNOTS((3,2,2,2,2,2,2,2,3),(0.35,0.3525,0.355,0.3575,
0.36,0.3625,0.365,0.3675,0.37),.UNSPECIFIED.)
CURVE()
GEOMETRIC_REPRESENTATION_ITEM()
RATIONAL_B_SPLINE_CURVE((1.,0.923879532511287,1.,0.923879532511287,1.,0.923879532511287,
1.,0.923879532511287,1.,0.923879532511287,1.,0.923879532511287,1.,0.923879532511287,
1.,0.923879532511287,1.))
REPRESENTATION_ITEM('')
);
#635=(
BOUNDED_CURVE()
B_SPLINE_CURVE(2,(#5132,#5133,#5134,#5135,#5136,#5137,#5138,#5139,#5140,
#5141,#5142,#5143,#5144,#5145,#5146,#5147,#5148),.UNSPECIFIED.,.F.,.F.)
B_SPLINE_CURVE_WITH_KNOTS((3,2,2,2,2,2,2,2,3),(0.35,0.3525,0.355,0.3575,
0.36,0.3625,0.365,0.3675,0.37),.UNSPECIFIED.)
CURVE()
GEOMETRIC_REPRESENTATION_ITEM()
RATIONAL_B_SPLINE_CURVE((1.,0.923879532511287,1.,0.923879532511287,1.,0.923879532511287,
1.,0.923879532511287,1.,0.923879532511287,1.,0.923879532511287,1.,0.923879532511287,
1.,0.923879532511287,1.))
REPRESENTATION_ITEM('')
);
#636=(
BOUNDED_CURVE()
B_SPLINE_CURVE(2,(#5153,#5154,#5155,#5156,#5157,#5158,#5159,#5160,#5161,
#5162,#5163,#5164,#5165,#5166,#5167,#5168,#5169),.UNSPECIFIED.,.F.,.F.)
B_SPLINE_CURVE_WITH_KNOTS((3,2,2,2,2,2,2,2,3),(0.33,0.3325,0.335,0.3375,
0.34,0.3425,0.345,0.3475,0.35),.UNSPECIFIED.)
CURVE()
GEOMETRIC_REPRESENTATION_ITEM()
RATIONAL_B_SPLINE_CURVE((1.,0.923879532511287,1.,0.923879532511287,1.,0.923879532511287,
1.,0.923879532511287,1.,0.923879532511287,1.,0.923879532511287,1.,0.923879532511287,
1.,0.923879532511287,1.))
REPRESENTATION_ITEM('')
);
#637=(
BOUNDED_CURVE()
B_SPLINE_CURVE(2,(#5170,#5171,#5172,#5173,#5174,#5175,#5176,#5177,#5178,
#5179,#5180,#5181,#5182,#5183,#5184,#5185,#5186),.UNSPECIFIED.,.F.,.F.)
B_SPLINE_CURVE_WITH_KNOTS((3,2,2,2,2,2,2,2,3),(0.33,0.3325,0.335,0.3375,
0.34,0.3425,0.345,0.3475,0.35),.UNSPECIFIED.)
CURVE()
GEOMETRIC_REPRESENTATION_ITEM()
RATIONAL_B_SPLINE_CURVE((1.,0.923879532511287,1.,0.923879532511287,1.,0.923879532511287,
1.,0.923879532511287,1.,0.923879532511287,1.,0.923879532511287,1.,0.923879532511287,
1.,0.923879532511287,1.))
REPRESENTATION_ITEM('')
);
#638=(
BOUNDED_CURVE()
B_SPLINE_CURVE(2,(#5191,#5192,#5193,#5194,#5195,#5196,#5197,#5198,#5199,
#5200,#5201,#5202,#5203,#5204,#5205,#5206,#5207),.UNSPECIFIED.,.F.,.F.)
B_SPLINE_CURVE_WITH_KNOTS((3,2,2,2,2,2,2,2,3),(0.31,0.3125,0.315,0.3175,
0.32,0.3225,0.325,0.3275,0.33),.UNSPECIFIED.)
CURVE()
GEOMETRIC_REPRESENTATION_ITEM()
RATIONAL_B_SPLINE_CURVE((1.,0.923879532511287,1.,0.923879532511287,1.,0.923879532511287,
1.,0.923879532511287,1.,0.923879532511287,1.,0.923879532511287,1.,0.923879532511287,
1.,0.923879532511287,1.))
REPRESENTATION_ITEM('')
);
#639=(
BOUNDED_CURVE()
B_SPLINE_CURVE(2,(#5208,#5209,#5210,#5211,#5212,#5213,#5214,#5215,#5216,
#5217,#5218,#5219,#5220,#5221,#5222,#5223,#5224),.UNSPECIFIED.,.F.,.F.)
B_SPLINE_CURVE_WITH_KNOTS((3,2,2,2,2,2,2,2,3),(0.31,0.3125,0.315,0.3175,
0.32,0.3225,0.325,0.3275,0.33),.UNSPECIFIED.)
CURVE()
GEOMETRIC_REPRESENTATION_ITEM()
RATIONAL_B_SPLINE_CURVE((1.,0.923879532511287,1.,0.923879532511287,1.,0.923879532511287,
1.,0.923879532511287,1.,0.923879532511287,1.,0.923879532511287,1.,0.923879532511287,
1.,0.923879532511287,1.))
REPRESENTATION_ITEM('')
);
#640=(
BOUNDED_CURVE()
B_SPLINE_CURVE(2,(#5229,#5230,#5231,#5232,#5233,#5234,#5235,#5236,#5237,
#5238,#5239,#5240,#5241,#5242,#5243,#5244,#5245),.UNSPECIFIED.,.F.,.F.)
B_SPLINE_CURVE_WITH_KNOTS((3,2,2,2,2,2,2,2,3),(0.29,0.2925,0.295,0.2975,
0.3,0.3025,0.305,0.3075,0.31),.UNSPECIFIED.)
CURVE()
GEOMETRIC_REPRESENTATION_ITEM()
RATIONAL_B_SPLINE_CURVE((1.,0.923879532511287,1.,0.923879532511287,1.,0.923879532511287,
1.,0.923879532511287,1.,0.923879532511287,1.,0.923879532511287,1.,0.923879532511287,
1.,0.923879532511287,1.))
REPRESENTATION_ITEM('')
);
#641=(
BOUNDED_CURVE()
B_SPLINE_CURVE(2,(#5246,#5247,#5248,#5249,#5250,#5251,#5252,#5253,#5254,
#5255,#5256,#5257,#5258,#5259,#5260,#5261,#5262),.UNSPECIFIED.,.F.,.F.)
B_SPLINE_CURVE_WITH_KNOTS((3,2,2,2,2,2,2,2,3),(0.29,0.2925,0.295,0.2975,
0.3,0.3025,0.305,0.3075,0.31),.UNSPECIFIED.)
CURVE()
GEOMETRIC_REPRESENTATION_ITEM()
RATIONAL_B_SPLINE_CURVE((1.,0.923879532511287,1.,0.923879532511287,1.,0.923879532511287,
1.,0.923879532511287,1.,0.923879532511287,1.,0.923879532511287,1.,0.923879532511287,
1.,0.923879532511287,1.))
REPRESENTATION_ITEM('')
);
#642=(
BOUNDED_CURVE()
B_SPLINE_CURVE(2,(#5267,#5268,#5269,#5270,#5271,#5272,#5273,#5274,#5275,
#5276,#5277,#5278,#5279,#5280,#5281,#5282,#5283),.UNSPECIFIED.,.F.,.F.)
B_SPLINE_CURVE_WITH_KNOTS((3,2,2,2,2,2,2,2,3),(0.27,0.2725,0.275,0.2775,
0.28,0.2825,0.285,0.2875,0.29),.UNSPECIFIED.)
CURVE()
GEOMETRIC_REPRESENTATION_ITEM()
RATIONAL_B_SPLINE_CURVE((1.,0.923879532511287,1.,0.923879532511287,1.,0.923879532511287,
1.,0.923879532511287,1.,0.923879532511287,1.,0.923879532511287,1.,0.923879532511287,
1.,0.923879532511287,1.))
REPRESENTATION_ITEM('')
);
#643=(
BOUNDED_CURVE()
B_SPLINE_CURVE(2,(#5284,#5285,#5286,#5287,#5288,#5289,#5290,#5291,#5292,
#5293,#5294,#5295,#5296,#5297,#5298,#5299,#5300),.UNSPECIFIED.,.F.,.F.)
B_SPLINE_CURVE_WITH_KNOTS((3,2,2,2,2,2,2,2,3),(0.27,0.2725,0.275,0.2775,
0.28,0.2825,0.285,0.2875,0.29),.UNSPECIFIED.)
CURVE()
GEOMETRIC_REPRESENTATION_ITEM()
RATIONAL_B_SPLINE_CURVE((1.,0.923879532511287,1.,0.923879532511287,1.,0.923879532511287,
1.,0.923879532511287,1.,0.923879532511287,1.,0.923879532511287,1.,0.923879532511287,
1.,0.923879532511287,1.))
REPRESENTATION_ITEM('')
);
#644=(
BOUNDED_CURVE()
B_SPLINE_CURVE(2,(#5305,#5306,#5307,#5308,#5309,#5310,#5311,#5312,#5313,
#5314,#5315,#5316,#5317,#5318,#5319,#5320,#5321),.UNSPECIFIED.,.F.,.F.)
B_SPLINE_CURVE_WITH_KNOTS((3,2,2,2,2,2,2,2,3),(0.25,0.2525,0.255,0.2575,
0.26,0.2625,0.265,0.2675,0.27),.UNSPECIFIED.)
CURVE()
GEOMETRIC_REPRESENTATION_ITEM()
RATIONAL_B_SPLINE_CURVE((1.,0.923879532511287,1.,0.923879532511287,1.,0.923879532511287,
1.,0.923879532511287,1.,0.923879532511287,1.,0.923879532511287,1.,0.923879532511287,
1.,0.923879532511287,1.))
REPRESENTATION_ITEM('')
);
#645=(
BOUNDED_CURVE()
B_SPLINE_CURVE(2,(#5322,#5323,#5324,#5325,#5326,#5327,#5328,#5329,#5330,
#5331,#5332,#5333,#5334,#5335,#5336,#5337,#5338),.UNSPECIFIED.,.F.,.F.)
B_SPLINE_CURVE_WITH_KNOTS((3,2,2,2,2,2,2,2,3),(0.25,0.2525,0.255,0.2575,
0.26,0.2625,0.265,0.2675,0.27),.UNSPECIFIED.)
CURVE()
GEOMETRIC_REPRESENTATION_ITEM()
RATIONAL_B_SPLINE_CURVE((1.,0.923879532511287,1.,0.923879532511287,1.,0.923879532511287,
1.,0.923879532511287,1.,0.923879532511287,1.,0.923879532511287,1.,0.923879532511287,
1.,0.923879532511287,1.))
REPRESENTATION_ITEM('')
);
#646=(
BOUNDED_CURVE()
B_SPLINE_CURVE(2,(#5343,#5344,#5345,#5346,#5347,#5348,#5349,#5350,#5351,
#5352,#5353,#5354,#5355,#5356,#5357,#5358,#5359),.UNSPECIFIED.,.F.,.F.)
B_SPLINE_CURVE_WITH_KNOTS((3,2,2,2,2,2,2,2,3),(0.23,0.2325,0.235,0.2375,
0.24,0.2425,0.245,0.2475,0.25),.UNSPECIFIED.)
CURVE()
GEOMETRIC_REPRESENTATION_ITEM()
RATIONAL_B_SPLINE_CURVE((1.,0.923879532511287,1.,0.923879532511287,1.,0.923879532511287,
1.,0.923879532511287,1.,0.923879532511287,1.,0.923879532511287,1.,0.923879532511287,
1.,0.923879532511287,1.))
REPRESENTATION_ITEM('')
);
#647=(
BOUNDED_CURVE()
B_SPLINE_CURVE(2,(#5360,#5361,#5362,#5363,#5364,#5365,#5366,#5367,#5368,
#5369,#5370,#5371,#5372,#5373,#5374,#5375,#5376),.UNSPECIFIED.,.F.,.F.)
B_SPLINE_CURVE_WITH_KNOTS((3,2,2,2,2,2,2,2,3),(0.23,0.2325,0.235,0.2375,
0.24,0.2425,0.245,0.2475,0.25),.UNSPECIFIED.)
CURVE()
GEOMETRIC_REPRESENTATION_ITEM()
RATIONAL_B_SPLINE_CURVE((1.,0.923879532511287,1.,0.923879532511287,1.,0.923879532511287,
1.,0.923879532511287,1.,0.923879532511287,1.,0.923879532511287,1.,0.923879532511287,
1.,0.923879532511287,1.))
REPRESENTATION_ITEM('')
);
#648=(
BOUNDED_CURVE()
B_SPLINE_CURVE(2,(#5381,#5382,#5383,#5384,#5385,#5386,#5387,#5388,#5389,
#5390,#5391,#5392,#5393,#5394,#5395,#5396,#5397),.UNSPECIFIED.,.F.,.F.)
B_SPLINE_CURVE_WITH_KNOTS((3,2,2,2,2,2,2,2,3),(0.21,0.2125,0.215,0.2175,
0.22,0.2225,0.225,0.2275,0.23),.UNSPECIFIED.)
CURVE()
GEOMETRIC_REPRESENTATION_ITEM()
RATIONAL_B_SPLINE_CURVE((1.,0.923879532511287,1.,0.923879532511287,1.,0.923879532511287,
1.,0.923879532511287,1.,0.923879532511287,1.,0.923879532511287,1.,0.923879532511287,
1.,0.923879532511287,1.))
REPRESENTATION_ITEM('')
);
#649=(
BOUNDED_CURVE()
B_SPLINE_CURVE(2,(#5398,#5399,#5400,#5401,#5402,#5403,#5404,#5405,#5406,
#5407,#5408,#5409,#5410,#5411,#5412,#5413,#5414),.UNSPECIFIED.,.F.,.F.)
B_SPLINE_CURVE_WITH_KNOTS((3,2,2,2,2,2,2,2,3),(0.21,0.2125,0.215,0.2175,
0.22,0.2225,0.225,0.2275,0.23),.UNSPECIFIED.)
CURVE()
GEOMETRIC_REPRESENTATION_ITEM()
RATIONAL_B_SPLINE_CURVE((1.,0.923879532511287,1.,0.923879532511287,1.,0.923879532511287,
1.,0.923879532511287,1.,0.923879532511287,1.,0.923879532511287,1.,0.923879532511287,
1.,0.923879532511287,1.))
REPRESENTATION_ITEM('')
);
#650=(
BOUNDED_CURVE()
B_SPLINE_CURVE(2,(#5419,#5420,#5421,#5422,#5423,#5424,#5425,#5426,#5427,
#5428,#5429,#5430,#5431,#5432,#5433,#5434,#5435),.UNSPECIFIED.,.F.,.F.)
B_SPLINE_CURVE_WITH_KNOTS((3,2,2,2,2,2,2,2,3),(0.19,0.1925,0.195,0.1975,
0.2,0.2025,0.205,0.2075,0.21),.UNSPECIFIED.)
CURVE()
GEOMETRIC_REPRESENTATION_ITEM()
RATIONAL_B_SPLINE_CURVE((1.,0.923879532511287,1.,0.923879532511287,1.,0.923879532511287,
1.,0.923879532511287,1.,0.923879532511287,1.,0.923879532511287,1.,0.923879532511287,
1.,0.923879532511287,1.))
REPRESENTATION_ITEM('')
);
#651=(
BOUNDED_CURVE()
B_SPLINE_CURVE(2,(#5436,#5437,#5438,#5439,#5440,#5441,#5442,#5443,#5444,
#5445,#5446,#5447,#5448,#5449,#5450,#5451,#5452),.UNSPECIFIED.,.F.,.F.)
B_SPLINE_CURVE_WITH_KNOTS((3,2,2,2,2,2,2,2,3),(0.19,0.1925,0.195,0.1975,
0.2,0.2025,0.205,0.2075,0.21),.UNSPECIFIED.)
CURVE()
GEOMETRIC_REPRESENTATION_ITEM()
RATIONAL_B_SPLINE_CURVE((1.,0.923879532511287,1.,0.923879532511287,1.,0.923879532511287,
1.,0.923879532511287,1.,0.923879532511287,1.,0.923879532511287,1.,0.923879532511287,
1.,0.923879532511287,1.))
REPRESENTATION_ITEM('')
);
#652=(
BOUNDED_CURVE()
B_SPLINE_CURVE(2,(#5457,#5458,#5459,#5460,#5461,#5462,#5463,#5464,#5465,
#5466,#5467,#5468,#5469,#5470,#5471,#5472,#5473),.UNSPECIFIED.,.F.,.F.)
B_SPLINE_CURVE_WITH_KNOTS((3,2,2,2,2,2,2,2,3),(0.17,0.1725,0.175,0.1775,
0.18,0.1825,0.185,0.1875,0.19),.UNSPECIFIED.)
CURVE()
GEOMETRIC_REPRESENTATION_ITEM()
RATIONAL_B_SPLINE_CURVE((1.,0.923879532511287,1.,0.923879532511287,1.,0.923879532511287,
1.,0.923879532511287,1.,0.923879532511287,1.,0.923879532511287,1.,0.923879532511287,
1.,0.923879532511287,1.))
REPRESENTATION_ITEM('')
);
#653=(
BOUNDED_CURVE()
B_SPLINE_CURVE(2,(#5474,#5475,#5476,#5477,#5478,#5479,#5480,#5481,#5482,
#5483,#5484,#5485,#5486,#5487,#5488,#5489,#5490),.UNSPECIFIED.,.F.,.F.)
B_SPLINE_CURVE_WITH_KNOTS((3,2,2,2,2,2,2,2,3),(0.17,0.1725,0.175,0.1775,
0.18,0.1825,0.185,0.1875,0.19),.UNSPECIFIED.)
CURVE()
GEOMETRIC_REPRESENTATION_ITEM()
RATIONAL_B_SPLINE_CURVE((1.,0.923879532511287,1.,0.923879532511287,1.,0.923879532511287,
1.,0.923879532511287,1.,0.923879532511287,1.,0.923879532511287,1.,0.923879532511287,
1.,0.923879532511287,1.))
REPRESENTATION_ITEM('')
);
#654=(
BOUNDED_CURVE()
B_SPLINE_CURVE(2,(#5495,#5496,#5497,#5498,#5499,#5500,#5501,#5502,#5503,
#5504,#5505,#5506,#5507,#5508,#5509,#5510,#5511),.UNSPECIFIED.,.F.,.F.)
B_SPLINE_CURVE_WITH_KNOTS((3,2,2,2,2,2,2,2,3),(0.15,0.1525,0.155,0.1575,
0.16,0.1625,0.165,0.1675,0.17),.UNSPECIFIED.)
CURVE()
GEOMETRIC_REPRESENTATION_ITEM()
RATIONAL_B_SPLINE_CURVE((1.,0.923879532511287,1.,0.923879532511287,1.,0.923879532511287,
1.,0.923879532511287,1.,0.923879532511287,1.,0.923879532511287,1.,0.923879532511287,
1.,0.923879532511287,1.))
REPRESENTATION_ITEM('')
);
#655=(
BOUNDED_CURVE()
B_SPLINE_CURVE(2,(#5512,#5513,#5514,#5515,#5516,#5517,#5518,#5519,#5520,
#5521,#5522,#5523,#5524,#5525,#5526,#5527,#5528),.UNSPECIFIED.,.F.,.F.)
B_SPLINE_CURVE_WITH_KNOTS((3,2,2,2,2,2,2,2,3),(0.15,0.1525,0.155,0.1575,
0.16,0.1625,0.165,0.1675,0.17),.UNSPECIFIED.)
CURVE()
GEOMETRIC_REPRESENTATION_ITEM()
RATIONAL_B_SPLINE_CURVE((1.,0.923879532511287,1.,0.923879532511287,1.,0.923879532511287,
1.,0.923879532511287,1.,0.923879532511287,1.,0.923879532511287,1.,0.923879532511287,
1.,0.923879532511287,1.))
REPRESENTATION_ITEM('')
);
#656=(
BOUNDED_CURVE()
B_SPLINE_CURVE(2,(#5533,#5534,#5535,#5536,#5537,#5538,#5539,#5540,#5541,
#5542,#5543,#5544,#5545,#5546,#5547,#5548,#5549),.UNSPECIFIED.,.F.,.F.)
B_SPLINE_CURVE_WITH_KNOTS((3,2,2,2,2,2,2,2,3),(0.13,0.1325,0.135,0.1375,
0.14,0.1425,0.145,0.1475,0.15),.UNSPECIFIED.)
CURVE()
GEOMETRIC_REPRESENTATION_ITEM()
RATIONAL_B_SPLINE_CURVE((1.,0.923879532511287,1.,0.923879532511287,1.,0.923879532511287,
1.,0.923879532511287,1.,0.923879532511287,1.,0.923879532511287,1.,0.923879532511287,
1.,0.923879532511287,1.))
REPRESENTATION_ITEM('')
);
#657=(
BOUNDED_CURVE()
B_SPLINE_CURVE(2,(#5550,#5551,#5552,#5553,#5554,#5555,#5556,#5557,#5558,
#5559,#5560,#5561,#5562,#5563,#5564,#5565,#5566),.UNSPECIFIED.,.F.,.F.)
B_SPLINE_CURVE_WITH_KNOTS((3,2,2,2,2,2,2,2,3),(0.13,0.1325,0.135,0.1375,
0.14,0.1425,0.145,0.1475,0.15),.UNSPECIFIED.)
CURVE()
GEOMETRIC_REPRESENTATION_ITEM()
RATIONAL_B_SPLINE_CURVE((1.,0.923879532511287,1.,0.923879532511287,1.,0.923879532511287,
1.,0.923879532511287,1.,0.923879532511287,1.,0.923879532511287,1.,0.923879532511287,
1.,0.923879532511287,1.))
REPRESENTATION_ITEM('')
);
#658=(
BOUNDED_CURVE()
B_SPLINE_CURVE(2,(#5571,#5572,#5573,#5574,#5575,#5576,#5577,#5578,#5579,
#5580,#5581,#5582,#5583,#5584,#5585,#5586,#5587),.UNSPECIFIED.,.F.,.F.)
B_SPLINE_CURVE_WITH_KNOTS((3,2,2,2,2,2,2,2,3),(0.11,0.1125,0.115,0.1175,
0.12,0.1225,0.125,0.1275,0.13),.UNSPECIFIED.)
CURVE()
GEOMETRIC_REPRESENTATION_ITEM()
RATIONAL_B_SPLINE_CURVE((1.,0.923879532511287,1.,0.923879532511287,1.,0.923879532511287,
1.,0.923879532511287,1.,0.923879532511287,1.,0.923879532511287,1.,0.923879532511287,
1.,0.923879532511287,1.))
REPRESENTATION_ITEM('')
);
#659=(
BOUNDED_CURVE()
B_SPLINE_CURVE(2,(#5588,#5589,#5590,#5591,#5592,#5593,#5594,#5595,#5596,
#5597,#5598,#5599,#5600,#5601,#5602,#5603,#5604),.UNSPECIFIED.,.F.,.F.)
B_SPLINE_CURVE_WITH_KNOTS((3,2,2,2,2,2,2,2,3),(0.11,0.1125,0.115,0.1175,
0.12,0.1225,0.125,0.1275,0.13),.UNSPECIFIED.)
CURVE()
GEOMETRIC_REPRESENTATION_ITEM()
RATIONAL_B_SPLINE_CURVE((1.,0.923879532511287,1.,0.923879532511287,1.,0.923879532511287,
1.,0.923879532511287,1.,0.923879532511287,1.,0.923879532511287,1.,0.923879532511287,
1.,0.923879532511287,1.))
REPRESENTATION_ITEM('')
);
#660=(
BOUNDED_CURVE()
B_SPLINE_CURVE(2,(#5609,#5610,#5611,#5612,#5613,#5614,#5615,#5616,#5617,
#5618,#5619,#5620,#5621,#5622,#5623,#5624,#5625),.UNSPECIFIED.,.F.,.F.)
B_SPLINE_CURVE_WITH_KNOTS((3,2,2,2,2,2,2,2,3),(0.09,0.0925,0.095,0.0975,
0.1,0.1025,0.105,0.1075,0.11),.UNSPECIFIED.)
CURVE()
GEOMETRIC_REPRESENTATION_ITEM()
RATIONAL_B_SPLINE_CURVE((1.,0.923879532511287,1.,0.923879532511287,1.,0.923879532511287,
1.,0.923879532511287,1.,0.923879532511287,1.,0.923879532511287,1.,0.923879532511287,
1.,0.923879532511287,1.))
REPRESENTATION_ITEM('')
);
#661=(
BOUNDED_CURVE()
B_SPLINE_CURVE(2,(#5626,#5627,#5628,#5629,#5630,#5631,#5632,#5633,#5634,
#5635,#5636,#5637,#5638,#5639,#5640,#5641,#5642),.UNSPECIFIED.,.F.,.F.)
B_SPLINE_CURVE_WITH_KNOTS((3,2,2,2,2,2,2,2,3),(0.09,0.0925,0.095,0.0975,
0.1,0.1025,0.105,0.1075,0.11),.UNSPECIFIED.)
CURVE()
GEOMETRIC_REPRESENTATION_ITEM()
RATIONAL_B_SPLINE_CURVE((1.,0.923879532511287,1.,0.923879532511287,1.,0.923879532511287,
1.,0.923879532511287,1.,0.923879532511287,1.,0.923879532511287,1.,0.923879532511287,
1.,0.923879532511287,1.))
REPRESENTATION_ITEM('')
);
#662=(
BOUNDED_CURVE()
B_SPLINE_CURVE(2,(#5647,#5648,#5649,#5650,#5651,#5652,#5653,#5654,#5655,
#5656,#5657,#5658,#5659,#5660,#5661,#5662,#5663),.UNSPECIFIED.,.F.,.F.)
B_SPLINE_CURVE_WITH_KNOTS((3,2,2,2,2,2,2,2,3),(0.07,0.0725,0.075,0.0775,
0.08,0.0825,0.085,0.0875,0.09),.UNSPECIFIED.)
CURVE()
GEOMETRIC_REPRESENTATION_ITEM()
RATIONAL_B_SPLINE_CURVE((1.,0.923879532511287,1.,0.923879532511287,1.,0.923879532511287,
1.,0.923879532511287,1.,0.923879532511287,1.,0.923879532511287,1.,0.923879532511287,
1.,0.923879532511287,1.))
REPRESENTATION_ITEM('')
);
#663=(
BOUNDED_CURVE()
B_SPLINE_CURVE(2,(#5664,#5665,#5666,#5667,#5668,#5669,#5670,#5671,#5672,
#5673,#5674,#5675,#5676,#5677,#5678,#5679,#5680),.UNSPECIFIED.,.F.,.F.)
B_SPLINE_CURVE_WITH_KNOTS((3,2,2,2,2,2,2,2,3),(0.07,0.0725,0.075,0.0775,
0.08,0.0825,0.085,0.0875,0.09),.UNSPECIFIED.)
CURVE()
GEOMETRIC_REPRESENTATION_ITEM()
RATIONAL_B_SPLINE_CURVE((1.,0.923879532511287,1.,0.923879532511287,1.,0.923879532511287,
1.,0.923879532511287,1.,0.923879532511287,1.,0.923879532511287,1.,0.923879532511287,
1.,0.923879532511287,1.))
REPRESENTATION_ITEM('')
);
#664=(
BOUNDED_CURVE()
B_SPLINE_CURVE(2,(#5685,#5686,#5687,#5688,#5689,#5690,#5691,#5692,#5693,
#5694,#5695,#5696,#5697,#5698,#5699,#5700,#5701),.UNSPECIFIED.,.F.,.F.)
B_SPLINE_CURVE_WITH_KNOTS((3,2,2,2,2,2,2,2,3),(0.05,0.0525,0.055,0.0575,
0.06,0.0625,0.065,0.0675,0.07),.UNSPECIFIED.)
CURVE()
GEOMETRIC_REPRESENTATION_ITEM()
RATIONAL_B_SPLINE_CURVE((1.,0.923879532511287,1.,0.923879532511287,1.,0.923879532511287,
1.,0.923879532511287,1.,0.923879532511287,1.,0.923879532511287,1.,0.923879532511287,
1.,0.923879532511287,1.))
REPRESENTATION_ITEM('')
);
#665=(
BOUNDED_CURVE()
B_SPLINE_CURVE(2,(#5702,#5703,#5704,#5705,#5706,#5707,#5708,#5709,#5710,
#5711,#5712,#5713,#5714,#5715,#5716,#5717,#5718),.UNSPECIFIED.,.F.,.F.)
B_SPLINE_CURVE_WITH_KNOTS((3,2,2,2,2,2,2,2,3),(0.05,0.0525,0.055,0.0575,
0.06,0.0625,0.065,0.0675,0.07),.UNSPECIFIED.)
CURVE()
GEOMETRIC_REPRESENTATION_ITEM()
RATIONAL_B_SPLINE_CURVE((1.,0.923879532511287,1.,0.923879532511287,1.,0.923879532511287,
1.,0.923879532511287,1.,0.923879532511287,1.,0.923879532511287,1.,0.923879532511287,
1.,0.923879532511287,1.))
REPRESENTATION_ITEM('')
);
#666=(
BOUNDED_CURVE()
B_SPLINE_CURVE(2,(#5723,#5724,#5725,#5726,#5727,#5728,#5729,#5730,#5731,
#5732,#5733,#5734,#5735,#5736,#5737,#5738,#5739),.UNSPECIFIED.,.F.,.F.)
B_SPLINE_CURVE_WITH_KNOTS((3,2,2,2,2,2,2,2,3),(0.03,0.0325,0.035,0.0375,
0.04,0.0425,0.045,0.0475,0.05),.UNSPECIFIED.)
CURVE()
GEOMETRIC_REPRESENTATION_ITEM()
RATIONAL_B_SPLINE_CURVE((1.,0.923879532511287,1.,0.923879532511287,1.,0.923879532511287,
1.,0.923879532511287,1.,0.923879532511287,1.,0.923879532511287,1.,0.923879532511287,
1.,0.923879532511287,1.))
REPRESENTATION_ITEM('')
);
#667=(
BOUNDED_CURVE()
B_SPLINE_CURVE(2,(#5740,#5741,#5742,#5743,#5744,#5745,#5746,#5747,#5748,
#5749,#5750,#5751,#5752,#5753,#5754,#5755,#5756),.UNSPECIFIED.,.F.,.F.)
B_SPLINE_CURVE_WITH_KNOTS((3,2,2,2,2,2,2,2,3),(0.03,0.0325,0.035,0.0375,
0.04,0.0425,0.045,0.0475,0.05),.UNSPECIFIED.)
CURVE()
GEOMETRIC_REPRESENTATION_ITEM()
RATIONAL_B_SPLINE_CURVE((1.,0.923879532511287,1.,0.923879532511287,1.,0.923879532511287,
1.,0.923879532511287,1.,0.923879532511287,1.,0.923879532511287,1.,0.923879532511287,
1.,0.923879532511287,1.))
REPRESENTATION_ITEM('')
);
#668=(
BOUNDED_CURVE()
B_SPLINE_CURVE(2,(#5762,#5763,#5764,#5765,#5766,#5767,#5768,#5769,#5770),
 .UNSPECIFIED.,.F.,.F.)
B_SPLINE_CURVE_WITH_KNOTS((3,2,2,2,3),(0.,0.0025,0.005,0.0075,0.01),
 .UNSPECIFIED.)
CURVE()
GEOMETRIC_REPRESENTATION_ITEM()
RATIONAL_B_SPLINE_CURVE((1.,0.923879532511287,1.,0.923879532511287,1.,0.923879532511287,
1.,0.923879532511287,1.))
REPRESENTATION_ITEM('')
);
#669=(
BOUNDED_CURVE()
B_SPLINE_CURVE(2,(#5773,#5774,#5775,#5776,#5777,#5778,#5779,#5780,#5781),
 .UNSPECIFIED.,.F.,.F.)
B_SPLINE_CURVE_WITH_KNOTS((3,2,2,2,3),(0.,0.0025,0.005,0.0075,0.01),
 .UNSPECIFIED.)
CURVE()
GEOMETRIC_REPRESENTATION_ITEM()
RATIONAL_B_SPLINE_CURVE((1.,0.923879532511287,1.,0.923879532511287,1.,0.923879532511287,
1.,0.923879532511287,1.))
REPRESENTATION_ITEM('')
);
#670=(
BOUNDED_CURVE()
B_SPLINE_CURVE(2,(#5787,#5788,#5789,#5790,#5791),.UNSPECIFIED.,.F.,.F.)
B_SPLINE_CURVE_WITH_KNOTS((3,2,3),(0.995,0.9975,1.),.UNSPECIFIED.)
CURVE()
GEOMETRIC_REPRESENTATION_ITEM()
RATIONAL_B_SPLINE_CURVE((1.,0.923879532511287,1.,0.923879532511287,1.))
REPRESENTATION_ITEM('')
);
#671=(
BOUNDED_CURVE()
B_SPLINE_CURVE(2,(#5794,#5795,#5796,#5797,#5798,#5799,#5800),
 .UNSPECIFIED.,.F.,.F.)
B_SPLINE_CURVE_WITH_KNOTS((3,2,2,3),(0.975,0.9775,0.98,0.9825),
 .UNSPECIFIED.)
CURVE()
GEOMETRIC_REPRESENTATION_ITEM()
RATIONAL_B_SPLINE_CURVE((1.,0.923879532511287,1.,0.923879532511287,1.,0.923879532511287,
1.))
REPRESENTATION_ITEM('')
);
#672=(
BOUNDED_CURVE()
B_SPLINE_CURVE(2,(#5805,#5806,#5807,#5808,#5809,#5810,#5811,#5812,#5813,
#5814,#5815,#5816,#5817,#5818,#5819,#5820,#5821),.UNSPECIFIED.,.F.,.F.)
B_SPLINE_CURVE_WITH_KNOTS((3,2,2,2,2,2,2,2,3),(0.975,0.9775,0.98,0.9825,
0.985,0.9875,0.99,0.9925,0.995),.UNSPECIFIED.)
CURVE()
GEOMETRIC_REPRESENTATION_ITEM()
RATIONAL_B_SPLINE_CURVE((1.,0.923879532511287,1.,0.923879532511287,1.,0.923879532511287,
1.,0.923879532511287,1.,0.923879532511287,1.,0.923879532511287,1.,0.923879532511287,
1.,0.923879532511287,1.))
REPRESENTATION_ITEM('')
);
#673=(
BOUNDED_CURVE()
B_SPLINE_CURVE(2,(#5822,#5823,#5824,#5825,#5826,#5827,#5828,#5829,#5830,
#5831,#5832,#5833,#5834,#5835,#5836,#5837,#5838),.UNSPECIFIED.,.F.,.F.)
B_SPLINE_CURVE_WITH_KNOTS((3,2,2,2,2,2,2,2,3),(0.955,0.9575,0.96,0.9625,
0.965,0.9675,0.97,0.9725,0.975),.UNSPECIFIED.)
CURVE()
GEOMETRIC_REPRESENTATION_ITEM()
RATIONAL_B_SPLINE_CURVE((1.,0.923879532511287,1.,0.923879532511287,1.,0.923879532511287,
1.,0.923879532511287,1.,0.923879532511287,1.,0.923879532511287,1.,0.923879532511287,
1.,0.923879532511287,1.))
REPRESENTATION_ITEM('')
);
#674=(
BOUNDED_CURVE()
B_SPLINE_CURVE(2,(#5843,#5844,#5845,#5846,#5847,#5848,#5849,#5850,#5851,
#5852,#5853,#5854,#5855,#5856,#5857,#5858,#5859),.UNSPECIFIED.,.F.,.F.)
B_SPLINE_CURVE_WITH_KNOTS((3,2,2,2,2,2,2,2,3),(0.955,0.9575,0.96,0.9625,
0.965,0.9675,0.97,0.9725,0.975),.UNSPECIFIED.)
CURVE()
GEOMETRIC_REPRESENTATION_ITEM()
RATIONAL_B_SPLINE_CURVE((1.,0.923879532511287,1.,0.923879532511287,1.,0.923879532511287,
1.,0.923879532511287,1.,0.923879532511287,1.,0.923879532511287,1.,0.923879532511287,
1.,0.923879532511287,1.))
REPRESENTATION_ITEM('')
);
#675=(
BOUNDED_CURVE()
B_SPLINE_CURVE(2,(#5860,#5861,#5862,#5863,#5864,#5865,#5866,#5867,#5868,
#5869,#5870,#5871,#5872,#5873,#5874,#5875,#5876),.UNSPECIFIED.,.F.,.F.)
B_SPLINE_CURVE_WITH_KNOTS((3,2,2,2,2,2,2,2,3),(0.935,0.9375,0.94,0.9425,
0.945,0.9475,0.95,0.9525,0.955),.UNSPECIFIED.)
CURVE()
GEOMETRIC_REPRESENTATION_ITEM()
RATIONAL_B_SPLINE_CURVE((1.,0.923879532511287,1.,0.923879532511287,1.,0.923879532511287,
1.,0.923879532511287,1.,0.923879532511287,1.,0.923879532511287,1.,0.923879532511287,
1.,0.923879532511287,1.))
REPRESENTATION_ITEM('')
);
#676=(
BOUNDED_CURVE()
B_SPLINE_CURVE(2,(#5881,#5882,#5883,#5884,#5885,#5886,#5887,#5888,#5889,
#5890,#5891,#5892,#5893,#5894,#5895,#5896,#5897),.UNSPECIFIED.,.F.,.F.)
B_SPLINE_CURVE_WITH_KNOTS((3,2,2,2,2,2,2,2,3),(0.935,0.9375,0.94,0.9425,
0.945,0.9475,0.95,0.9525,0.955),.UNSPECIFIED.)
CURVE()
GEOMETRIC_REPRESENTATION_ITEM()
RATIONAL_B_SPLINE_CURVE((1.,0.923879532511287,1.,0.923879532511287,1.,0.923879532511287,
1.,0.923879532511287,1.,0.923879532511287,1.,0.923879532511287,1.,0.923879532511287,
1.,0.923879532511287,1.))
REPRESENTATION_ITEM('')
);
#677=(
BOUNDED_CURVE()
B_SPLINE_CURVE(2,(#5898,#5899,#5900,#5901,#5902,#5903,#5904,#5905,#5906,
#5907,#5908,#5909,#5910,#5911,#5912,#5913,#5914),.UNSPECIFIED.,.F.,.F.)
B_SPLINE_CURVE_WITH_KNOTS((3,2,2,2,2,2,2,2,3),(0.915,0.9175,0.92,0.9225,
0.925,0.9275,0.93,0.9325,0.935),.UNSPECIFIED.)
CURVE()
GEOMETRIC_REPRESENTATION_ITEM()
RATIONAL_B_SPLINE_CURVE((1.,0.923879532511287,1.,0.923879532511287,1.,0.923879532511287,
1.,0.923879532511287,1.,0.923879532511287,1.,0.923879532511287,1.,0.923879532511287,
1.,0.923879532511287,1.))
REPRESENTATION_ITEM('')
);
#678=(
BOUNDED_CURVE()
B_SPLINE_CURVE(2,(#5919,#5920,#5921,#5922,#5923,#5924,#5925,#5926,#5927,
#5928,#5929,#5930,#5931,#5932,#5933,#5934,#5935),.UNSPECIFIED.,.F.,.F.)
B_SPLINE_CURVE_WITH_KNOTS((3,2,2,2,2,2,2,2,3),(0.915,0.9175,0.92,0.9225,
0.925,0.9275,0.93,0.9325,0.935),.UNSPECIFIED.)
CURVE()
GEOMETRIC_REPRESENTATION_ITEM()
RATIONAL_B_SPLINE_CURVE((1.,0.923879532511287,1.,0.923879532511287,1.,0.923879532511287,
1.,0.923879532511287,1.,0.923879532511287,1.,0.923879532511287,1.,0.923879532511287,
1.,0.923879532511287,1.))
REPRESENTATION_ITEM('')
);
#679=(
BOUNDED_CURVE()
B_SPLINE_CURVE(2,(#5936,#5937,#5938,#5939,#5940,#5941,#5942,#5943,#5944,
#5945,#5946,#5947,#5948,#5949,#5950,#5951,#5952),.UNSPECIFIED.,.F.,.F.)
B_SPLINE_CURVE_WITH_KNOTS((3,2,2,2,2,2,2,2,3),(0.895,0.8975,0.9,0.9025,
0.905,0.9075,0.91,0.9125,0.915),.UNSPECIFIED.)
CURVE()
GEOMETRIC_REPRESENTATION_ITEM()
RATIONAL_B_SPLINE_CURVE((1.,0.923879532511287,1.,0.923879532511287,1.,0.923879532511287,
1.,0.923879532511287,1.,0.923879532511287,1.,0.923879532511287,1.,0.923879532511287,
1.,0.923879532511287,1.))
REPRESENTATION_ITEM('')
);
#680=(
BOUNDED_CURVE()
B_SPLINE_CURVE(2,(#5957,#5958,#5959,#5960,#5961,#5962,#5963,#5964,#5965,
#5966,#5967,#5968,#5969,#5970,#5971,#5972,#5973),.UNSPECIFIED.,.F.,.F.)
B_SPLINE_CURVE_WITH_KNOTS((3,2,2,2,2,2,2,2,3),(0.895,0.8975,0.9,0.9025,
0.905,0.9075,0.91,0.9125,0.915),.UNSPECIFIED.)
CURVE()
GEOMETRIC_REPRESENTATION_ITEM()
RATIONAL_B_SPLINE_CURVE((1.,0.923879532511287,1.,0.923879532511287,1.,0.923879532511287,
1.,0.923879532511287,1.,0.923879532511287,1.,0.923879532511287,1.,0.923879532511287,
1.,0.923879532511287,1.))
REPRESENTATION_ITEM('')
);
#681=(
BOUNDED_CURVE()
B_SPLINE_CURVE(2,(#5974,#5975,#5976,#5977,#5978,#5979,#5980,#5981,#5982,
#5983,#5984,#5985,#5986,#5987,#5988,#5989,#5990),.UNSPECIFIED.,.F.,.F.)
B_SPLINE_CURVE_WITH_KNOTS((3,2,2,2,2,2,2,2,3),(0.875,0.8775,0.88,0.8825,
0.885,0.8875,0.89,0.8925,0.895),.UNSPECIFIED.)
CURVE()
GEOMETRIC_REPRESENTATION_ITEM()
RATIONAL_B_SPLINE_CURVE((1.,0.923879532511287,1.,0.923879532511287,1.,0.923879532511287,
1.,0.923879532511287,1.,0.923879532511287,1.,0.923879532511287,1.,0.923879532511287,
1.,0.923879532511287,1.))
REPRESENTATION_ITEM('')
);
#682=(
BOUNDED_CURVE()
B_SPLINE_CURVE(2,(#5995,#5996,#5997,#5998,#5999,#6000,#6001,#6002,#6003,
#6004,#6005,#6006,#6007,#6008,#6009,#6010,#6011),.UNSPECIFIED.,.F.,.F.)
B_SPLINE_CURVE_WITH_KNOTS((3,2,2,2,2,2,2,2,3),(0.875,0.8775,0.88,0.8825,
0.885,0.8875,0.89,0.8925,0.895),.UNSPECIFIED.)
CURVE()
GEOMETRIC_REPRESENTATION_ITEM()
RATIONAL_B_SPLINE_CURVE((1.,0.923879532511287,1.,0.923879532511287,1.,0.923879532511287,
1.,0.923879532511287,1.,0.923879532511287,1.,0.923879532511287,1.,0.923879532511287,
1.,0.923879532511287,1.))
REPRESENTATION_ITEM('')
);
#683=(
BOUNDED_CURVE()
B_SPLINE_CURVE(2,(#6012,#6013,#6014,#6015,#6016,#6017,#6018,#6019,#6020,
#6021,#6022,#6023,#6024,#6025,#6026,#6027,#6028),.UNSPECIFIED.,.F.,.F.)
B_SPLINE_CURVE_WITH_KNOTS((3,2,2,2,2,2,2,2,3),(0.855,0.8575,0.86,0.8625,
0.865,0.8675,0.87,0.8725,0.875),.UNSPECIFIED.)
CURVE()
GEOMETRIC_REPRESENTATION_ITEM()
RATIONAL_B_SPLINE_CURVE((1.,0.923879532511287,1.,0.923879532511287,1.,0.923879532511287,
1.,0.923879532511287,1.,0.923879532511287,1.,0.923879532511287,1.,0.923879532511287,
1.,0.923879532511287,1.))
REPRESENTATION_ITEM('')
);
#684=(
BOUNDED_CURVE()
B_SPLINE_CURVE(2,(#6033,#6034,#6035,#6036,#6037,#6038,#6039,#6040,#6041,
#6042,#6043,#6044,#6045,#6046,#6047,#6048,#6049),.UNSPECIFIED.,.F.,.F.)
B_SPLINE_CURVE_WITH_KNOTS((3,2,2,2,2,2,2,2,3),(0.855,0.8575,0.86,0.8625,
0.865,0.8675,0.87,0.8725,0.875),.UNSPECIFIED.)
CURVE()
GEOMETRIC_REPRESENTATION_ITEM()
RATIONAL_B_SPLINE_CURVE((1.,0.923879532511287,1.,0.923879532511287,1.,0.923879532511287,
1.,0.923879532511287,1.,0.923879532511287,1.,0.923879532511287,1.,0.923879532511287,
1.,0.923879532511287,1.))
REPRESENTATION_ITEM('')
);
#685=(
BOUNDED_CURVE()
B_SPLINE_CURVE(2,(#6050,#6051,#6052,#6053,#6054,#6055,#6056,#6057,#6058,
#6059,#6060,#6061,#6062,#6063,#6064,#6065,#6066),.UNSPECIFIED.,.F.,.F.)
B_SPLINE_CURVE_WITH_KNOTS((3,2,2,2,2,2,2,2,3),(0.835,0.8375,0.84,0.8425,
0.845,0.8475,0.85,0.8525,0.855),.UNSPECIFIED.)
CURVE()
GEOMETRIC_REPRESENTATION_ITEM()
RATIONAL_B_SPLINE_CURVE((1.,0.923879532511287,1.,0.923879532511287,1.,0.923879532511287,
1.,0.923879532511287,1.,0.923879532511287,1.,0.923879532511287,1.,0.923879532511287,
1.,0.923879532511287,1.))
REPRESENTATION_ITEM('')
);
#686=(
BOUNDED_CURVE()
B_SPLINE_CURVE(2,(#6071,#6072,#6073,#6074,#6075,#6076,#6077,#6078,#6079,
#6080,#6081,#6082,#6083,#6084,#6085,#6086,#6087),.UNSPECIFIED.,.F.,.F.)
B_SPLINE_CURVE_WITH_KNOTS((3,2,2,2,2,2,2,2,3),(0.835,0.8375,0.84,0.8425,
0.845,0.8475,0.85,0.8525,0.855),.UNSPECIFIED.)
CURVE()
GEOMETRIC_REPRESENTATION_ITEM()
RATIONAL_B_SPLINE_CURVE((1.,0.923879532511287,1.,0.923879532511287,1.,0.923879532511287,
1.,0.923879532511287,1.,0.923879532511287,1.,0.923879532511287,1.,0.923879532511287,
1.,0.923879532511287,1.))
REPRESENTATION_ITEM('')
);
#687=(
BOUNDED_CURVE()
B_SPLINE_CURVE(2,(#6088,#6089,#6090,#6091,#6092,#6093,#6094,#6095,#6096,
#6097,#6098,#6099,#6100,#6101,#6102,#6103,#6104),.UNSPECIFIED.,.F.,.F.)
B_SPLINE_CURVE_WITH_KNOTS((3,2,2,2,2,2,2,2,3),(0.815,0.8175,0.82,0.8225,
0.825,0.8275,0.83,0.8325,0.835),.UNSPECIFIED.)
CURVE()
GEOMETRIC_REPRESENTATION_ITEM()
RATIONAL_B_SPLINE_CURVE((1.,0.923879532511287,1.,0.923879532511287,1.,0.923879532511287,
1.,0.923879532511287,1.,0.923879532511287,1.,0.923879532511287,1.,0.923879532511287,
1.,0.923879532511287,1.))
REPRESENTATION_ITEM('')
);
#688=(
BOUNDED_CURVE()
B_SPLINE_CURVE(2,(#6109,#6110,#6111,#6112,#6113,#6114,#6115,#6116,#6117,
#6118,#6119,#6120,#6121,#6122,#6123,#6124,#6125),.UNSPECIFIED.,.F.,.F.)
B_SPLINE_CURVE_WITH_KNOTS((3,2,2,2,2,2,2,2,3),(0.815,0.8175,0.82,0.8225,
0.825,0.8275,0.83,0.8325,0.835),.UNSPECIFIED.)
CURVE()
GEOMETRIC_REPRESENTATION_ITEM()
RATIONAL_B_SPLINE_CURVE((1.,0.923879532511287,1.,0.923879532511287,1.,0.923879532511287,
1.,0.923879532511287,1.,0.923879532511287,1.,0.923879532511287,1.,0.923879532511287,
1.,0.923879532511287,1.))
REPRESENTATION_ITEM('')
);
#689=(
BOUNDED_CURVE()
B_SPLINE_CURVE(2,(#6126,#6127,#6128,#6129,#6130,#6131,#6132,#6133,#6134,
#6135,#6136,#6137,#6138,#6139,#6140,#6141,#6142),.UNSPECIFIED.,.F.,.F.)
B_SPLINE_CURVE_WITH_KNOTS((3,2,2,2,2,2,2,2,3),(0.795,0.7975,0.8,0.8025,
0.805,0.8075,0.81,0.8125,0.815),.UNSPECIFIED.)
CURVE()
GEOMETRIC_REPRESENTATION_ITEM()
RATIONAL_B_SPLINE_CURVE((1.,0.923879532511287,1.,0.923879532511287,1.,0.923879532511287,
1.,0.923879532511287,1.,0.923879532511287,1.,0.923879532511287,1.,0.923879532511287,
1.,0.923879532511287,1.))
REPRESENTATION_ITEM('')
);
#690=(
BOUNDED_CURVE()
B_SPLINE_CURVE(2,(#6147,#6148,#6149,#6150,#6151,#6152,#6153,#6154,#6155,
#6156,#6157,#6158,#6159,#6160,#6161,#6162,#6163),.UNSPECIFIED.,.F.,.F.)
B_SPLINE_CURVE_WITH_KNOTS((3,2,2,2,2,2,2,2,3),(0.795,0.7975,0.8,0.8025,
0.805,0.8075,0.81,0.8125,0.815),.UNSPECIFIED.)
CURVE()
GEOMETRIC_REPRESENTATION_ITEM()
RATIONAL_B_SPLINE_CURVE((1.,0.923879532511287,1.,0.923879532511287,1.,0.923879532511287,
1.,0.923879532511287,1.,0.923879532511287,1.,0.923879532511287,1.,0.923879532511287,
1.,0.923879532511287,1.))
REPRESENTATION_ITEM('')
);
#691=(
BOUNDED_CURVE()
B_SPLINE_CURVE(2,(#6164,#6165,#6166,#6167,#6168,#6169,#6170,#6171,#6172,
#6173,#6174,#6175,#6176,#6177,#6178,#6179,#6180),.UNSPECIFIED.,.F.,.F.)
B_SPLINE_CURVE_WITH_KNOTS((3,2,2,2,2,2,2,2,3),(0.775,0.7775,0.78,0.7825,
0.785,0.7875,0.79,0.7925,0.795),.UNSPECIFIED.)
CURVE()
GEOMETRIC_REPRESENTATION_ITEM()
RATIONAL_B_SPLINE_CURVE((1.,0.923879532511287,1.,0.923879532511287,1.,0.923879532511287,
1.,0.923879532511287,1.,0.923879532511287,1.,0.923879532511287,1.,0.923879532511287,
1.,0.923879532511287,1.))
REPRESENTATION_ITEM('')
);
#692=(
BOUNDED_CURVE()
B_SPLINE_CURVE(2,(#6185,#6186,#6187,#6188,#6189,#6190,#6191,#6192,#6193,
#6194,#6195,#6196,#6197,#6198,#6199,#6200,#6201),.UNSPECIFIED.,.F.,.F.)
B_SPLINE_CURVE_WITH_KNOTS((3,2,2,2,2,2,2,2,3),(0.775,0.7775,0.78,0.7825,
0.785,0.7875,0.79,0.7925,0.795),.UNSPECIFIED.)
CURVE()
GEOMETRIC_REPRESENTATION_ITEM()
RATIONAL_B_SPLINE_CURVE((1.,0.923879532511287,1.,0.923879532511287,1.,0.923879532511287,
1.,0.923879532511287,1.,0.923879532511287,1.,0.923879532511287,1.,0.923879532511287,
1.,0.923879532511287,1.))
REPRESENTATION_ITEM('')
);
#693=(
BOUNDED_CURVE()
B_SPLINE_CURVE(2,(#6202,#6203,#6204,#6205,#6206,#6207,#6208,#6209,#6210,
#6211,#6212,#6213,#6214,#6215,#6216,#6217,#6218),.UNSPECIFIED.,.F.,.F.)
B_SPLINE_CURVE_WITH_KNOTS((3,2,2,2,2,2,2,2,3),(0.755,0.7575,0.76,0.7625,
0.765,0.7675,0.77,0.7725,0.775),.UNSPECIFIED.)
CURVE()
GEOMETRIC_REPRESENTATION_ITEM()
RATIONAL_B_SPLINE_CURVE((1.,0.923879532511287,1.,0.923879532511287,1.,0.923879532511287,
1.,0.923879532511287,1.,0.923879532511287,1.,0.923879532511287,1.,0.923879532511287,
1.,0.923879532511287,1.))
REPRESENTATION_ITEM('')
);
#694=(
BOUNDED_CURVE()
B_SPLINE_CURVE(2,(#6223,#6224,#6225,#6226,#6227,#6228,#6229,#6230,#6231,
#6232,#6233,#6234,#6235,#6236,#6237,#6238,#6239),.UNSPECIFIED.,.F.,.F.)
B_SPLINE_CURVE_WITH_KNOTS((3,2,2,2,2,2,2,2,3),(0.755,0.7575,0.76,0.7625,
0.765,0.7675,0.77,0.7725,0.775),.UNSPECIFIED.)
CURVE()
GEOMETRIC_REPRESENTATION_ITEM()
RATIONAL_B_SPLINE_CURVE((1.,0.923879532511287,1.,0.923879532511287,1.,0.923879532511287,
1.,0.923879532511287,1.,0.923879532511287,1.,0.923879532511287,1.,0.923879532511287,
1.,0.923879532511287,1.))
REPRESENTATION_ITEM('')
);
#695=(
BOUNDED_CURVE()
B_SPLINE_CURVE(2,(#6240,#6241,#6242,#6243,#6244,#6245,#6246,#6247,#6248,
#6249,#6250,#6251,#6252,#6253,#6254,#6255,#6256),.UNSPECIFIED.,.F.,.F.)
B_SPLINE_CURVE_WITH_KNOTS((3,2,2,2,2,2,2,2,3),(0.735,0.7375,0.74,0.7425,
0.745,0.7475,0.75,0.7525,0.755),.UNSPECIFIED.)
CURVE()
GEOMETRIC_REPRESENTATION_ITEM()
RATIONAL_B_SPLINE_CURVE((1.,0.923879532511287,1.,0.923879532511287,1.,0.923879532511287,
1.,0.923879532511287,1.,0.923879532511287,1.,0.923879532511287,1.,0.923879532511287,
1.,0.923879532511287,1.))
REPRESENTATION_ITEM('')
);
#696=(
BOUNDED_CURVE()
B_SPLINE_CURVE(2,(#6261,#6262,#6263,#6264,#6265,#6266,#6267,#6268,#6269,
#6270,#6271,#6272,#6273,#6274,#6275,#6276,#6277),.UNSPECIFIED.,.F.,.F.)
B_SPLINE_CURVE_WITH_KNOTS((3,2,2,2,2,2,2,2,3),(0.735,0.7375,0.74,0.7425,
0.745,0.7475,0.75,0.7525,0.755),.UNSPECIFIED.)
CURVE()
GEOMETRIC_REPRESENTATION_ITEM()
RATIONAL_B_SPLINE_CURVE((1.,0.923879532511287,1.,0.923879532511287,1.,0.923879532511287,
1.,0.923879532511287,1.,0.923879532511287,1.,0.923879532511287,1.,0.923879532511287,
1.,0.923879532511287,1.))
REPRESENTATION_ITEM('')
);
#697=(
BOUNDED_CURVE()
B_SPLINE_CURVE(2,(#6278,#6279,#6280,#6281,#6282,#6283,#6284,#6285,#6286,
#6287,#6288,#6289,#6290,#6291,#6292,#6293,#6294),.UNSPECIFIED.,.F.,.F.)
B_SPLINE_CURVE_WITH_KNOTS((3,2,2,2,2,2,2,2,3),(0.715,0.7175,0.72,0.7225,
0.725,0.7275,0.73,0.7325,0.735),.UNSPECIFIED.)
CURVE()
GEOMETRIC_REPRESENTATION_ITEM()
RATIONAL_B_SPLINE_CURVE((1.,0.923879532511287,1.,0.923879532511287,1.,0.923879532511287,
1.,0.923879532511287,1.,0.923879532511287,1.,0.923879532511287,1.,0.923879532511287,
1.,0.923879532511287,1.))
REPRESENTATION_ITEM('')
);
#698=(
BOUNDED_CURVE()
B_SPLINE_CURVE(2,(#6299,#6300,#6301,#6302,#6303,#6304,#6305,#6306,#6307,
#6308,#6309,#6310,#6311,#6312,#6313,#6314,#6315),.UNSPECIFIED.,.F.,.F.)
B_SPLINE_CURVE_WITH_KNOTS((3,2,2,2,2,2,2,2,3),(0.715,0.7175,0.72,0.7225,
0.725,0.7275,0.73,0.7325,0.735),.UNSPECIFIED.)
CURVE()
GEOMETRIC_REPRESENTATION_ITEM()
RATIONAL_B_SPLINE_CURVE((1.,0.923879532511287,1.,0.923879532511287,1.,0.923879532511287,
1.,0.923879532511287,1.,0.923879532511287,1.,0.923879532511287,1.,0.923879532511287,
1.,0.923879532511287,1.))
REPRESENTATION_ITEM('')
);
#699=(
BOUNDED_CURVE()
B_SPLINE_CURVE(2,(#6316,#6317,#6318,#6319,#6320,#6321,#6322,#6323,#6324,
#6325,#6326,#6327,#6328,#6329,#6330,#6331,#6332),.UNSPECIFIED.,.F.,.F.)
B_SPLINE_CURVE_WITH_KNOTS((3,2,2,2,2,2,2,2,3),(0.695,0.6975,0.7,0.7025,
0.705,0.7075,0.71,0.7125,0.715),.UNSPECIFIED.)
CURVE()
GEOMETRIC_REPRESENTATION_ITEM()
RATIONAL_B_SPLINE_CURVE((1.,0.923879532511287,1.,0.923879532511287,1.,0.923879532511287,
1.,0.923879532511287,1.,0.923879532511287,1.,0.923879532511287,1.,0.923879532511287,
1.,0.923879532511287,1.))
REPRESENTATION_ITEM('')
);
#700=(
BOUNDED_CURVE()
B_SPLINE_CURVE(2,(#6337,#6338,#6339,#6340,#6341,#6342,#6343,#6344,#6345,
#6346,#6347,#6348,#6349,#6350,#6351,#6352,#6353),.UNSPECIFIED.,.F.,.F.)
B_SPLINE_CURVE_WITH_KNOTS((3,2,2,2,2,2,2,2,3),(0.695,0.6975,0.7,0.7025,
0.705,0.7075,0.71,0.7125,0.715),.UNSPECIFIED.)
CURVE()
GEOMETRIC_REPRESENTATION_ITEM()
RATIONAL_B_SPLINE_CURVE((1.,0.923879532511287,1.,0.923879532511287,1.,0.923879532511287,
1.,0.923879532511287,1.,0.923879532511287,1.,0.923879532511287,1.,0.923879532511287,
1.,0.923879532511287,1.))
REPRESENTATION_ITEM('')
);
#701=(
BOUNDED_CURVE()
B_SPLINE_CURVE(2,(#6354,#6355,#6356,#6357,#6358,#6359,#6360,#6361,#6362,
#6363,#6364,#6365,#6366,#6367,#6368,#6369,#6370),.UNSPECIFIED.,.F.,.F.)
B_SPLINE_CURVE_WITH_KNOTS((3,2,2,2,2,2,2,2,3),(0.675,0.6775,0.68,0.6825,
0.685,0.6875,0.69,0.6925,0.695),.UNSPECIFIED.)
CURVE()
GEOMETRIC_REPRESENTATION_ITEM()
RATIONAL_B_SPLINE_CURVE((1.,0.923879532511287,1.,0.923879532511287,1.,0.923879532511287,
1.,0.923879532511287,1.,0.923879532511287,1.,0.923879532511287,1.,0.923879532511287,
1.,0.923879532511287,1.))
REPRESENTATION_ITEM('')
);
#702=(
BOUNDED_CURVE()
B_SPLINE_CURVE(2,(#6375,#6376,#6377,#6378,#6379,#6380,#6381,#6382,#6383,
#6384,#6385,#6386,#6387,#6388,#6389,#6390,#6391),.UNSPECIFIED.,.F.,.F.)
B_SPLINE_CURVE_WITH_KNOTS((3,2,2,2,2,2,2,2,3),(0.675,0.6775,0.68,0.6825,
0.685,0.6875,0.69,0.6925,0.695),.UNSPECIFIED.)
CURVE()
GEOMETRIC_REPRESENTATION_ITEM()
RATIONAL_B_SPLINE_CURVE((1.,0.923879532511287,1.,0.923879532511287,1.,0.923879532511287,
1.,0.923879532511287,1.,0.923879532511287,1.,0.923879532511287,1.,0.923879532511287,
1.,0.923879532511287,1.))
REPRESENTATION_ITEM('')
);
#703=(
BOUNDED_CURVE()
B_SPLINE_CURVE(2,(#6392,#6393,#6394,#6395,#6396,#6397,#6398,#6399,#6400,
#6401,#6402,#6403,#6404,#6405,#6406,#6407,#6408),.UNSPECIFIED.,.F.,.F.)
B_SPLINE_CURVE_WITH_KNOTS((3,2,2,2,2,2,2,2,3),(0.655,0.6575,0.66,0.6625,
0.665,0.6675,0.67,0.6725,0.675),.UNSPECIFIED.)
CURVE()
GEOMETRIC_REPRESENTATION_ITEM()
RATIONAL_B_SPLINE_CURVE((1.,0.923879532511287,1.,0.923879532511287,1.,0.923879532511287,
1.,0.923879532511287,1.,0.923879532511287,1.,0.923879532511287,1.,0.923879532511287,
1.,0.923879532511287,1.))
REPRESENTATION_ITEM('')
);
#704=(
BOUNDED_CURVE()
B_SPLINE_CURVE(2,(#6413,#6414,#6415,#6416,#6417,#6418,#6419,#6420,#6421,
#6422,#6423,#6424,#6425,#6426,#6427,#6428,#6429),.UNSPECIFIED.,.F.,.F.)
B_SPLINE_CURVE_WITH_KNOTS((3,2,2,2,2,2,2,2,3),(0.655,0.6575,0.66,0.6625,
0.665,0.6675,0.67,0.6725,0.675),.UNSPECIFIED.)
CURVE()
GEOMETRIC_REPRESENTATION_ITEM()
RATIONAL_B_SPLINE_CURVE((1.,0.923879532511287,1.,0.923879532511287,1.,0.923879532511287,
1.,0.923879532511287,1.,0.923879532511287,1.,0.923879532511287,1.,0.923879532511287,
1.,0.923879532511287,1.))
REPRESENTATION_ITEM('')
);
#705=(
BOUNDED_CURVE()
B_SPLINE_CURVE(2,(#6430,#6431,#6432,#6433,#6434,#6435,#6436,#6437,#6438,
#6439,#6440,#6441,#6442,#6443,#6444,#6445,#6446),.UNSPECIFIED.,.F.,.F.)
B_SPLINE_CURVE_WITH_KNOTS((3,2,2,2,2,2,2,2,3),(0.635,0.6375,0.64,0.6425,
0.645,0.6475,0.65,0.6525,0.655),.UNSPECIFIED.)
CURVE()
GEOMETRIC_REPRESENTATION_ITEM()
RATIONAL_B_SPLINE_CURVE((1.,0.923879532511287,1.,0.923879532511287,1.,0.923879532511287,
1.,0.923879532511287,1.,0.923879532511287,1.,0.923879532511287,1.,0.923879532511287,
1.,0.923879532511287,1.))
REPRESENTATION_ITEM('')
);
#706=(
BOUNDED_CURVE()
B_SPLINE_CURVE(2,(#6451,#6452,#6453,#6454,#6455,#6456,#6457,#6458,#6459,
#6460,#6461,#6462,#6463,#6464,#6465,#6466,#6467),.UNSPECIFIED.,.F.,.F.)
B_SPLINE_CURVE_WITH_KNOTS((3,2,2,2,2,2,2,2,3),(0.635,0.6375,0.64,0.6425,
0.645,0.6475,0.65,0.6525,0.655),.UNSPECIFIED.)
CURVE()
GEOMETRIC_REPRESENTATION_ITEM()
RATIONAL_B_SPLINE_CURVE((1.,0.923879532511287,1.,0.923879532511287,1.,0.923879532511287,
1.,0.923879532511287,1.,0.923879532511287,1.,0.923879532511287,1.,0.923879532511287,
1.,0.923879532511287,1.))
REPRESENTATION_ITEM('')
);
#707=(
BOUNDED_CURVE()
B_SPLINE_CURVE(2,(#6468,#6469,#6470,#6471,#6472,#6473,#6474,#6475,#6476,
#6477,#6478,#6479,#6480,#6481,#6482,#6483,#6484),.UNSPECIFIED.,.F.,.F.)
B_SPLINE_CURVE_WITH_KNOTS((3,2,2,2,2,2,2,2,3),(0.615,0.6175,0.62,0.6225,
0.625,0.6275,0.63,0.6325,0.635),.UNSPECIFIED.)
CURVE()
GEOMETRIC_REPRESENTATION_ITEM()
RATIONAL_B_SPLINE_CURVE((1.,0.923879532511287,1.,0.923879532511287,1.,0.923879532511287,
1.,0.923879532511287,1.,0.923879532511287,1.,0.923879532511287,1.,0.923879532511287,
1.,0.923879532511287,1.))
REPRESENTATION_ITEM('')
);
#708=(
BOUNDED_CURVE()
B_SPLINE_CURVE(2,(#6489,#6490,#6491,#6492,#6493,#6494,#6495,#6496,#6497,
#6498,#6499,#6500,#6501,#6502,#6503,#6504,#6505),.UNSPECIFIED.,.F.,.F.)
B_SPLINE_CURVE_WITH_KNOTS((3,2,2,2,2,2,2,2,3),(0.615,0.6175,0.62,0.6225,
0.625,0.6275,0.63,0.6325,0.635),.UNSPECIFIED.)
CURVE()
GEOMETRIC_REPRESENTATION_ITEM()
RATIONAL_B_SPLINE_CURVE((1.,0.923879532511287,1.,0.923879532511287,1.,0.923879532511287,
1.,0.923879532511287,1.,0.923879532511287,1.,0.923879532511287,1.,0.923879532511287,
1.,0.923879532511287,1.))
REPRESENTATION_ITEM('')
);
#709=(
BOUNDED_CURVE()
B_SPLINE_CURVE(2,(#6506,#6507,#6508,#6509,#6510,#6511,#6512,#6513,#6514,
#6515,#6516,#6517,#6518,#6519,#6520,#6521,#6522),.UNSPECIFIED.,.F.,.F.)
B_SPLINE_CURVE_WITH_KNOTS((3,2,2,2,2,2,2,2,3),(0.595,0.5975,0.6,0.6025,
0.605,0.6075,0.61,0.6125,0.615),.UNSPECIFIED.)
CURVE()
GEOMETRIC_REPRESENTATION_ITEM()
RATIONAL_B_SPLINE_CURVE((1.,0.923879532511287,1.,0.923879532511287,1.,0.923879532511287,
1.,0.923879532511287,1.,0.923879532511287,1.,0.923879532511287,1.,0.923879532511287,
1.,0.923879532511287,1.))
REPRESENTATION_ITEM('')
);
#710=(
BOUNDED_CURVE()
B_SPLINE_CURVE(2,(#6527,#6528,#6529,#6530,#6531,#6532,#6533,#6534,#6535,
#6536,#6537,#6538,#6539,#6540,#6541,#6542,#6543),.UNSPECIFIED.,.F.,.F.)
B_SPLINE_CURVE_WITH_KNOTS((3,2,2,2,2,2,2,2,3),(0.595,0.5975,0.6,0.6025,
0.605,0.6075,0.61,0.6125,0.615),.UNSPECIFIED.)
CURVE()
GEOMETRIC_REPRESENTATION_ITEM()
RATIONAL_B_SPLINE_CURVE((1.,0.923879532511287,1.,0.923879532511287,1.,0.923879532511287,
1.,0.923879532511287,1.,0.923879532511287,1.,0.923879532511287,1.,0.923879532511287,
1.,0.923879532511287,1.))
REPRESENTATION_ITEM('')
);
#711=(
BOUNDED_CURVE()
B_SPLINE_CURVE(2,(#6544,#6545,#6546,#6547,#6548,#6549,#6550,#6551,#6552,
#6553,#6554,#6555,#6556,#6557,#6558,#6559,#6560),.UNSPECIFIED.,.F.,.F.)
B_SPLINE_CURVE_WITH_KNOTS((3,2,2,2,2,2,2,2,3),(0.575,0.5775,0.58,0.5825,
0.585,0.5875,0.59,0.5925,0.595),.UNSPECIFIED.)
CURVE()
GEOMETRIC_REPRESENTATION_ITEM()
RATIONAL_B_SPLINE_CURVE((1.,0.923879532511287,1.,0.923879532511287,1.,0.923879532511287,
1.,0.923879532511287,1.,0.923879532511287,1.,0.923879532511287,1.,0.923879532511287,
1.,0.923879532511287,1.))
REPRESENTATION_ITEM('')
);
#712=(
BOUNDED_CURVE()
B_SPLINE_CURVE(2,(#6565,#6566,#6567,#6568,#6569,#6570,#6571,#6572,#6573,
#6574,#6575,#6576,#6577,#6578,#6579,#6580,#6581),.UNSPECIFIED.,.F.,.F.)
B_SPLINE_CURVE_WITH_KNOTS((3,2,2,2,2,2,2,2,3),(0.575,0.5775,0.58,0.5825,
0.585,0.5875,0.59,0.5925,0.595),.UNSPECIFIED.)
CURVE()
GEOMETRIC_REPRESENTATION_ITEM()
RATIONAL_B_SPLINE_CURVE((1.,0.923879532511287,1.,0.923879532511287,1.,0.923879532511287,
1.,0.923879532511287,1.,0.923879532511287,1.,0.923879532511287,1.,0.923879532511287,
1.,0.923879532511287,1.))
REPRESENTATION_ITEM('')
);
#713=(
BOUNDED_CURVE()
B_SPLINE_CURVE(2,(#6582,#6583,#6584,#6585,#6586,#6587,#6588,#6589,#6590,
#6591,#6592,#6593,#6594,#6595,#6596,#6597,#6598),.UNSPECIFIED.,.F.,.F.)
B_SPLINE_CURVE_WITH_KNOTS((3,2,2,2,2,2,2,2,3),(0.555,0.5575,0.56,0.5625,
0.565,0.5675,0.57,0.5725,0.575),.UNSPECIFIED.)
CURVE()
GEOMETRIC_REPRESENTATION_ITEM()
RATIONAL_B_SPLINE_CURVE((1.,0.923879532511287,1.,0.923879532511287,1.,0.923879532511287,
1.,0.923879532511287,1.,0.923879532511287,1.,0.923879532511287,1.,0.923879532511287,
1.,0.923879532511287,1.))
REPRESENTATION_ITEM('')
);
#714=(
BOUNDED_CURVE()
B_SPLINE_CURVE(2,(#6603,#6604,#6605,#6606,#6607,#6608,#6609,#6610,#6611,
#6612,#6613,#6614,#6615,#6616,#6617,#6618,#6619),.UNSPECIFIED.,.F.,.F.)
B_SPLINE_CURVE_WITH_KNOTS((3,2,2,2,2,2,2,2,3),(0.555,0.5575,0.56,0.5625,
0.565,0.5675,0.57,0.5725,0.575),.UNSPECIFIED.)
CURVE()
GEOMETRIC_REPRESENTATION_ITEM()
RATIONAL_B_SPLINE_CURVE((1.,0.923879532511287,1.,0.923879532511287,1.,0.923879532511287,
1.,0.923879532511287,1.,0.923879532511287,1.,0.923879532511287,1.,0.923879532511287,
1.,0.923879532511287,1.))
REPRESENTATION_ITEM('')
);
#715=(
BOUNDED_CURVE()
B_SPLINE_CURVE(2,(#6620,#6621,#6622,#6623,#6624,#6625,#6626,#6627,#6628,
#6629,#6630,#6631,#6632,#6633,#6634,#6635,#6636),.UNSPECIFIED.,.F.,.F.)
B_SPLINE_CURVE_WITH_KNOTS((3,2,2,2,2,2,2,2,3),(0.535,0.5375,0.54,0.5425,
0.545,0.5475,0.55,0.5525,0.555),.UNSPECIFIED.)
CURVE()
GEOMETRIC_REPRESENTATION_ITEM()
RATIONAL_B_SPLINE_CURVE((1.,0.923879532511287,1.,0.923879532511287,1.,0.923879532511287,
1.,0.923879532511287,1.,0.923879532511287,1.,0.923879532511287,1.,0.923879532511287,
1.,0.923879532511287,1.))
REPRESENTATION_ITEM('')
);
#716=(
BOUNDED_CURVE()
B_SPLINE_CURVE(2,(#6641,#6642,#6643,#6644,#6645,#6646,#6647,#6648,#6649,
#6650,#6651,#6652,#6653,#6654,#6655,#6656,#6657),.UNSPECIFIED.,.F.,.F.)
B_SPLINE_CURVE_WITH_KNOTS((3,2,2,2,2,2,2,2,3),(0.535,0.5375,0.54,0.5425,
0.545,0.5475,0.55,0.5525,0.555),.UNSPECIFIED.)
CURVE()
GEOMETRIC_REPRESENTATION_ITEM()
RATIONAL_B_SPLINE_CURVE((1.,0.923879532511287,1.,0.923879532511287,1.,0.923879532511287,
1.,0.923879532511287,1.,0.923879532511287,1.,0.923879532511287,1.,0.923879532511287,
1.,0.923879532511287,1.))
REPRESENTATION_ITEM('')
);
#717=(
BOUNDED_CURVE()
B_SPLINE_CURVE(2,(#6658,#6659,#6660,#6661,#6662,#6663,#6664,#6665,#6666,
#6667,#6668,#6669,#6670,#6671,#6672,#6673,#6674),.UNSPECIFIED.,.F.,.F.)
B_SPLINE_CURVE_WITH_KNOTS((3,2,2,2,2,2,2,2,3),(0.515,0.5175,0.52,0.5225,
0.525,0.5275,0.53,0.5325,0.535),.UNSPECIFIED.)
CURVE()
GEOMETRIC_REPRESENTATION_ITEM()
RATIONAL_B_SPLINE_CURVE((1.,0.923879532511287,1.,0.923879532511287,1.,0.923879532511287,
1.,0.923879532511287,1.,0.923879532511287,1.,0.923879532511287,1.,0.923879532511287,
1.,0.923879532511287,1.))
REPRESENTATION_ITEM('')
);
#718=(
BOUNDED_CURVE()
B_SPLINE_CURVE(2,(#6679,#6680,#6681,#6682,#6683,#6684,#6685,#6686,#6687,
#6688,#6689,#6690,#6691,#6692,#6693,#6694,#6695),.UNSPECIFIED.,.F.,.F.)
B_SPLINE_CURVE_WITH_KNOTS((3,2,2,2,2,2,2,2,3),(0.515,0.5175,0.52,0.5225,
0.525,0.5275,0.53,0.5325,0.535),.UNSPECIFIED.)
CURVE()
GEOMETRIC_REPRESENTATION_ITEM()
RATIONAL_B_SPLINE_CURVE((1.,0.923879532511287,1.,0.923879532511287,1.,0.923879532511287,
1.,0.923879532511287,1.,0.923879532511287,1.,0.923879532511287,1.,0.923879532511287,
1.,0.923879532511287,1.))
REPRESENTATION_ITEM('')
);
#719=(
BOUNDED_CURVE()
B_SPLINE_CURVE(2,(#6696,#6697,#6698,#6699,#6700,#6701,#6702,#6703,#6704,
#6705,#6706,#6707,#6708,#6709,#6710,#6711,#6712),.UNSPECIFIED.,.F.,.F.)
B_SPLINE_CURVE_WITH_KNOTS((3,2,2,2,2,2,2,2,3),(0.495,0.4975,0.5,0.5025,
0.505,0.5075,0.51,0.5125,0.515),.UNSPECIFIED.)
CURVE()
GEOMETRIC_REPRESENTATION_ITEM()
RATIONAL_B_SPLINE_CURVE((1.,0.923879532511287,1.,0.923879532511287,1.,0.923879532511287,
1.,0.923879532511287,1.,0.923879532511287,1.,0.923879532511287,1.,0.923879532511287,
1.,0.923879532511287,1.))
REPRESENTATION_ITEM('')
);
#720=(
BOUNDED_CURVE()
B_SPLINE_CURVE(2,(#6717,#6718,#6719,#6720,#6721,#6722,#6723,#6724,#6725,
#6726,#6727,#6728,#6729,#6730,#6731,#6732,#6733),.UNSPECIFIED.,.F.,.F.)
B_SPLINE_CURVE_WITH_KNOTS((3,2,2,2,2,2,2,2,3),(0.495,0.4975,0.5,0.5025,
0.505,0.5075,0.51,0.5125,0.515),.UNSPECIFIED.)
CURVE()
GEOMETRIC_REPRESENTATION_ITEM()
RATIONAL_B_SPLINE_CURVE((1.,0.923879532511287,1.,0.923879532511287,1.,0.923879532511287,
1.,0.923879532511287,1.,0.923879532511287,1.,0.923879532511287,1.,0.923879532511287,
1.,0.923879532511287,1.))
REPRESENTATION_ITEM('')
);
#721=(
BOUNDED_CURVE()
B_SPLINE_CURVE(2,(#6734,#6735,#6736,#6737,#6738,#6739,#6740,#6741,#6742,
#6743,#6744,#6745,#6746,#6747,#6748,#6749,#6750),.UNSPECIFIED.,.F.,.F.)
B_SPLINE_CURVE_WITH_KNOTS((3,2,2,2,2,2,2,2,3),(0.475,0.4775,0.48,0.4825,
0.485,0.4875,0.49,0.4925,0.495),.UNSPECIFIED.)
CURVE()
GEOMETRIC_REPRESENTATION_ITEM()
RATIONAL_B_SPLINE_CURVE((1.,0.923879532511287,1.,0.923879532511287,1.,0.923879532511287,
1.,0.923879532511287,1.,0.923879532511287,1.,0.923879532511287,1.,0.923879532511287,
1.,0.923879532511287,1.))
REPRESENTATION_ITEM('')
);
#722=(
BOUNDED_CURVE()
B_SPLINE_CURVE(2,(#6755,#6756,#6757,#6758,#6759,#6760,#6761,#6762,#6763,
#6764,#6765,#6766,#6767,#6768,#6769,#6770,#6771),.UNSPECIFIED.,.F.,.F.)
B_SPLINE_CURVE_WITH_KNOTS((3,2,2,2,2,2,2,2,3),(0.475,0.4775,0.48,0.4825,
0.485,0.4875,0.49,0.4925,0.495),.UNSPECIFIED.)
CURVE()
GEOMETRIC_REPRESENTATION_ITEM()
RATIONAL_B_SPLINE_CURVE((1.,0.923879532511287,1.,0.923879532511287,1.,0.923879532511287,
1.,0.923879532511287,1.,0.923879532511287,1.,0.923879532511287,1.,0.923879532511287,
1.,0.923879532511287,1.))
REPRESENTATION_ITEM('')
);
#723=(
BOUNDED_CURVE()
B_SPLINE_CURVE(2,(#6772,#6773,#6774,#6775,#6776,#6777,#6778,#6779,#6780,
#6781,#6782,#6783,#6784,#6785,#6786,#6787,#6788),.UNSPECIFIED.,.F.,.F.)
B_SPLINE_CURVE_WITH_KNOTS((3,2,2,2,2,2,2,2,3),(0.455,0.4575,0.46,0.4625,
0.465,0.4675,0.47,0.4725,0.475),.UNSPECIFIED.)
CURVE()
GEOMETRIC_REPRESENTATION_ITEM()
RATIONAL_B_SPLINE_CURVE((1.,0.923879532511287,1.,0.923879532511287,1.,0.923879532511287,
1.,0.923879532511287,1.,0.923879532511287,1.,0.923879532511287,1.,0.923879532511287,
1.,0.923879532511287,1.))
REPRESENTATION_ITEM('')
);
#724=(
BOUNDED_CURVE()
B_SPLINE_CURVE(2,(#6793,#6794,#6795,#6796,#6797,#6798,#6799,#6800,#6801,
#6802,#6803,#6804,#6805,#6806,#6807,#6808,#6809),.UNSPECIFIED.,.F.,.F.)
B_SPLINE_CURVE_WITH_KNOTS((3,2,2,2,2,2,2,2,3),(0.455,0.4575,0.46,0.4625,
0.465,0.4675,0.47,0.4725,0.475),.UNSPECIFIED.)
CURVE()
GEOMETRIC_REPRESENTATION_ITEM()
RATIONAL_B_SPLINE_CURVE((1.,0.923879532511287,1.,0.923879532511287,1.,0.923879532511287,
1.,0.923879532511287,1.,0.923879532511287,1.,0.923879532511287,1.,0.923879532511287,
1.,0.923879532511287,1.))
REPRESENTATION_ITEM('')
);
#725=(
BOUNDED_CURVE()
B_SPLINE_CURVE(2,(#6810,#6811,#6812,#6813,#6814,#6815,#6816,#6817,#6818,
#6819,#6820,#6821,#6822,#6823,#6824,#6825,#6826),.UNSPECIFIED.,.F.,.F.)
B_SPLINE_CURVE_WITH_KNOTS((3,2,2,2,2,2,2,2,3),(0.435,0.4375,0.44,0.4425,
0.445,0.4475,0.45,0.4525,0.455),.UNSPECIFIED.)
CURVE()
GEOMETRIC_REPRESENTATION_ITEM()
RATIONAL_B_SPLINE_CURVE((1.,0.923879532511287,1.,0.923879532511287,1.,0.923879532511287,
1.,0.923879532511287,1.,0.923879532511287,1.,0.923879532511287,1.,0.923879532511287,
1.,0.923879532511287,1.))
REPRESENTATION_ITEM('')
);
#726=(
BOUNDED_CURVE()
B_SPLINE_CURVE(2,(#6831,#6832,#6833,#6834,#6835,#6836,#6837,#6838,#6839,
#6840,#6841,#6842,#6843,#6844,#6845,#6846,#6847),.UNSPECIFIED.,.F.,.F.)
B_SPLINE_CURVE_WITH_KNOTS((3,2,2,2,2,2,2,2,3),(0.435,0.4375,0.44,0.4425,
0.445,0.4475,0.45,0.4525,0.455),.UNSPECIFIED.)
CURVE()
GEOMETRIC_REPRESENTATION_ITEM()
RATIONAL_B_SPLINE_CURVE((1.,0.923879532511287,1.,0.923879532511287,1.,0.923879532511287,
1.,0.923879532511287,1.,0.923879532511287,1.,0.923879532511287,1.,0.923879532511287,
1.,0.923879532511287,1.))
REPRESENTATION_ITEM('')
);
#727=(
BOUNDED_CURVE()
B_SPLINE_CURVE(2,(#6848,#6849,#6850,#6851,#6852,#6853,#6854,#6855,#6856,
#6857,#6858,#6859,#6860,#6861,#6862,#6863,#6864),.UNSPECIFIED.,.F.,.F.)
B_SPLINE_CURVE_WITH_KNOTS((3,2,2,2,2,2,2,2,3),(0.415,0.4175,0.42,0.4225,
0.425,0.4275,0.43,0.4325,0.435),.UNSPECIFIED.)
CURVE()
GEOMETRIC_REPRESENTATION_ITEM()
RATIONAL_B_SPLINE_CURVE((1.,0.923879532511287,1.,0.923879532511287,1.,0.923879532511287,
1.,0.923879532511287,1.,0.923879532511287,1.,0.923879532511287,1.,0.923879532511287,
1.,0.923879532511287,1.))
REPRESENTATION_ITEM('')
);
#728=(
BOUNDED_CURVE()
B_SPLINE_CURVE(2,(#6869,#6870,#6871,#6872,#6873,#6874,#6875,#6876,#6877,
#6878,#6879,#6880,#6881,#6882,#6883,#6884,#6885),.UNSPECIFIED.,.F.,.F.)
B_SPLINE_CURVE_WITH_KNOTS((3,2,2,2,2,2,2,2,3),(0.415,0.4175,0.42,0.4225,
0.425,0.4275,0.43,0.4325,0.435),.UNSPECIFIED.)
CURVE()
GEOMETRIC_REPRESENTATION_ITEM()
RATIONAL_B_SPLINE_CURVE((1.,0.923879532511287,1.,0.923879532511287,1.,0.923879532511287,
1.,0.923879532511287,1.,0.923879532511287,1.,0.923879532511287,1.,0.923879532511287,
1.,0.923879532511287,1.))
REPRESENTATION_ITEM('')
);
#729=(
BOUNDED_CURVE()
B_SPLINE_CURVE(2,(#6886,#6887,#6888,#6889,#6890,#6891,#6892,#6893,#6894,
#6895,#6896,#6897,#6898,#6899,#6900,#6901,#6902),.UNSPECIFIED.,.F.,.F.)
B_SPLINE_CURVE_WITH_KNOTS((3,2,2,2,2,2,2,2,3),(0.395,0.3975,0.4,0.4025,
0.405,0.4075,0.41,0.4125,0.415),.UNSPECIFIED.)
CURVE()
GEOMETRIC_REPRESENTATION_ITEM()
RATIONAL_B_SPLINE_CURVE((1.,0.923879532511287,1.,0.923879532511287,1.,0.923879532511287,
1.,0.923879532511287,1.,0.923879532511287,1.,0.923879532511287,1.,0.923879532511287,
1.,0.923879532511287,1.))
REPRESENTATION_ITEM('')
);
#730=(
BOUNDED_CURVE()
B_SPLINE_CURVE(2,(#6907,#6908,#6909,#6910,#6911,#6912,#6913,#6914,#6915,
#6916,#6917,#6918,#6919,#6920,#6921,#6922,#6923),.UNSPECIFIED.,.F.,.F.)
B_SPLINE_CURVE_WITH_KNOTS((3,2,2,2,2,2,2,2,3),(0.395,0.3975,0.4,0.4025,
0.405,0.4075,0.41,0.4125,0.415),.UNSPECIFIED.)
CURVE()
GEOMETRIC_REPRESENTATION_ITEM()
RATIONAL_B_SPLINE_CURVE((1.,0.923879532511287,1.,0.923879532511287,1.,0.923879532511287,
1.,0.923879532511287,1.,0.923879532511287,1.,0.923879532511287,1.,0.923879532511287,
1.,0.923879532511287,1.))
REPRESENTATION_ITEM('')
);
#731=(
BOUNDED_CURVE()
B_SPLINE_CURVE(2,(#6924,#6925,#6926,#6927,#6928,#6929,#6930,#6931,#6932,
#6933,#6934,#6935,#6936,#6937,#6938,#6939,#6940),.UNSPECIFIED.,.F.,.F.)
B_SPLINE_CURVE_WITH_KNOTS((3,2,2,2,2,2,2,2,3),(0.375,0.3775,0.38,0.3825,
0.385,0.3875,0.39,0.3925,0.395),.UNSPECIFIED.)
CURVE()
GEOMETRIC_REPRESENTATION_ITEM()
RATIONAL_B_SPLINE_CURVE((1.,0.923879532511287,1.,0.923879532511287,1.,0.923879532511287,
1.,0.923879532511287,1.,0.923879532511287,1.,0.923879532511287,1.,0.923879532511287,
1.,0.923879532511287,1.))
REPRESENTATION_ITEM('')
);
#732=(
BOUNDED_CURVE()
B_SPLINE_CURVE(2,(#6945,#6946,#6947,#6948,#6949,#6950,#6951,#6952,#6953,
#6954,#6955,#6956,#6957,#6958,#6959,#6960,#6961),.UNSPECIFIED.,.F.,.F.)
B_SPLINE_CURVE_WITH_KNOTS((3,2,2,2,2,2,2,2,3),(0.375,0.3775,0.38,0.3825,
0.385,0.3875,0.39,0.3925,0.395),.UNSPECIFIED.)
CURVE()
GEOMETRIC_REPRESENTATION_ITEM()
RATIONAL_B_SPLINE_CURVE((1.,0.923879532511287,1.,0.923879532511287,1.,0.923879532511287,
1.,0.923879532511287,1.,0.923879532511287,1.,0.923879532511287,1.,0.923879532511287,
1.,0.923879532511287,1.))
REPRESENTATION_ITEM('')
);
#733=(
BOUNDED_CURVE()
B_SPLINE_CURVE(2,(#6962,#6963,#6964,#6965,#6966,#6967,#6968,#6969,#6970,
#6971,#6972,#6973,#6974,#6975,#6976,#6977,#6978),.UNSPECIFIED.,.F.,.F.)
B_SPLINE_CURVE_WITH_KNOTS((3,2,2,2,2,2,2,2,3),(0.355,0.3575,0.36,0.3625,
0.365,0.3675,0.37,0.3725,0.375),.UNSPECIFIED.)
CURVE()
GEOMETRIC_REPRESENTATION_ITEM()
RATIONAL_B_SPLINE_CURVE((1.,0.923879532511287,1.,0.923879532511287,1.,0.923879532511287,
1.,0.923879532511287,1.,0.923879532511287,1.,0.923879532511287,1.,0.923879532511287,
1.,0.923879532511287,1.))
REPRESENTATION_ITEM('')
);
#734=(
BOUNDED_CURVE()
B_SPLINE_CURVE(2,(#6983,#6984,#6985,#6986,#6987,#6988,#6989,#6990,#6991,
#6992,#6993,#6994,#6995,#6996,#6997,#6998,#6999),.UNSPECIFIED.,.F.,.F.)
B_SPLINE_CURVE_WITH_KNOTS((3,2,2,2,2,2,2,2,3),(0.355,0.3575,0.36,0.3625,
0.365,0.3675,0.37,0.3725,0.375),.UNSPECIFIED.)
CURVE()
GEOMETRIC_REPRESENTATION_ITEM()
RATIONAL_B_SPLINE_CURVE((1.,0.923879532511287,1.,0.923879532511287,1.,0.923879532511287,
1.,0.923879532511287,1.,0.923879532511287,1.,0.923879532511287,1.,0.923879532511287,
1.,0.923879532511287,1.))
REPRESENTATION_ITEM('')
);
#735=(
BOUNDED_CURVE()
B_SPLINE_CURVE(2,(#7000,#7001,#7002,#7003,#7004,#7005,#7006,#7007,#7008,
#7009,#7010,#7011,#7012,#7013,#7014,#7015,#7016),.UNSPECIFIED.,.F.,.F.)
B_SPLINE_CURVE_WITH_KNOTS((3,2,2,2,2,2,2,2,3),(0.335,0.3375,0.34,0.3425,
0.345,0.3475,0.35,0.3525,0.355),.UNSPECIFIED.)
CURVE()
GEOMETRIC_REPRESENTATION_ITEM()
RATIONAL_B_SPLINE_CURVE((1.,0.923879532511287,1.,0.923879532511287,1.,0.923879532511287,
1.,0.923879532511287,1.,0.923879532511287,1.,0.923879532511287,1.,0.923879532511287,
1.,0.923879532511287,1.))
REPRESENTATION_ITEM('')
);
#736=(
BOUNDED_CURVE()
B_SPLINE_CURVE(2,(#7021,#7022,#7023,#7024,#7025,#7026,#7027,#7028,#7029,
#7030,#7031,#7032,#7033,#7034,#7035,#7036,#7037),.UNSPECIFIED.,.F.,.F.)
B_SPLINE_CURVE_WITH_KNOTS((3,2,2,2,2,2,2,2,3),(0.335,0.3375,0.34,0.3425,
0.345,0.3475,0.35,0.3525,0.355),.UNSPECIFIED.)
CURVE()
GEOMETRIC_REPRESENTATION_ITEM()
RATIONAL_B_SPLINE_CURVE((1.,0.923879532511287,1.,0.923879532511287,1.,0.923879532511287,
1.,0.923879532511287,1.,0.923879532511287,1.,0.923879532511287,1.,0.923879532511287,
1.,0.923879532511287,1.))
REPRESENTATION_ITEM('')
);
#737=(
BOUNDED_CURVE()
B_SPLINE_CURVE(2,(#7038,#7039,#7040,#7041,#7042,#7043,#7044,#7045,#7046,
#7047,#7048,#7049,#7050,#7051,#7052,#7053,#7054),.UNSPECIFIED.,.F.,.F.)
B_SPLINE_CURVE_WITH_KNOTS((3,2,2,2,2,2,2,2,3),(0.315,0.3175,0.32,0.3225,
0.325,0.3275,0.33,0.3325,0.335),.UNSPECIFIED.)
CURVE()
GEOMETRIC_REPRESENTATION_ITEM()
RATIONAL_B_SPLINE_CURVE((1.,0.923879532511287,1.,0.923879532511287,1.,0.923879532511287,
1.,0.923879532511287,1.,0.923879532511287,1.,0.923879532511287,1.,0.923879532511287,
1.,0.923879532511287,1.))
REPRESENTATION_ITEM('')
);
#738=(
BOUNDED_CURVE()
B_SPLINE_CURVE(2,(#7059,#7060,#7061,#7062,#7063,#7064,#7065,#7066,#7067,
#7068,#7069,#7070,#7071,#7072,#7073,#7074,#7075),.UNSPECIFIED.,.F.,.F.)
B_SPLINE_CURVE_WITH_KNOTS((3,2,2,2,2,2,2,2,3),(0.315,0.3175,0.32,0.3225,
0.325,0.3275,0.33,0.3325,0.335),.UNSPECIFIED.)
CURVE()
GEOMETRIC_REPRESENTATION_ITEM()
RATIONAL_B_SPLINE_CURVE((1.,0.923879532511287,1.,0.923879532511287,1.,0.923879532511287,
1.,0.923879532511287,1.,0.923879532511287,1.,0.923879532511287,1.,0.923879532511287,
1.,0.923879532511287,1.))
REPRESENTATION_ITEM('')
);
#739=(
BOUNDED_CURVE()
B_SPLINE_CURVE(2,(#7076,#7077,#7078,#7079,#7080,#7081,#7082,#7083,#7084,
#7085,#7086,#7087,#7088,#7089,#7090,#7091,#7092),.UNSPECIFIED.,.F.,.F.)
B_SPLINE_CURVE_WITH_KNOTS((3,2,2,2,2,2,2,2,3),(0.295,0.2975,0.3,0.3025,
0.305,0.3075,0.31,0.3125,0.315),.UNSPECIFIED.)
CURVE()
GEOMETRIC_REPRESENTATION_ITEM()
RATIONAL_B_SPLINE_CURVE((1.,0.923879532511287,1.,0.923879532511287,1.,0.923879532511287,
1.,0.923879532511287,1.,0.923879532511287,1.,0.923879532511287,1.,0.923879532511287,
1.,0.923879532511287,1.))
REPRESENTATION_ITEM('')
);
#740=(
BOUNDED_CURVE()
B_SPLINE_CURVE(2,(#7097,#7098,#7099,#7100,#7101,#7102,#7103,#7104,#7105,
#7106,#7107,#7108,#7109,#7110,#7111,#7112,#7113),.UNSPECIFIED.,.F.,.F.)
B_SPLINE_CURVE_WITH_KNOTS((3,2,2,2,2,2,2,2,3),(0.295,0.2975,0.3,0.3025,
0.305,0.3075,0.31,0.3125,0.315),.UNSPECIFIED.)
CURVE()
GEOMETRIC_REPRESENTATION_ITEM()
RATIONAL_B_SPLINE_CURVE((1.,0.923879532511287,1.,0.923879532511287,1.,0.923879532511287,
1.,0.923879532511287,1.,0.923879532511287,1.,0.923879532511287,1.,0.923879532511287,
1.,0.923879532511287,1.))
REPRESENTATION_ITEM('')
);
#741=(
BOUNDED_CURVE()
B_SPLINE_CURVE(2,(#7114,#7115,#7116,#7117,#7118,#7119,#7120,#7121,#7122,
#7123,#7124,#7125,#7126,#7127,#7128,#7129,#7130),.UNSPECIFIED.,.F.,.F.)
B_SPLINE_CURVE_WITH_KNOTS((3,2,2,2,2,2,2,2,3),(0.275,0.2775,0.28,0.2825,
0.285,0.2875,0.29,0.2925,0.295),.UNSPECIFIED.)
CURVE()
GEOMETRIC_REPRESENTATION_ITEM()
RATIONAL_B_SPLINE_CURVE((1.,0.923879532511287,1.,0.923879532511287,1.,0.923879532511287,
1.,0.923879532511287,1.,0.923879532511287,1.,0.923879532511287,1.,0.923879532511287,
1.,0.923879532511287,1.))
REPRESENTATION_ITEM('')
);
#742=(
BOUNDED_CURVE()
B_SPLINE_CURVE(2,(#7135,#7136,#7137,#7138,#7139,#7140,#7141,#7142,#7143,
#7144,#7145,#7146,#7147,#7148,#7149,#7150,#7151),.UNSPECIFIED.,.F.,.F.)
B_SPLINE_CURVE_WITH_KNOTS((3,2,2,2,2,2,2,2,3),(0.275,0.2775,0.28,0.2825,
0.285,0.2875,0.29,0.2925,0.295),.UNSPECIFIED.)
CURVE()
GEOMETRIC_REPRESENTATION_ITEM()
RATIONAL_B_SPLINE_CURVE((1.,0.923879532511287,1.,0.923879532511287,1.,0.923879532511287,
1.,0.923879532511287,1.,0.923879532511287,1.,0.923879532511287,1.,0.923879532511287,
1.,0.923879532511287,1.))
REPRESENTATION_ITEM('')
);
#743=(
BOUNDED_CURVE()
B_SPLINE_CURVE(2,(#7152,#7153,#7154,#7155,#7156,#7157,#7158,#7159,#7160,
#7161,#7162,#7163,#7164,#7165,#7166,#7167,#7168),.UNSPECIFIED.,.F.,.F.)
B_SPLINE_CURVE_WITH_KNOTS((3,2,2,2,2,2,2,2,3),(0.255,0.2575,0.26,0.2625,
0.265,0.2675,0.27,0.2725,0.275),.UNSPECIFIED.)
CURVE()
GEOMETRIC_REPRESENTATION_ITEM()
RATIONAL_B_SPLINE_CURVE((1.,0.923879532511287,1.,0.923879532511287,1.,0.923879532511287,
1.,0.923879532511287,1.,0.923879532511287,1.,0.923879532511287,1.,0.923879532511287,
1.,0.923879532511287,1.))
REPRESENTATION_ITEM('')
);
#744=(
BOUNDED_CURVE()
B_SPLINE_CURVE(2,(#7173,#7174,#7175,#7176,#7177,#7178,#7179,#7180,#7181,
#7182,#7183,#7184,#7185,#7186,#7187,#7188,#7189),.UNSPECIFIED.,.F.,.F.)
B_SPLINE_CURVE_WITH_KNOTS((3,2,2,2,2,2,2,2,3),(0.255,0.2575,0.26,0.2625,
0.265,0.2675,0.27,0.2725,0.275),.UNSPECIFIED.)
CURVE()
GEOMETRIC_REPRESENTATION_ITEM()
RATIONAL_B_SPLINE_CURVE((1.,0.923879532511287,1.,0.923879532511287,1.,0.923879532511287,
1.,0.923879532511287,1.,0.923879532511287,1.,0.923879532511287,1.,0.923879532511287,
1.,0.923879532511287,1.))
REPRESENTATION_ITEM('')
);
#745=(
BOUNDED_CURVE()
B_SPLINE_CURVE(2,(#7190,#7191,#7192,#7193,#7194,#7195,#7196,#7197,#7198,
#7199,#7200,#7201,#7202,#7203,#7204,#7205,#7206),.UNSPECIFIED.,.F.,.F.)
B_SPLINE_CURVE_WITH_KNOTS((3,2,2,2,2,2,2,2,3),(0.235,0.2375,0.24,0.2425,
0.245,0.2475,0.25,0.2525,0.255),.UNSPECIFIED.)
CURVE()
GEOMETRIC_REPRESENTATION_ITEM()
RATIONAL_B_SPLINE_CURVE((1.,0.923879532511287,1.,0.923879532511287,1.,0.923879532511287,
1.,0.923879532511287,1.,0.923879532511287,1.,0.923879532511287,1.,0.923879532511287,
1.,0.923879532511287,1.))
REPRESENTATION_ITEM('')
);
#746=(
BOUNDED_CURVE()
B_SPLINE_CURVE(2,(#7211,#7212,#7213,#7214,#7215,#7216,#7217,#7218,#7219,
#7220,#7221,#7222,#7223,#7224,#7225,#7226,#7227),.UNSPECIFIED.,.F.,.F.)
B_SPLINE_CURVE_WITH_KNOTS((3,2,2,2,2,2,2,2,3),(0.235,0.2375,0.24,0.2425,
0.245,0.2475,0.25,0.2525,0.255),.UNSPECIFIED.)
CURVE()
GEOMETRIC_REPRESENTATION_ITEM()
RATIONAL_B_SPLINE_CURVE((1.,0.923879532511287,1.,0.923879532511287,1.,0.923879532511287,
1.,0.923879532511287,1.,0.923879532511287,1.,0.923879532511287,1.,0.923879532511287,
1.,0.923879532511287,1.))
REPRESENTATION_ITEM('')
);
#747=(
BOUNDED_CURVE()
B_SPLINE_CURVE(2,(#7228,#7229,#7230,#7231,#7232,#7233,#7234,#7235,#7236,
#7237,#7238,#7239,#7240,#7241,#7242,#7243,#7244),.UNSPECIFIED.,.F.,.F.)
B_SPLINE_CURVE_WITH_KNOTS((3,2,2,2,2,2,2,2,3),(0.215,0.2175,0.22,0.2225,
0.225,0.2275,0.23,0.2325,0.235),.UNSPECIFIED.)
CURVE()
GEOMETRIC_REPRESENTATION_ITEM()
RATIONAL_B_SPLINE_CURVE((1.,0.923879532511287,1.,0.923879532511287,1.,0.923879532511287,
1.,0.923879532511287,1.,0.923879532511287,1.,0.923879532511287,1.,0.923879532511287,
1.,0.923879532511287,1.))
REPRESENTATION_ITEM('')
);
#748=(
BOUNDED_CURVE()
B_SPLINE_CURVE(2,(#7249,#7250,#7251,#7252,#7253,#7254,#7255,#7256,#7257,
#7258,#7259,#7260,#7261,#7262,#7263,#7264,#7265),.UNSPECIFIED.,.F.,.F.)
B_SPLINE_CURVE_WITH_KNOTS((3,2,2,2,2,2,2,2,3),(0.215,0.2175,0.22,0.2225,
0.225,0.2275,0.23,0.2325,0.235),.UNSPECIFIED.)
CURVE()
GEOMETRIC_REPRESENTATION_ITEM()
RATIONAL_B_SPLINE_CURVE((1.,0.923879532511287,1.,0.923879532511287,1.,0.923879532511287,
1.,0.923879532511287,1.,0.923879532511287,1.,0.923879532511287,1.,0.923879532511287,
1.,0.923879532511287,1.))
REPRESENTATION_ITEM('')
);
#749=(
BOUNDED_CURVE()
B_SPLINE_CURVE(2,(#7266,#7267,#7268,#7269,#7270,#7271,#7272,#7273,#7274,
#7275,#7276,#7277,#7278,#7279,#7280,#7281,#7282),.UNSPECIFIED.,.F.,.F.)
B_SPLINE_CURVE_WITH_KNOTS((3,2,2,2,2,2,2,2,3),(0.195,0.1975,0.2,0.2025,
0.205,0.2075,0.21,0.2125,0.215),.UNSPECIFIED.)
CURVE()
GEOMETRIC_REPRESENTATION_ITEM()
RATIONAL_B_SPLINE_CURVE((1.,0.923879532511287,1.,0.923879532511287,1.,0.923879532511287,
1.,0.923879532511287,1.,0.923879532511287,1.,0.923879532511287,1.,0.923879532511287,
1.,0.923879532511287,1.))
REPRESENTATION_ITEM('')
);
#750=(
BOUNDED_CURVE()
B_SPLINE_CURVE(2,(#7287,#7288,#7289,#7290,#7291,#7292,#7293,#7294,#7295,
#7296,#7297,#7298,#7299,#7300,#7301,#7302,#7303),.UNSPECIFIED.,.F.,.F.)
B_SPLINE_CURVE_WITH_KNOTS((3,2,2,2,2,2,2,2,3),(0.195,0.1975,0.2,0.2025,
0.205,0.2075,0.21,0.2125,0.215),.UNSPECIFIED.)
CURVE()
GEOMETRIC_REPRESENTATION_ITEM()
RATIONAL_B_SPLINE_CURVE((1.,0.923879532511287,1.,0.923879532511287,1.,0.923879532511287,
1.,0.923879532511287,1.,0.923879532511287,1.,0.923879532511287,1.,0.923879532511287,
1.,0.923879532511287,1.))
REPRESENTATION_ITEM('')
);
#751=(
BOUNDED_CURVE()
B_SPLINE_CURVE(2,(#7304,#7305,#7306,#7307,#7308,#7309,#7310,#7311,#7312,
#7313,#7314,#7315,#7316,#7317,#7318,#7319,#7320),.UNSPECIFIED.,.F.,.F.)
B_SPLINE_CURVE_WITH_KNOTS((3,2,2,2,2,2,2,2,3),(0.175,0.1775,0.18,0.1825,
0.185,0.1875,0.19,0.1925,0.195),.UNSPECIFIED.)
CURVE()
GEOMETRIC_REPRESENTATION_ITEM()
RATIONAL_B_SPLINE_CURVE((1.,0.923879532511287,1.,0.923879532511287,1.,0.923879532511287,
1.,0.923879532511287,1.,0.923879532511287,1.,0.923879532511287,1.,0.923879532511287,
1.,0.923879532511287,1.))
REPRESENTATION_ITEM('')
);
#752=(
BOUNDED_CURVE()
B_SPLINE_CURVE(2,(#7325,#7326,#7327,#7328,#7329,#7330,#7331,#7332,#7333,
#7334,#7335,#7336,#7337,#7338,#7339,#7340,#7341),.UNSPECIFIED.,.F.,.F.)
B_SPLINE_CURVE_WITH_KNOTS((3,2,2,2,2,2,2,2,3),(0.175,0.1775,0.18,0.1825,
0.185,0.1875,0.19,0.1925,0.195),.UNSPECIFIED.)
CURVE()
GEOMETRIC_REPRESENTATION_ITEM()
RATIONAL_B_SPLINE_CURVE((1.,0.923879532511287,1.,0.923879532511287,1.,0.923879532511287,
1.,0.923879532511287,1.,0.923879532511287,1.,0.923879532511287,1.,0.923879532511287,
1.,0.923879532511287,1.))
REPRESENTATION_ITEM('')
);
#753=(
BOUNDED_CURVE()
B_SPLINE_CURVE(2,(#7342,#7343,#7344,#7345,#7346,#7347,#7348,#7349,#7350,
#7351,#7352,#7353,#7354,#7355,#7356,#7357,#7358),.UNSPECIFIED.,.F.,.F.)
B_SPLINE_CURVE_WITH_KNOTS((3,2,2,2,2,2,2,2,3),(0.155,0.1575,0.16,0.1625,
0.165,0.1675,0.17,0.1725,0.175),.UNSPECIFIED.)
CURVE()
GEOMETRIC_REPRESENTATION_ITEM()
RATIONAL_B_SPLINE_CURVE((1.,0.923879532511287,1.,0.923879532511287,1.,0.923879532511287,
1.,0.923879532511287,1.,0.923879532511287,1.,0.923879532511287,1.,0.923879532511287,
1.,0.923879532511287,1.))
REPRESENTATION_ITEM('')
);
#754=(
BOUNDED_CURVE()
B_SPLINE_CURVE(2,(#7363,#7364,#7365,#7366,#7367,#7368,#7369,#7370,#7371,
#7372,#7373,#7374,#7375,#7376,#7377,#7378,#7379),.UNSPECIFIED.,.F.,.F.)
B_SPLINE_CURVE_WITH_KNOTS((3,2,2,2,2,2,2,2,3),(0.155,0.1575,0.16,0.1625,
0.165,0.1675,0.17,0.1725,0.175),.UNSPECIFIED.)
CURVE()
GEOMETRIC_REPRESENTATION_ITEM()
RATIONAL_B_SPLINE_CURVE((1.,0.923879532511287,1.,0.923879532511287,1.,0.923879532511287,
1.,0.923879532511287,1.,0.923879532511287,1.,0.923879532511287,1.,0.923879532511287,
1.,0.923879532511287,1.))
REPRESENTATION_ITEM('')
);
#755=(
BOUNDED_CURVE()
B_SPLINE_CURVE(2,(#7380,#7381,#7382,#7383,#7384,#7385,#7386,#7387,#7388,
#7389,#7390,#7391,#7392,#7393,#7394,#7395,#7396),.UNSPECIFIED.,.F.,.F.)
B_SPLINE_CURVE_WITH_KNOTS((3,2,2,2,2,2,2,2,3),(0.135,0.1375,0.14,0.1425,
0.145,0.1475,0.15,0.1525,0.155),.UNSPECIFIED.)
CURVE()
GEOMETRIC_REPRESENTATION_ITEM()
RATIONAL_B_SPLINE_CURVE((1.,0.923879532511287,1.,0.923879532511287,1.,0.923879532511287,
1.,0.923879532511287,1.,0.923879532511287,1.,0.923879532511287,1.,0.923879532511287,
1.,0.923879532511287,1.))
REPRESENTATION_ITEM('')
);
#756=(
BOUNDED_CURVE()
B_SPLINE_CURVE(2,(#7401,#7402,#7403,#7404,#7405,#7406,#7407,#7408,#7409,
#7410,#7411,#7412,#7413,#7414,#7415,#7416,#7417),.UNSPECIFIED.,.F.,.F.)
B_SPLINE_CURVE_WITH_KNOTS((3,2,2,2,2,2,2,2,3),(0.135,0.1375,0.14,0.1425,
0.145,0.1475,0.15,0.1525,0.155),.UNSPECIFIED.)
CURVE()
GEOMETRIC_REPRESENTATION_ITEM()
RATIONAL_B_SPLINE_CURVE((1.,0.923879532511287,1.,0.923879532511287,1.,0.923879532511287,
1.,0.923879532511287,1.,0.923879532511287,1.,0.923879532511287,1.,0.923879532511287,
1.,0.923879532511287,1.))
REPRESENTATION_ITEM('')
);
#757=(
BOUNDED_CURVE()
B_SPLINE_CURVE(2,(#7418,#7419,#7420,#7421,#7422,#7423,#7424,#7425,#7426,
#7427,#7428,#7429,#7430,#7431,#7432,#7433,#7434),.UNSPECIFIED.,.F.,.F.)
B_SPLINE_CURVE_WITH_KNOTS((3,2,2,2,2,2,2,2,3),(0.115,0.1175,0.12,0.1225,
0.125,0.1275,0.13,0.1325,0.135),.UNSPECIFIED.)
CURVE()
GEOMETRIC_REPRESENTATION_ITEM()
RATIONAL_B_SPLINE_CURVE((1.,0.923879532511287,1.,0.923879532511287,1.,0.923879532511287,
1.,0.923879532511287,1.,0.923879532511287,1.,0.923879532511287,1.,0.923879532511287,
1.,0.923879532511287,1.))
REPRESENTATION_ITEM('')
);
#758=(
BOUNDED_CURVE()
B_SPLINE_CURVE(2,(#7439,#7440,#7441,#7442,#7443,#7444,#7445,#7446,#7447,
#7448,#7449,#7450,#7451,#7452,#7453,#7454,#7455),.UNSPECIFIED.,.F.,.F.)
B_SPLINE_CURVE_WITH_KNOTS((3,2,2,2,2,2,2,2,3),(0.115,0.1175,0.12,0.1225,
0.125,0.1275,0.13,0.1325,0.135),.UNSPECIFIED.)
CURVE()
GEOMETRIC_REPRESENTATION_ITEM()
RATIONAL_B_SPLINE_CURVE((1.,0.923879532511287,1.,0.923879532511287,1.,0.923879532511287,
1.,0.923879532511287,1.,0.923879532511287,1.,0.923879532511287,1.,0.923879532511287,
1.,0.923879532511287,1.))
REPRESENTATION_ITEM('')
);
#759=(
BOUNDED_CURVE()
B_SPLINE_CURVE(2,(#7456,#7457,#7458,#7459,#7460,#7461,#7462,#7463,#7464,
#7465,#7466,#7467,#7468,#7469,#7470,#7471,#7472),.UNSPECIFIED.,.F.,.F.)
B_SPLINE_CURVE_WITH_KNOTS((3,2,2,2,2,2,2,2,3),(0.095,0.0975,0.1,0.1025,
0.105,0.1075,0.11,0.1125,0.115),.UNSPECIFIED.)
CURVE()
GEOMETRIC_REPRESENTATION_ITEM()
RATIONAL_B_SPLINE_CURVE((1.,0.923879532511287,1.,0.923879532511287,1.,0.923879532511287,
1.,0.923879532511287,1.,0.923879532511287,1.,0.923879532511287,1.,0.923879532511287,
1.,0.923879532511287,1.))
REPRESENTATION_ITEM('')
);
#760=(
BOUNDED_CURVE()
B_SPLINE_CURVE(2,(#7477,#7478,#7479,#7480,#7481,#7482,#7483,#7484,#7485,
#7486,#7487,#7488,#7489,#7490,#7491,#7492,#7493),.UNSPECIFIED.,.F.,.F.)
B_SPLINE_CURVE_WITH_KNOTS((3,2,2,2,2,2,2,2,3),(0.095,0.0975,0.1,0.1025,
0.105,0.1075,0.11,0.1125,0.115),.UNSPECIFIED.)
CURVE()
GEOMETRIC_REPRESENTATION_ITEM()
RATIONAL_B_SPLINE_CURVE((1.,0.923879532511287,1.,0.923879532511287,1.,0.923879532511287,
1.,0.923879532511287,1.,0.923879532511287,1.,0.923879532511287,1.,0.923879532511287,
1.,0.923879532511287,1.))
REPRESENTATION_ITEM('')
);
#761=(
BOUNDED_CURVE()
B_SPLINE_CURVE(2,(#7494,#7495,#7496,#7497,#7498,#7499,#7500,#7501,#7502,
#7503,#7504,#7505,#7506,#7507,#7508,#7509,#7510),.UNSPECIFIED.,.F.,.F.)
B_SPLINE_CURVE_WITH_KNOTS((3,2,2,2,2,2,2,2,3),(0.075,0.0775,0.08,0.0825,
0.085,0.0875,0.09,0.0925,0.095),.UNSPECIFIED.)
CURVE()
GEOMETRIC_REPRESENTATION_ITEM()
RATIONAL_B_SPLINE_CURVE((1.,0.923879532511287,1.,0.923879532511287,1.,0.923879532511287,
1.,0.923879532511287,1.,0.923879532511287,1.,0.923879532511287,1.,0.923879532511287,
1.,0.923879532511287,1.))
REPRESENTATION_ITEM('')
);
#762=(
BOUNDED_CURVE()
B_SPLINE_CURVE(2,(#7515,#7516,#7517,#7518,#7519,#7520,#7521,#7522,#7523,
#7524,#7525,#7526,#7527,#7528,#7529,#7530,#7531),.UNSPECIFIED.,.F.,.F.)
B_SPLINE_CURVE_WITH_KNOTS((3,2,2,2,2,2,2,2,3),(0.075,0.0775,0.08,0.0825,
0.085,0.0875,0.09,0.0925,0.095),.UNSPECIFIED.)
CURVE()
GEOMETRIC_REPRESENTATION_ITEM()
RATIONAL_B_SPLINE_CURVE((1.,0.923879532511287,1.,0.923879532511287,1.,0.923879532511287,
1.,0.923879532511287,1.,0.923879532511287,1.,0.923879532511287,1.,0.923879532511287,
1.,0.923879532511287,1.))
REPRESENTATION_ITEM('')
);
#763=(
BOUNDED_CURVE()
B_SPLINE_CURVE(2,(#7532,#7533,#7534,#7535,#7536,#7537,#7538,#7539,#7540,
#7541,#7542,#7543,#7544,#7545,#7546,#7547,#7548),.UNSPECIFIED.,.F.,.F.)
B_SPLINE_CURVE_WITH_KNOTS((3,2,2,2,2,2,2,2,3),(0.055,0.0575,0.06,0.0625,
0.065,0.0675,0.07,0.0725,0.075),.UNSPECIFIED.)
CURVE()
GEOMETRIC_REPRESENTATION_ITEM()
RATIONAL_B_SPLINE_CURVE((1.,0.923879532511287,1.,0.923879532511287,1.,0.923879532511287,
1.,0.923879532511287,1.,0.923879532511287,1.,0.923879532511287,1.,0.923879532511287,
1.,0.923879532511287,1.))
REPRESENTATION_ITEM('')
);
#764=(
BOUNDED_CURVE()
B_SPLINE_CURVE(2,(#7553,#7554,#7555,#7556,#7557,#7558,#7559,#7560,#7561,
#7562,#7563,#7564,#7565,#7566,#7567,#7568,#7569),.UNSPECIFIED.,.F.,.F.)
B_SPLINE_CURVE_WITH_KNOTS((3,2,2,2,2,2,2,2,3),(0.055,0.0575,0.06,0.0625,
0.065,0.0675,0.07,0.0725,0.075),.UNSPECIFIED.)
CURVE()
GEOMETRIC_REPRESENTATION_ITEM()
RATIONAL_B_SPLINE_CURVE((1.,0.923879532511287,1.,0.923879532511287,1.,0.923879532511287,
1.,0.923879532511287,1.,0.923879532511287,1.,0.923879532511287,1.,0.923879532511287,
1.,0.923879532511287,1.))
REPRESENTATION_ITEM('')
);
#765=(
BOUNDED_CURVE()
B_SPLINE_CURVE(2,(#7570,#7571,#7572,#7573,#7574,#7575,#7576,#7577,#7578,
#7579,#7580,#7581,#7582,#7583,#7584,#7585,#7586),.UNSPECIFIED.,.F.,.F.)
B_SPLINE_CURVE_WITH_KNOTS((3,2,2,2,2,2,2,2,3),(0.035,0.0375,0.04,0.0425,
0.045,0.0475,0.05,0.0525,0.055),.UNSPECIFIED.)
CURVE()
GEOMETRIC_REPRESENTATION_ITEM()
RATIONAL_B_SPLINE_CURVE((1.,0.923879532511287,1.,0.923879532511287,1.,0.923879532511287,
1.,0.923879532511287,1.,0.923879532511287,1.,0.923879532511287,1.,0.923879532511287,
1.,0.923879532511287,1.))
REPRESENTATION_ITEM('')
);
#766=(
BOUNDED_CURVE()
B_SPLINE_CURVE(2,(#7593,#7594,#7595,#7596,#7597,#7598,#7599,#7600,#7601,
#7602,#7603,#7604,#7605,#7606,#7607,#7608,#7609),.UNSPECIFIED.,.F.,.F.)
B_SPLINE_CURVE_WITH_KNOTS((3,2,2,2,2,2,2,2,3),(0.015,0.0175,0.02,0.0225,
0.025,0.0275,0.03,0.0325,0.035),.UNSPECIFIED.)
CURVE()
GEOMETRIC_REPRESENTATION_ITEM()
RATIONAL_B_SPLINE_CURVE((1.,0.923879532511287,1.,0.923879532511287,1.,0.923879532511287,
1.,0.923879532511287,1.,0.923879532511287,1.,0.923879532511287,1.,0.923879532511287,
1.,0.923879532511287,1.))
REPRESENTATION_ITEM('')
);
#767=(
BOUNDED_CURVE()
B_SPLINE_CURVE(2,(#7613,#7614,#7615,#7616,#7617,#7618,#7619,#7620,#7621,
#7622,#7623,#7624,#7625),.UNSPECIFIED.,.F.,.F.)
B_SPLINE_CURVE_WITH_KNOTS((3,2,2,2,2,2,3),(0.,0.0025,0.005,0.0075,0.01,
0.0125,0.015),.UNSPECIFIED.)
CURVE()
GEOMETRIC_REPRESENTATION_ITEM()
RATIONAL_B_SPLINE_CURVE((1.,0.923879532511287,1.,0.923879532511287,1.,0.923879532511287,
1.,0.923879532511287,1.,0.923879532511287,1.,0.923879532511287,1.))
REPRESENTATION_ITEM('')
);
#768=(
BOUNDED_CURVE()
B_SPLINE_CURVE(2,(#7628,#7629,#7630,#7631,#7632,#7633,#7634,#7635,#7636,
#7637,#7638,#7639,#7640),.UNSPECIFIED.,.F.,.F.)
B_SPLINE_CURVE_WITH_KNOTS((3,2,2,2,2,2,3),(0.,0.0025,0.005,0.0075,0.01,
0.0125,0.015),.UNSPECIFIED.)
CURVE()
GEOMETRIC_REPRESENTATION_ITEM()
RATIONAL_B_SPLINE_CURVE((1.,0.923879532511287,1.,0.923879532511287,1.,0.923879532511287,
1.,0.923879532511287,1.,0.923879532511287,1.,0.923879532511287,1.))
REPRESENTATION_ITEM('')
);
#769=(
BOUNDED_CURVE()
B_SPLINE_CURVE(2,(#7726,#7727,#7728,#7729,#7730,#7731,#7732,#7733,#7734,
#7735,#7736,#7737,#7738,#7739,#7740,#7741,#7742),.UNSPECIFIED.,.F.,.F.)
B_SPLINE_CURVE_WITH_KNOTS((3,2,2,2,2,2,2,2,3),(0.035,0.0375,0.04,0.0425,
0.045,0.0475,0.05,0.0525,0.055),.UNSPECIFIED.)
CURVE()
GEOMETRIC_REPRESENTATION_ITEM()
RATIONAL_B_SPLINE_CURVE((1.,0.923879532511287,1.,0.923879532511287,1.,0.923879532511287,
1.,0.923879532511287,1.,0.923879532511287,1.,0.923879532511287,1.,0.923879532511287,
1.,0.923879532511287,1.))
REPRESENTATION_ITEM('')
);
#770=(
BOUNDED_CURVE()
B_SPLINE_CURVE(2,(#7743,#7744,#7745,#7746,#7747,#7748,#7749,#7750,#7751,
#7752,#7753,#7754,#7755,#7756,#7757,#7758,#7759),.UNSPECIFIED.,.F.,.F.)
B_SPLINE_CURVE_WITH_KNOTS((3,2,2,2,2,2,2,2,3),(0.015,0.0175,0.02,0.0225,
0.025,0.0275,0.03,0.0325,0.035),.UNSPECIFIED.)
CURVE()
GEOMETRIC_REPRESENTATION_ITEM()
RATIONAL_B_SPLINE_CURVE((1.,0.923879532511287,1.,0.923879532511287,1.,0.923879532511287,
1.,0.923879532511287,1.,0.923879532511287,1.,0.923879532511287,1.,0.923879532511287,
1.,0.923879532511287,1.))
REPRESENTATION_ITEM('')
);
#771=(
BOUNDED_CURVE()
B_SPLINE_CURVE(2,(#9384,#9385,#9386,#9387,#9388,#9389,#9390,#9391,#9392,
#9393,#9394,#9395,#9396,#9397,#9398,#9399,#9400),.UNSPECIFIED.,.F.,.F.)
B_SPLINE_CURVE_WITH_KNOTS((3,2,2,2,2,2,2,2,3),(0.01,0.0125,0.015,0.0175,
0.02,0.0225,0.025,0.0275,0.03),.UNSPECIFIED.)
CURVE()
GEOMETRIC_REPRESENTATION_ITEM()
RATIONAL_B_SPLINE_CURVE((1.,0.923879532511287,1.,0.923879532511287,1.,0.923879532511287,
1.,0.923879532511287,1.,0.923879532511287,1.,0.923879532511287,1.,0.923879532511287,
1.,0.923879532511287,1.))
REPRESENTATION_ITEM('')
);
#772=(
BOUNDED_CURVE()
B_SPLINE_CURVE(2,(#9402,#9403,#9404,#9405,#9406,#9407,#9408,#9409,#9410,
#9411,#9412,#9413,#9414,#9415,#9416,#9417,#9418),.UNSPECIFIED.,.F.,.F.)
B_SPLINE_CURVE_WITH_KNOTS((3,2,2,2,2,2,2,2,3),(0.01,0.0125,0.015,0.0175,
0.02,0.0225,0.025,0.0275,0.03),.UNSPECIFIED.)
CURVE()
GEOMETRIC_REPRESENTATION_ITEM()
RATIONAL_B_SPLINE_CURVE((1.,0.923879532511287,1.,0.923879532511287,1.,0.923879532511287,
1.,0.923879532511287,1.,0.923879532511287,1.,0.923879532511287,1.,0.923879532511287,
1.,0.923879532511287,1.))
REPRESENTATION_ITEM('')
);
#773=(
BOUNDED_CURVE()
B_SPLINE_CURVE(2,(#11021,#11022,#11023,#11024,#11025,#11026,#11027,#11028,
#11029,#11030,#11031,#11032,#11033,#11034,#11035),.UNSPECIFIED.,.F.,.F.)
B_SPLINE_CURVE_WITH_KNOTS((3,2,2,2,2,2,2,3),(0.9825,0.985,0.9875,0.99,0.9925,
0.995,0.9975,1.),.UNSPECIFIED.)
CURVE()
GEOMETRIC_REPRESENTATION_ITEM()
RATIONAL_B_SPLINE_CURVE((1.,0.923879532511287,1.,0.923879532511287,1.,0.923879532511287,
1.,0.923879532511287,1.,0.923879532511287,1.,0.923879532511287,1.,0.923879532511287,
1.))
REPRESENTATION_ITEM('')
);
#780=LINE('',#3911,#931);
#781=LINE('',#3923,#932);
#782=LINE('',#3936,#933);
#783=LINE('',#3974,#934);
#784=LINE('',#4012,#935);
#785=LINE('',#4050,#936);
#786=LINE('',#4088,#937);
#787=LINE('',#4126,#938);
#788=LINE('',#4164,#939);
#789=LINE('',#4202,#940);
#790=LINE('',#4240,#941);
#791=LINE('',#4278,#942);
#792=LINE('',#4316,#943);
#793=LINE('',#4354,#944);
#794=LINE('',#4392,#945);
#795=LINE('',#4430,#946);
#796=LINE('',#4468,#947);
#797=LINE('',#4506,#948);
#798=LINE('',#4544,#949);
#799=LINE('',#4582,#950);
#800=LINE('',#4620,#951);
#801=LINE('',#4658,#952);
#802=LINE('',#4696,#953);
#803=LINE('',#4734,#954);
#804=LINE('',#4772,#955);
#805=LINE('',#4810,#956);
#806=LINE('',#4848,#957);
#807=LINE('',#4886,#958);
#808=LINE('',#4924,#959);
#809=LINE('',#4962,#960);
#810=LINE('',#5000,#961);
#811=LINE('',#5038,#962);
#812=LINE('',#5076,#963);
#813=LINE('',#5114,#964);
#814=LINE('',#5152,#965);
#815=LINE('',#5190,#966);
#816=LINE('',#5228,#967);
#817=LINE('',#5266,#968);
#818=LINE('',#5304,#969);
#819=LINE('',#5342,#970);
#820=LINE('',#5380,#971);
#821=LINE('',#5418,#972);
#822=LINE('',#5456,#973);
#823=LINE('',#5494,#974);
#824=LINE('',#5532,#975);
#825=LINE('',#5570,#976);
#826=LINE('',#5608,#977);
#827=LINE('',#5646,#978);
#828=LINE('',#5684,#979);
#829=LINE('',#5722,#980);
#830=LINE('',#5760,#981);
#831=LINE('',#5772,#982);
#832=LINE('',#5785,#983);
#833=LINE('',#5804,#984);
#834=LINE('',#5842,#985);
#835=LINE('',#5880,#986);
#836=LINE('',#5918,#987);
#837=LINE('',#5956,#988);
#838=LINE('',#5994,#989);
#839=LINE('',#6032,#990);
#840=LINE('',#6070,#991);
#841=LINE('',#6108,#992);
#842=LINE('',#6146,#993);
#843=LINE('',#6184,#994);
#844=LINE('',#6222,#995);
#845=LINE('',#6260,#996);
#846=LINE('',#6298,#997);
#847=LINE('',#6336,#998);
#848=LINE('',#6374,#999);
#849=LINE('',#6412,#1000);
#850=LINE('',#6450,#1001);
#851=LINE('',#6488,#1002);
#852=LINE('',#6526,#1003);
#853=LINE('',#6564,#1004);
#854=LINE('',#6602,#1005);
#855=LINE('',#6640,#1006);
#856=LINE('',#6678,#1007);
#857=LINE('',#6716,#1008);
#858=LINE('',#6754,#1009);
#859=LINE('',#6792,#1010);
#860=LINE('',#6830,#1011);
#861=LINE('',#6868,#1012);
#862=LINE('',#6906,#1013);
#863=LINE('',#6944,#1014);
#864=LINE('',#6982,#1015);
#865=LINE('',#7020,#1016);
#866=LINE('',#7058,#1017);
#867=LINE('',#7096,#1018);
#868=LINE('',#7134,#1019);
#869=LINE('',#7172,#1020);
#870=LINE('',#7210,#1021);
#871=LINE('',#7248,#1022);
#872=LINE('',#7286,#1023);
#873=LINE('',#7324,#1024);
#874=LINE('',#7362,#1025);
#875=LINE('',#7400,#1026);
#876=LINE('',#7438,#1027);
#877=LINE('',#7476,#1028);
#878=LINE('',#7514,#1029);
#879=LINE('',#7552,#1030);
#880=LINE('',#7591,#1031);
#881=LINE('',#7611,#1032);
#882=LINE('',#7627,#1033);
#883=LINE('',#7647,#1034);
#884=LINE('',#7773,#1035);
#885=LINE('',#7775,#1036);
#886=LINE('',#7776,#1037);
#887=LINE('',#7778,#1038);
#888=LINE('',#7780,#1039);
#889=LINE('',#7781,#1040);
#890=LINE('',#11039,#1041);
#891=LINE('',#11044,#1042);
#892=LINE('',#11048,#1043);
#893=LINE('',#11050,#1044);
#931=VECTOR('',#3284,104.958734125);
#932=VECTOR('',#3285,0.25);
#933=VECTOR('',#3288,104.958734125);
#934=VECTOR('',#3291,104.958734125);
#935=VECTOR('',#3294,104.958734125);
#936=VECTOR('',#3297,104.958734125);
#937=VECTOR('',#3300,104.958734125);
#938=VECTOR('',#3303,104.958734125);
#939=VECTOR('',#3306,104.958734125);
#940=VECTOR('',#3309,104.958734125);
#941=VECTOR('',#3312,104.958734125);
#942=VECTOR('',#3315,104.958734125);
#943=VECTOR('',#3318,104.958734125);
#944=VECTOR('',#3321,104.958734125);
#945=VECTOR('',#3324,104.958734125);
#946=VECTOR('',#3327,104.958734125);
#947=VECTOR('',#3330,104.958734125);
#948=VECTOR('',#3333,104.958734125);
#949=VECTOR('',#3336,104.958734125);
#950=VECTOR('',#3339,104.958734125);
#951=VECTOR('',#3342,104.958734125);
#952=VECTOR('',#3345,104.958734125);
#953=VECTOR('',#3348,104.958734125);
#954=VECTOR('',#3351,104.958734125);
#955=VECTOR('',#3354,104.958734125);
#956=VECTOR('',#3357,104.958734125);
#957=VECTOR('',#3360,104.958734125);
#958=VECTOR('',#3363,104.958734125);
#959=VECTOR('',#3366,104.958734125);
#960=VECTOR('',#3369,104.958734125);
#961=VECTOR('',#3372,104.958734125);
#962=VECTOR('',#3375,104.958734125);
#963=VECTOR('',#3378,104.958734125);
#964=VECTOR('',#3381,104.958734125);
#965=VECTOR('',#3384,104.958734125);
#966=VECTOR('',#3387,104.958734125);
#967=VECTOR('',#3390,104.958734125);
#968=VECTOR('',#3393,104.958734125);
#969=VECTOR('',#3396,104.958734125);
#970=VECTOR('',#3399,104.958734125);
#971=VECTOR('',#3402,104.958734125);
#972=VECTOR('',#3405,104.958734125);
#973=VECTOR('',#3408,104.958734125);
#974=VECTOR('',#3411,104.958734125);
#975=VECTOR('',#3414,104.958734125);
#976=VECTOR('',#3417,104.958734125);
#977=VECTOR('',#3420,104.958734125);
#978=VECTOR('',#3423,104.958734125);
#979=VECTOR('',#3426,104.958734125);
#980=VECTOR('',#3429,104.958734125);
#981=VECTOR('',#3432,104.958734125);
#982=VECTOR('',#3433,0.250000000000004);
#983=VECTOR('',#3436,105.5);
#984=VECTOR('',#3441,105.5);
#985=VECTOR('',#3444,105.5);
#986=VECTOR('',#3447,105.5);
#987=VECTOR('',#3450,105.5);
#988=VECTOR('',#3453,105.5);
#989=VECTOR('',#3456,105.5);
#990=VECTOR('',#3459,105.5);
#991=VECTOR('',#3462,105.5);
#992=VECTOR('',#3465,105.5);
#993=VECTOR('',#3468,105.5);
#994=VECTOR('',#3471,105.5);
#995=VECTOR('',#3474,105.5);
#996=VECTOR('',#3477,105.5);
#997=VECTOR('',#3480,105.5);
#998=VECTOR('',#3483,105.5);
#999=VECTOR('',#3486,105.5);
#1000=VECTOR('',#3489,105.5);
#1001=VECTOR('',#3492,105.5);
#1002=VECTOR('',#3495,105.5);
#1003=VECTOR('',#3498,105.5);
#1004=VECTOR('',#3501,105.5);
#1005=VECTOR('',#3504,105.5);
#1006=VECTOR('',#3507,105.5);
#1007=VECTOR('',#3510,105.5);
#1008=VECTOR('',#3513,105.5);
#1009=VECTOR('',#3516,105.5);
#1010=VECTOR('',#3519,105.5);
#1011=VECTOR('',#3522,105.5);
#1012=VECTOR('',#3525,105.5);
#1013=VECTOR('',#3528,105.5);
#1014=VECTOR('',#3531,105.5);
#1015=VECTOR('',#3534,105.5);
#1016=VECTOR('',#3537,105.5);
#1017=VECTOR('',#3540,105.5);
#1018=VECTOR('',#3543,105.5);
#1019=VECTOR('',#3546,105.5);
#1020=VECTOR('',#3549,105.5);
#1021=VECTOR('',#3552,105.5);
#1022=VECTOR('',#3555,105.5);
#1023=VECTOR('',#3558,105.5);
#1024=VECTOR('',#3561,105.5);
#1025=VECTOR('',#3564,105.5);
#1026=VECTOR('',#3567,105.5);
#1027=VECTOR('',#3570,105.5);
#1028=VECTOR('',#3573,105.5);
#1029=VECTOR('',#3576,105.5);
#1030=VECTOR('',#3579,105.5);
#1031=VECTOR('',#3584,105.5);
#1032=VECTOR('',#3585,105.5);
#1033=VECTOR('',#3586,0.874999997268811);
#1034=VECTOR('',#3593,120.5);
#1035=VECTOR('',#3616,118.168461709225);
#1036=VECTOR('',#3619,0.624999997268823);
#1037=VECTOR('',#3620,0.624999997268819);
#1038=VECTOR('',#3623,0.624999997268823);
#1039=VECTOR('',#3624,0.624999997268822);
#1040=VECTOR('',#3625,0.874999997268824);
#1041=VECTOR('',#3632,9.99999999999999);
#1042=VECTOR('',#3639,9.99999999999999);
#1043=VECTOR('',#3646,114.797295826488);
#1044=VECTOR('',#3649,120.5);
#1082=VERTEX_POINT('',#3909);
#1083=VERTEX_POINT('',#3910);
#1084=VERTEX_POINT('',#3912);
#1085=VERTEX_POINT('',#3922);
#1086=VERTEX_POINT('',#3934);
#1087=VERTEX_POINT('',#3935);
#1088=VERTEX_POINT('',#3972);
#1089=VERTEX_POINT('',#3973);
#1090=VERTEX_POINT('',#4010);
#1091=VERTEX_POINT('',#4011);
#1092=VERTEX_POINT('',#4048);
#1093=VERTEX_POINT('',#4049);
#1094=VERTEX_POINT('',#4086);
#1095=VERTEX_POINT('',#4087);
#1096=VERTEX_POINT('',#4124);
#1097=VERTEX_POINT('',#4125);
#1098=VERTEX_POINT('',#4162);
#1099=VERTEX_POINT('',#4163);
#1100=VERTEX_POINT('',#4200);
#1101=VERTEX_POINT('',#4201);
#1102=VERTEX_POINT('',#4238);
#1103=VERTEX_POINT('',#4239);
#1104=VERTEX_POINT('',#4276);
#1105=VERTEX_POINT('',#4277);
#1106=VERTEX_POINT('',#4314);
#1107=VERTEX_POINT('',#4315);
#1108=VERTEX_POINT('',#4352);
#1109=VERTEX_POINT('',#4353);
#1110=VERTEX_POINT('',#4390);
#1111=VERTEX_POINT('',#4391);
#1112=VERTEX_POINT('',#4428);
#1113=VERTEX_POINT('',#4429);
#1114=VERTEX_POINT('',#4466);
#1115=VERTEX_POINT('',#4467);
#1116=VERTEX_POINT('',#4504);
#1117=VERTEX_POINT('',#4505);
#1118=VERTEX_POINT('',#4542);
#1119=VERTEX_POINT('',#4543);
#1120=VERTEX_POINT('',#4580);
#1121=VERTEX_POINT('',#4581);
#1122=VERTEX_POINT('',#4618);
#1123=VERTEX_POINT('',#4619);
#1124=VERTEX_POINT('',#4656);
#1125=VERTEX_POINT('',#4657);
#1126=VERTEX_POINT('',#4694);
#1127=VERTEX_POINT('',#4695);
#1128=VERTEX_POINT('',#4732);
#1129=VERTEX_POINT('',#4733);
#1130=VERTEX_POINT('',#4770);
#1131=VERTEX_POINT('',#4771);
#1132=VERTEX_POINT('',#4808);
#1133=VERTEX_POINT('',#4809);
#1134=VERTEX_POINT('',#4846);
#1135=VERTEX_POINT('',#4847);
#1136=VERTEX_POINT('',#4884);
#1137=VERTEX_POINT('',#4885);
#1138=VERTEX_POINT('',#4922);
#1139=VERTEX_POINT('',#4923);
#1140=VERTEX_POINT('',#4960);
#1141=VERTEX_POINT('',#4961);
#1142=VERTEX_POINT('',#4998);
#1143=VERTEX_POINT('',#4999);
#1144=VERTEX_POINT('',#5036);
#1145=VERTEX_POINT('',#5037);
#1146=VERTEX_POINT('',#5074);
#1147=VERTEX_POINT('',#5075);
#1148=VERTEX_POINT('',#5112);
#1149=VERTEX_POINT('',#5113);
#1150=VERTEX_POINT('',#5150);
#1151=VERTEX_POINT('',#5151);
#1152=VERTEX_POINT('',#5188);
#1153=VERTEX_POINT('',#5189);
#1154=VERTEX_POINT('',#5226);
#1155=VERTEX_POINT('',#5227);
#1156=VERTEX_POINT('',#5264);
#1157=VERTEX_POINT('',#5265);
#1158=VERTEX_POINT('',#5302);
#1159=VERTEX_POINT('',#5303);
#1160=VERTEX_POINT('',#5340);
#1161=VERTEX_POINT('',#5341);
#1162=VERTEX_POINT('',#5378);
#1163=VERTEX_POINT('',#5379);
#1164=VERTEX_POINT('',#5416);
#1165=VERTEX_POINT('',#5417);
#1166=VERTEX_POINT('',#5454);
#1167=VERTEX_POINT('',#5455);
#1168=VERTEX_POINT('',#5492);
#1169=VERTEX_POINT('',#5493);
#1170=VERTEX_POINT('',#5530);
#1171=VERTEX_POINT('',#5531);
#1172=VERTEX_POINT('',#5568);
#1173=VERTEX_POINT('',#5569);
#1174=VERTEX_POINT('',#5606);
#1175=VERTEX_POINT('',#5607);
#1176=VERTEX_POINT('',#5644);
#1177=VERTEX_POINT('',#5645);
#1178=VERTEX_POINT('',#5682);
#1179=VERTEX_POINT('',#5683);
#1180=VERTEX_POINT('',#5720);
#1181=VERTEX_POINT('',#5721);
#1182=VERTEX_POINT('',#5758);
#1183=VERTEX_POINT('',#5759);
#1184=VERTEX_POINT('',#5761);
#1185=VERTEX_POINT('',#5771);
#1186=VERTEX_POINT('',#5783);
#1187=VERTEX_POINT('',#5784);
#1188=VERTEX_POINT('',#5786);
#1189=VERTEX_POINT('',#5792);
#1190=VERTEX_POINT('',#5802);
#1191=VERTEX_POINT('',#5803);
#1192=VERTEX_POINT('',#5840);
#1193=VERTEX_POINT('',#5841);
#1194=VERTEX_POINT('',#5878);
#1195=VERTEX_POINT('',#5879);
#1196=VERTEX_POINT('',#5916);
#1197=VERTEX_POINT('',#5917);
#1198=VERTEX_POINT('',#5954);
#1199=VERTEX_POINT('',#5955);
#1200=VERTEX_POINT('',#5992);
#1201=VERTEX_POINT('',#5993);
#1202=VERTEX_POINT('',#6030);
#1203=VERTEX_POINT('',#6031);
#1204=VERTEX_POINT('',#6068);
#1205=VERTEX_POINT('',#6069);
#1206=VERTEX_POINT('',#6106);
#1207=VERTEX_POINT('',#6107);
#1208=VERTEX_POINT('',#6144);
#1209=VERTEX_POINT('',#6145);
#1210=VERTEX_POINT('',#6182);
#1211=VERTEX_POINT('',#6183);
#1212=VERTEX_POINT('',#6220);
#1213=VERTEX_POINT('',#6221);
#1214=VERTEX_POINT('',#6258);
#1215=VERTEX_POINT('',#6259);
#1216=VERTEX_POINT('',#6296);
#1217=VERTEX_POINT('',#6297);
#1218=VERTEX_POINT('',#6334);
#1219=VERTEX_POINT('',#6335);
#1220=VERTEX_POINT('',#6372);
#1221=VERTEX_POINT('',#6373);
#1222=VERTEX_POINT('',#6410);
#1223=VERTEX_POINT('',#6411);
#1224=VERTEX_POINT('',#6448);
#1225=VERTEX_POINT('',#6449);
#1226=VERTEX_POINT('',#6486);
#1227=VERTEX_POINT('',#6487);
#1228=VERTEX_POINT('',#6524);
#1229=VERTEX_POINT('',#6525);
#1230=VERTEX_POINT('',#6562);
#1231=VERTEX_POINT('',#6563);
#1232=VERTEX_POINT('',#6600);
#1233=VERTEX_POINT('',#6601);
#1234=VERTEX_POINT('',#6638);
#1235=VERTEX_POINT('',#6639);
#1236=VERTEX_POINT('',#6676);
#1237=VERTEX_POINT('',#6677);
#1238=VERTEX_POINT('',#6714);
#1239=VERTEX_POINT('',#6715);
#1240=VERTEX_POINT('',#6752);
#1241=VERTEX_POINT('',#6753);
#1242=VERTEX_POINT('',#6790);
#1243=VERTEX_POINT('',#6791);
#1244=VERTEX_POINT('',#6828);
#1245=VERTEX_POINT('',#6829);
#1246=VERTEX_POINT('',#6866);
#1247=VERTEX_POINT('',#6867);
#1248=VERTEX_POINT('',#6904);
#1249=VERTEX_POINT('',#6905);
#1250=VERTEX_POINT('',#6942);
#1251=VERTEX_POINT('',#6943);
#1252=VERTEX_POINT('',#6980);
#1253=VERTEX_POINT('',#6981);
#1254=VERTEX_POINT('',#7018);
#1255=VERTEX_POINT('',#7019);
#1256=VERTEX_POINT('',#7056);
#1257=VERTEX_POINT('',#7057);
#1258=VERTEX_POINT('',#7094);
#1259=VERTEX_POINT('',#7095);
#1260=VERTEX_POINT('',#7132);
#1261=VERTEX_POINT('',#7133);
#1262=VERTEX_POINT('',#7170);
#1263=VERTEX_POINT('',#7171);
#1264=VERTEX_POINT('',#7208);
#1265=VERTEX_POINT('',#7209);
#1266=VERTEX_POINT('',#7246);
#1267=VERTEX_POINT('',#7247);
#1268=VERTEX_POINT('',#7284);
#1269=VERTEX_POINT('',#7285);
#1270=VERTEX_POINT('',#7322);
#1271=VERTEX_POINT('',#7323);
#1272=VERTEX_POINT('',#7360);
#1273=VERTEX_POINT('',#7361);
#1274=VERTEX_POINT('',#7398);
#1275=VERTEX_POINT('',#7399);
#1276=VERTEX_POINT('',#7436);
#1277=VERTEX_POINT('',#7437);
#1278=VERTEX_POINT('',#7474);
#1279=VERTEX_POINT('',#7475);
#1280=VERTEX_POINT('',#7512);
#1281=VERTEX_POINT('',#7513);
#1282=VERTEX_POINT('',#7550);
#1283=VERTEX_POINT('',#7551);
#1284=VERTEX_POINT('',#7588);
#1285=VERTEX_POINT('',#7590);
#1286=VERTEX_POINT('',#7592);
#1287=VERTEX_POINT('',#7610);
#1288=VERTEX_POINT('',#7612);
#1289=VERTEX_POINT('',#7626);
#1290=VERTEX_POINT('',#7642);
#1291=VERTEX_POINT('',#7643);
#1292=VERTEX_POINT('',#7646);
#1293=VERTEX_POINT('',#7649);
#1294=VERTEX_POINT('',#7650);
#1295=VERTEX_POINT('',#7687);
#1296=VERTEX_POINT('',#7688);
#1297=VERTEX_POINT('',#7761);
#1298=VERTEX_POINT('',#7763);
#1299=VERTEX_POINT('',#7766);
#1300=VERTEX_POINT('',#7770);
#1301=VERTEX_POINT('',#7779);
#1302=VERTEX_POINT('',#11038);
#1303=VERTEX_POINT('',#11043);
#1370=EDGE_CURVE('',#1082,#1083,#780,.T.);
#1371=EDGE_CURVE('',#1083,#1084,#570,.T.);
#1372=EDGE_CURVE('',#1085,#1084,#781,.T.);
#1373=EDGE_CURVE('',#1082,#1085,#571,.T.);
#1374=EDGE_CURVE('',#1086,#1087,#782,.T.);
#1375=EDGE_CURVE('',#1087,#1083,#572,.T.);
#1376=EDGE_CURVE('',#1086,#1082,#573,.T.);
#1377=EDGE_CURVE('',#1088,#1089,#783,.T.);
#1378=EDGE_CURVE('',#1089,#1087,#574,.T.);
#1379=EDGE_CURVE('',#1088,#1086,#575,.T.);
#1380=EDGE_CURVE('',#1090,#1091,#784,.T.);
#1381=EDGE_CURVE('',#1091,#1089,#576,.T.);
#1382=EDGE_CURVE('',#1090,#1088,#577,.T.);
#1383=EDGE_CURVE('',#1092,#1093,#785,.T.);
#1384=EDGE_CURVE('',#1093,#1091,#578,.T.);
#1385=EDGE_CURVE('',#1092,#1090,#579,.T.);
#1386=EDGE_CURVE('',#1094,#1095,#786,.T.);
#1387=EDGE_CURVE('',#1095,#1093,#580,.T.);
#1388=EDGE_CURVE('',#1094,#1092,#581,.T.);
#1389=EDGE_CURVE('',#1096,#1097,#787,.T.);
#1390=EDGE_CURVE('',#1097,#1095,#582,.T.);
#1391=EDGE_CURVE('',#1096,#1094,#583,.T.);
#1392=EDGE_CURVE('',#1098,#1099,#788,.T.);
#1393=EDGE_CURVE('',#1099,#1097,#584,.T.);
#1394=EDGE_CURVE('',#1098,#1096,#585,.T.);
#1395=EDGE_CURVE('',#1100,#1101,#789,.T.);
#1396=EDGE_CURVE('',#1101,#1099,#586,.T.);
#1397=EDGE_CURVE('',#1100,#1098,#587,.T.);
#1398=EDGE_CURVE('',#1102,#1103,#790,.T.);
#1399=EDGE_CURVE('',#1103,#1101,#588,.T.);
#1400=EDGE_CURVE('',#1102,#1100,#589,.T.);
#1401=EDGE_CURVE('',#1104,#1105,#791,.T.);
#1402=EDGE_CURVE('',#1105,#1103,#590,.T.);
#1403=EDGE_CURVE('',#1104,#1102,#591,.T.);
#1404=EDGE_CURVE('',#1106,#1107,#792,.T.);
#1405=EDGE_CURVE('',#1107,#1105,#592,.T.);
#1406=EDGE_CURVE('',#1106,#1104,#593,.T.);
#1407=EDGE_CURVE('',#1108,#1109,#793,.T.);
#1408=EDGE_CURVE('',#1109,#1107,#594,.T.);
#1409=EDGE_CURVE('',#1108,#1106,#595,.T.);
#1410=EDGE_CURVE('',#1110,#1111,#794,.T.);
#1411=EDGE_CURVE('',#1111,#1109,#596,.T.);
#1412=EDGE_CURVE('',#1110,#1108,#597,.T.);
#1413=EDGE_CURVE('',#1112,#1113,#795,.T.);
#1414=EDGE_CURVE('',#1113,#1111,#598,.T.);
#1415=EDGE_CURVE('',#1112,#1110,#599,.T.);
#1416=EDGE_CURVE('',#1114,#1115,#796,.T.);
#1417=EDGE_CURVE('',#1115,#1113,#600,.T.);
#1418=EDGE_CURVE('',#1114,#1112,#601,.T.);
#1419=EDGE_CURVE('',#1116,#1117,#797,.T.);
#1420=EDGE_CURVE('',#1117,#1115,#602,.T.);
#1421=EDGE_CURVE('',#1116,#1114,#603,.T.);
#1422=EDGE_CURVE('',#1118,#1119,#798,.T.);
#1423=EDGE_CURVE('',#1119,#1117,#604,.T.);
#1424=EDGE_CURVE('',#1118,#1116,#605,.T.);
#1425=EDGE_CURVE('',#1120,#1121,#799,.T.);
#1426=EDGE_CURVE('',#1121,#1119,#606,.T.);
#1427=EDGE_CURVE('',#1120,#1118,#607,.T.);
#1428=EDGE_CURVE('',#1122,#1123,#800,.T.);
#1429=EDGE_CURVE('',#1123,#1121,#608,.T.);
#1430=EDGE_CURVE('',#1122,#1120,#609,.T.);
#1431=EDGE_CURVE('',#1124,#1125,#801,.T.);
#1432=EDGE_CURVE('',#1125,#1123,#610,.T.);
#1433=EDGE_CURVE('',#1124,#1122,#611,.T.);
#1434=EDGE_CURVE('',#1126,#1127,#802,.T.);
#1435=EDGE_CURVE('',#1127,#1125,#612,.T.);
#1436=EDGE_CURVE('',#1126,#1124,#613,.T.);
#1437=EDGE_CURVE('',#1128,#1129,#803,.T.);
#1438=EDGE_CURVE('',#1129,#1127,#614,.T.);
#1439=EDGE_CURVE('',#1128,#1126,#615,.T.);
#1440=EDGE_CURVE('',#1130,#1131,#804,.T.);
#1441=EDGE_CURVE('',#1131,#1129,#616,.T.);
#1442=EDGE_CURVE('',#1130,#1128,#617,.T.);
#1443=EDGE_CURVE('',#1132,#1133,#805,.T.);
#1444=EDGE_CURVE('',#1133,#1131,#618,.T.);
#1445=EDGE_CURVE('',#1132,#1130,#619,.T.);
#1446=EDGE_CURVE('',#1134,#1135,#806,.T.);
#1447=EDGE_CURVE('',#1135,#1133,#620,.T.);
#1448=EDGE_CURVE('',#1134,#1132,#621,.T.);
#1449=EDGE_CURVE('',#1136,#1137,#807,.T.);
#1450=EDGE_CURVE('',#1137,#1135,#622,.T.);
#1451=EDGE_CURVE('',#1136,#1134,#623,.T.);
#1452=EDGE_CURVE('',#1138,#1139,#808,.T.);
#1453=EDGE_CURVE('',#1139,#1137,#624,.T.);
#1454=EDGE_CURVE('',#1138,#1136,#625,.T.);
#1455=EDGE_CURVE('',#1140,#1141,#809,.T.);
#1456=EDGE_CURVE('',#1141,#1139,#626,.T.);
#1457=EDGE_CURVE('',#1140,#1138,#627,.T.);
#1458=EDGE_CURVE('',#1142,#1143,#810,.T.);
#1459=EDGE_CURVE('',#1143,#1141,#628,.T.);
#1460=EDGE_CURVE('',#1142,#1140,#629,.T.);
#1461=EDGE_CURVE('',#1144,#1145,#811,.T.);
#1462=EDGE_CURVE('',#1145,#1143,#630,.T.);
#1463=EDGE_CURVE('',#1144,#1142,#631,.T.);
#1464=EDGE_CURVE('',#1146,#1147,#812,.T.);
#1465=EDGE_CURVE('',#1147,#1145,#632,.T.);
#1466=EDGE_CURVE('',#1146,#1144,#633,.T.);
#1467=EDGE_CURVE('',#1148,#1149,#813,.T.);
#1468=EDGE_CURVE('',#1149,#1147,#634,.T.);
#1469=EDGE_CURVE('',#1148,#1146,#635,.T.);
#1470=EDGE_CURVE('',#1150,#1151,#814,.T.);
#1471=EDGE_CURVE('',#1151,#1149,#636,.T.);
#1472=EDGE_CURVE('',#1150,#1148,#637,.T.);
#1473=EDGE_CURVE('',#1152,#1153,#815,.T.);
#1474=EDGE_CURVE('',#1153,#1151,#638,.T.);
#1475=EDGE_CURVE('',#1152,#1150,#639,.T.);
#1476=EDGE_CURVE('',#1154,#1155,#816,.T.);
#1477=EDGE_CURVE('',#1155,#1153,#640,.T.);
#1478=EDGE_CURVE('',#1154,#1152,#641,.T.);
#1479=EDGE_CURVE('',#1156,#1157,#817,.T.);
#1480=EDGE_CURVE('',#1157,#1155,#642,.T.);
#1481=EDGE_CURVE('',#1156,#1154,#643,.T.);
#1482=EDGE_CURVE('',#1158,#1159,#818,.T.);
#1483=EDGE_CURVE('',#1159,#1157,#644,.T.);
#1484=EDGE_CURVE('',#1158,#1156,#645,.T.);
#1485=EDGE_CURVE('',#1160,#1161,#819,.T.);
#1486=EDGE_CURVE('',#1161,#1159,#646,.T.);
#1487=EDGE_CURVE('',#1160,#1158,#647,.T.);
#1488=EDGE_CURVE('',#1162,#1163,#820,.T.);
#1489=EDGE_CURVE('',#1163,#1161,#648,.T.);
#1490=EDGE_CURVE('',#1162,#1160,#649,.T.);
#1491=EDGE_CURVE('',#1164,#1165,#821,.T.);
#1492=EDGE_CURVE('',#1165,#1163,#650,.T.);
#1493=EDGE_CURVE('',#1164,#1162,#651,.T.);
#1494=EDGE_CURVE('',#1166,#1167,#822,.T.);
#1495=EDGE_CURVE('',#1167,#1165,#652,.T.);
#1496=EDGE_CURVE('',#1166,#1164,#653,.T.);
#1497=EDGE_CURVE('',#1168,#1169,#823,.T.);
#1498=EDGE_CURVE('',#1169,#1167,#654,.T.);
#1499=EDGE_CURVE('',#1168,#1166,#655,.T.);
#1500=EDGE_CURVE('',#1170,#1171,#824,.T.);
#1501=EDGE_CURVE('',#1171,#1169,#656,.T.);
#1502=EDGE_CURVE('',#1170,#1168,#657,.T.);
#1503=EDGE_CURVE('',#1172,#1173,#825,.T.);
#1504=EDGE_CURVE('',#1173,#1171,#658,.T.);
#1505=EDGE_CURVE('',#1172,#1170,#659,.T.);
#1506=EDGE_CURVE('',#1174,#1175,#826,.T.);
#1507=EDGE_CURVE('',#1175,#1173,#660,.T.);
#1508=EDGE_CURVE('',#1174,#1172,#661,.T.);
#1509=EDGE_CURVE('',#1176,#1177,#827,.T.);
#1510=EDGE_CURVE('',#1177,#1175,#662,.T.);
#1511=EDGE_CURVE('',#1176,#1174,#663,.T.);
#1512=EDGE_CURVE('',#1178,#1179,#828,.T.);
#1513=EDGE_CURVE('',#1179,#1177,#664,.T.);
#1514=EDGE_CURVE('',#1178,#1176,#665,.T.);
#1515=EDGE_CURVE('',#1180,#1181,#829,.T.);
#1516=EDGE_CURVE('',#1181,#1179,#666,.T.);
#1517=EDGE_CURVE('',#1180,#1178,#667,.T.);
#1518=EDGE_CURVE('',#1182,#1183,#830,.T.);
#1519=EDGE_CURVE('',#1184,#1182,#668,.T.);
#1520=EDGE_CURVE('',#1185,#1184,#831,.T.);
#1521=EDGE_CURVE('',#1185,#1183,#669,.T.);
#1522=EDGE_CURVE('',#1186,#1187,#832,.T.);
#1523=EDGE_CURVE('',#1187,#1188,#670,.T.);
#1524=EDGE_CURVE('',#1189,#1188,#149,.T.);
#1525=EDGE_CURVE('',#1186,#1189,#671,.T.);
#1526=EDGE_CURVE('',#1190,#1191,#833,.T.);
#1527=EDGE_CURVE('',#1191,#1187,#672,.T.);
#1528=EDGE_CURVE('',#1190,#1186,#673,.T.);
#1529=EDGE_CURVE('',#1192,#1193,#834,.T.);
#1530=EDGE_CURVE('',#1193,#1191,#674,.T.);
#1531=EDGE_CURVE('',#1192,#1190,#675,.T.);
#1532=EDGE_CURVE('',#1194,#1195,#835,.T.);
#1533=EDGE_CURVE('',#1195,#1193,#676,.T.);
#1534=EDGE_CURVE('',#1194,#1192,#677,.T.);
#1535=EDGE_CURVE('',#1196,#1197,#836,.T.);
#1536=EDGE_CURVE('',#1197,#1195,#678,.T.);
#1537=EDGE_CURVE('',#1196,#1194,#679,.T.);
#1538=EDGE_CURVE('',#1198,#1199,#837,.T.);
#1539=EDGE_CURVE('',#1199,#1197,#680,.T.);
#1540=EDGE_CURVE('',#1198,#1196,#681,.T.);
#1541=EDGE_CURVE('',#1200,#1201,#838,.T.);
#1542=EDGE_CURVE('',#1201,#1199,#682,.T.);
#1543=EDGE_CURVE('',#1200,#1198,#683,.T.);
#1544=EDGE_CURVE('',#1202,#1203,#839,.T.);
#1545=EDGE_CURVE('',#1203,#1201,#684,.T.);
#1546=EDGE_CURVE('',#1202,#1200,#685,.T.);
#1547=EDGE_CURVE('',#1204,#1205,#840,.T.);
#1548=EDGE_CURVE('',#1205,#1203,#686,.T.);
#1549=EDGE_CURVE('',#1204,#1202,#687,.T.);
#1550=EDGE_CURVE('',#1206,#1207,#841,.T.);
#1551=EDGE_CURVE('',#1207,#1205,#688,.T.);
#1552=EDGE_CURVE('',#1206,#1204,#689,.T.);
#1553=EDGE_CURVE('',#1208,#1209,#842,.T.);
#1554=EDGE_CURVE('',#1209,#1207,#690,.T.);
#1555=EDGE_CURVE('',#1208,#1206,#691,.T.);
#1556=EDGE_CURVE('',#1210,#1211,#843,.T.);
#1557=EDGE_CURVE('',#1211,#1209,#692,.T.);
#1558=EDGE_CURVE('',#1210,#1208,#693,.T.);
#1559=EDGE_CURVE('',#1212,#1213,#844,.T.);
#1560=EDGE_CURVE('',#1213,#1211,#694,.T.);
#1561=EDGE_CURVE('',#1212,#1210,#695,.T.);
#1562=EDGE_CURVE('',#1214,#1215,#845,.T.);
#1563=EDGE_CURVE('',#1215,#1213,#696,.T.);
#1564=EDGE_CURVE('',#1214,#1212,#697,.T.);
#1565=EDGE_CURVE('',#1216,#1217,#846,.T.);
#1566=EDGE_CURVE('',#1217,#1215,#698,.T.);
#1567=EDGE_CURVE('',#1216,#1214,#699,.T.);
#1568=EDGE_CURVE('',#1218,#1219,#847,.T.);
#1569=EDGE_CURVE('',#1219,#1217,#700,.T.);
#1570=EDGE_CURVE('',#1218,#1216,#701,.T.);
#1571=EDGE_CURVE('',#1220,#1221,#848,.T.);
#1572=EDGE_CURVE('',#1221,#1219,#702,.T.);
#1573=EDGE_CURVE('',#1220,#1218,#703,.T.);
#1574=EDGE_CURVE('',#1222,#1223,#849,.T.);
#1575=EDGE_CURVE('',#1223,#1221,#704,.T.);
#1576=EDGE_CURVE('',#1222,#1220,#705,.T.);
#1577=EDGE_CURVE('',#1224,#1225,#850,.T.);
#1578=EDGE_CURVE('',#1225,#1223,#706,.T.);
#1579=EDGE_CURVE('',#1224,#1222,#707,.T.);
#1580=EDGE_CURVE('',#1226,#1227,#851,.T.);
#1581=EDGE_CURVE('',#1227,#1225,#708,.T.);
#1582=EDGE_CURVE('',#1226,#1224,#709,.T.);
#1583=EDGE_CURVE('',#1228,#1229,#852,.T.);
#1584=EDGE_CURVE('',#1229,#1227,#710,.T.);
#1585=EDGE_CURVE('',#1228,#1226,#711,.T.);
#1586=EDGE_CURVE('',#1230,#1231,#853,.T.);
#1587=EDGE_CURVE('',#1231,#1229,#712,.T.);
#1588=EDGE_CURVE('',#1230,#1228,#713,.T.);
#1589=EDGE_CURVE('',#1232,#1233,#854,.T.);
#1590=EDGE_CURVE('',#1233,#1231,#714,.T.);
#1591=EDGE_CURVE('',#1232,#1230,#715,.T.);
#1592=EDGE_CURVE('',#1234,#1235,#855,.T.);
#1593=EDGE_CURVE('',#1235,#1233,#716,.T.);
#1594=EDGE_CURVE('',#1234,#1232,#717,.T.);
#1595=EDGE_CURVE('',#1236,#1237,#856,.T.);
#1596=EDGE_CURVE('',#1237,#1235,#718,.T.);
#1597=EDGE_CURVE('',#1236,#1234,#719,.T.);
#1598=EDGE_CURVE('',#1238,#1239,#857,.T.);
#1599=EDGE_CURVE('',#1239,#1237,#720,.T.);
#1600=EDGE_CURVE('',#1238,#1236,#721,.T.);
#1601=EDGE_CURVE('',#1240,#1241,#858,.T.);
#1602=EDGE_CURVE('',#1241,#1239,#722,.T.);
#1603=EDGE_CURVE('',#1240,#1238,#723,.T.);
#1604=EDGE_CURVE('',#1242,#1243,#859,.T.);
#1605=EDGE_CURVE('',#1243,#1241,#724,.T.);
#1606=EDGE_CURVE('',#1242,#1240,#725,.T.);
#1607=EDGE_CURVE('',#1244,#1245,#860,.T.);
#1608=EDGE_CURVE('',#1245,#1243,#726,.T.);
#1609=EDGE_CURVE('',#1244,#1242,#727,.T.);
#1610=EDGE_CURVE('',#1246,#1247,#861,.T.);
#1611=EDGE_CURVE('',#1247,#1245,#728,.T.);
#1612=EDGE_CURVE('',#1246,#1244,#729,.T.);
#1613=EDGE_CURVE('',#1248,#1249,#862,.T.);
#1614=EDGE_CURVE('',#1249,#1247,#730,.T.);
#1615=EDGE_CURVE('',#1248,#1246,#731,.T.);
#1616=EDGE_CURVE('',#1250,#1251,#863,.T.);
#1617=EDGE_CURVE('',#1251,#1249,#732,.T.);
#1618=EDGE_CURVE('',#1250,#1248,#733,.T.);
#1619=EDGE_CURVE('',#1252,#1253,#864,.T.);
#1620=EDGE_CURVE('',#1253,#1251,#734,.T.);
#1621=EDGE_CURVE('',#1252,#1250,#735,.T.);
#1622=EDGE_CURVE('',#1254,#1255,#865,.T.);
#1623=EDGE_CURVE('',#1255,#1253,#736,.T.);
#1624=EDGE_CURVE('',#1254,#1252,#737,.T.);
#1625=EDGE_CURVE('',#1256,#1257,#866,.T.);
#1626=EDGE_CURVE('',#1257,#1255,#738,.T.);
#1627=EDGE_CURVE('',#1256,#1254,#739,.T.);
#1628=EDGE_CURVE('',#1258,#1259,#867,.T.);
#1629=EDGE_CURVE('',#1259,#1257,#740,.T.);
#1630=EDGE_CURVE('',#1258,#1256,#741,.T.);
#1631=EDGE_CURVE('',#1260,#1261,#868,.T.);
#1632=EDGE_CURVE('',#1261,#1259,#742,.T.);
#1633=EDGE_CURVE('',#1260,#1258,#743,.T.);
#1634=EDGE_CURVE('',#1262,#1263,#869,.T.);
#1635=EDGE_CURVE('',#1263,#1261,#744,.T.);
#1636=EDGE_CURVE('',#1262,#1260,#745,.T.);
#1637=EDGE_CURVE('',#1264,#1265,#870,.T.);
#1638=EDGE_CURVE('',#1265,#1263,#746,.T.);
#1639=EDGE_CURVE('',#1264,#1262,#747,.T.);
#1640=EDGE_CURVE('',#1266,#1267,#871,.T.);
#1641=EDGE_CURVE('',#1267,#1265,#748,.T.);
#1642=EDGE_CURVE('',#1266,#1264,#749,.T.);
#1643=EDGE_CURVE('',#1268,#1269,#872,.T.);
#1644=EDGE_CURVE('',#1269,#1267,#750,.T.);
#1645=EDGE_CURVE('',#1268,#1266,#751,.T.);
#1646=EDGE_CURVE('',#1270,#1271,#873,.T.);
#1647=EDGE_CURVE('',#1271,#1269,#752,.T.);
#1648=EDGE_CURVE('',#1270,#1268,#753,.T.);
#1649=EDGE_CURVE('',#1272,#1273,#874,.T.);
#1650=EDGE_CURVE('',#1273,#1271,#754,.T.);
#1651=EDGE_CURVE('',#1272,#1270,#755,.T.);
#1652=EDGE_CURVE('',#1274,#1275,#875,.T.);
#1653=EDGE_CURVE('',#1275,#1273,#756,.T.);
#1654=EDGE_CURVE('',#1274,#1272,#757,.T.);
#1655=EDGE_CURVE('',#1276,#1277,#876,.T.);
#1656=EDGE_CURVE('',#1277,#1275,#758,.T.);
#1657=EDGE_CURVE('',#1276,#1274,#759,.T.);
#1658=EDGE_CURVE('',#1278,#1279,#877,.T.);
#1659=EDGE_CURVE('',#1279,#1277,#760,.T.);
#1660=EDGE_CURVE('',#1278,#1276,#761,.T.);
#1661=EDGE_CURVE('',#1280,#1281,#878,.T.);
#1662=EDGE_CURVE('',#1281,#1279,#762,.T.);
#1663=EDGE_CURVE('',#1280,#1278,#763,.T.);
#1664=EDGE_CURVE('',#1282,#1283,#879,.T.);
#1665=EDGE_CURVE('',#1283,#1281,#764,.T.);
#1666=EDGE_CURVE('',#1282,#1280,#765,.T.);
#1667=EDGE_CURVE('',#1284,#1284,#150,.T.);
#1668=EDGE_CURVE('',#1284,#1285,#880,.T.);
#1669=EDGE_CURVE('',#1285,#1286,#766,.T.);
#1670=EDGE_CURVE('',#1287,#1286,#881,.T.);
#1671=EDGE_CURVE('',#1288,#1287,#767,.T.);
#1672=EDGE_CURVE('',#1289,#1288,#882,.T.);
#1673=EDGE_CURVE('',#1289,#1285,#768,.T.);
#1674=EDGE_CURVE('',#1290,#1291,#151,.T.);
#1675=EDGE_CURVE('',#1291,#1290,#152,.T.);
#1676=EDGE_CURVE('',#1290,#1292,#883,.T.);
#1677=EDGE_CURVE('',#1292,#1292,#153,.F.);
#1678=EDGE_CURVE('',#1293,#1294,#135,.T.);
#1679=EDGE_CURVE('',#1294,#1293,#136,.T.);
#1680=EDGE_CURVE('',#1295,#1296,#137,.T.);
#1681=EDGE_CURVE('',#1296,#1295,#138,.T.);
#1682=EDGE_CURVE('',#1286,#1283,#769,.T.);
#1683=EDGE_CURVE('',#1287,#1282,#770,.T.);
#1684=EDGE_CURVE('',#1297,#1297,#154,.T.);
#1685=EDGE_CURVE('',#1298,#1298,#155,.T.);
#1686=EDGE_CURVE('',#1299,#1299,#156,.F.);
#1687=EDGE_CURVE('',#1188,#1189,#157,.T.);
#1688=EDGE_CURVE('',#1300,#1300,#158,.T.);
#1689=EDGE_CURVE('',#1292,#1297,#884,.T.);
#1690=EDGE_CURVE('',#1184,#1289,#885,.T.);
#1691=EDGE_CURVE('',#1288,#1185,#886,.T.);
#1692=EDGE_CURVE('',#1188,#1085,#887,.T.);
#1693=EDGE_CURVE('',#1084,#1301,#888,.T.);
#1694=EDGE_CURVE('',#1301,#1188,#889,.T.);
#1695=EDGE_CURVE('',#1182,#1180,#771,.T.);
#1696=EDGE_CURVE('',#1183,#1181,#772,.T.);
#1697=EDGE_CURVE('',#1189,#1301,#773,.T.);
#1698=EDGE_CURVE('',#1294,#1302,#890,.T.);
#1699=EDGE_CURVE('',#1302,#1302,#159,.T.);
#1700=EDGE_CURVE('',#1296,#1303,#891,.T.);
#1701=EDGE_CURVE('',#1303,#1303,#160,.T.);
#1702=EDGE_CURVE('',#1300,#1298,#892,.T.);
#1703=EDGE_CURVE('',#1291,#1299,#893,.T.);
#1803=ORIENTED_EDGE('',*,*,#1370,.T.);
#1804=ORIENTED_EDGE('',*,*,#1371,.T.);
#1805=ORIENTED_EDGE('',*,*,#1372,.F.);
#1806=ORIENTED_EDGE('',*,*,#1373,.F.);
#1807=ORIENTED_EDGE('',*,*,#1374,.T.);
#1808=ORIENTED_EDGE('',*,*,#1375,.T.);
#1809=ORIENTED_EDGE('',*,*,#1370,.F.);
#1810=ORIENTED_EDGE('',*,*,#1376,.F.);
#1811=ORIENTED_EDGE('',*,*,#1377,.T.);
#1812=ORIENTED_EDGE('',*,*,#1378,.T.);
#1813=ORIENTED_EDGE('',*,*,#1374,.F.);
#1814=ORIENTED_EDGE('',*,*,#1379,.F.);
#1815=ORIENTED_EDGE('',*,*,#1380,.T.);
#1816=ORIENTED_EDGE('',*,*,#1381,.T.);
#1817=ORIENTED_EDGE('',*,*,#1377,.F.);
#1818=ORIENTED_EDGE('',*,*,#1382,.F.);
#1819=ORIENTED_EDGE('',*,*,#1383,.T.);
#1820=ORIENTED_EDGE('',*,*,#1384,.T.);
#1821=ORIENTED_EDGE('',*,*,#1380,.F.);
#1822=ORIENTED_EDGE('',*,*,#1385,.F.);
#1823=ORIENTED_EDGE('',*,*,#1386,.T.);
#1824=ORIENTED_EDGE('',*,*,#1387,.T.);
#1825=ORIENTED_EDGE('',*,*,#1383,.F.);
#1826=ORIENTED_EDGE('',*,*,#1388,.F.);
#1827=ORIENTED_EDGE('',*,*,#1389,.T.);
#1828=ORIENTED_EDGE('',*,*,#1390,.T.);
#1829=ORIENTED_EDGE('',*,*,#1386,.F.);
#1830=ORIENTED_EDGE('',*,*,#1391,.F.);
#1831=ORIENTED_EDGE('',*,*,#1392,.T.);
#1832=ORIENTED_EDGE('',*,*,#1393,.T.);
#1833=ORIENTED_EDGE('',*,*,#1389,.F.);
#1834=ORIENTED_EDGE('',*,*,#1394,.F.);
#1835=ORIENTED_EDGE('',*,*,#1395,.T.);
#1836=ORIENTED_EDGE('',*,*,#1396,.T.);
#1837=ORIENTED_EDGE('',*,*,#1392,.F.);
#1838=ORIENTED_EDGE('',*,*,#1397,.F.);
#1839=ORIENTED_EDGE('',*,*,#1398,.T.);
#1840=ORIENTED_EDGE('',*,*,#1399,.T.);
#1841=ORIENTED_EDGE('',*,*,#1395,.F.);
#1842=ORIENTED_EDGE('',*,*,#1400,.F.);
#1843=ORIENTED_EDGE('',*,*,#1401,.T.);
#1844=ORIENTED_EDGE('',*,*,#1402,.T.);
#1845=ORIENTED_EDGE('',*,*,#1398,.F.);
#1846=ORIENTED_EDGE('',*,*,#1403,.F.);
#1847=ORIENTED_EDGE('',*,*,#1404,.T.);
#1848=ORIENTED_EDGE('',*,*,#1405,.T.);
#1849=ORIENTED_EDGE('',*,*,#1401,.F.);
#1850=ORIENTED_EDGE('',*,*,#1406,.F.);
#1851=ORIENTED_EDGE('',*,*,#1407,.T.);
#1852=ORIENTED_EDGE('',*,*,#1408,.T.);
#1853=ORIENTED_EDGE('',*,*,#1404,.F.);
#1854=ORIENTED_EDGE('',*,*,#1409,.F.);
#1855=ORIENTED_EDGE('',*,*,#1410,.T.);
#1856=ORIENTED_EDGE('',*,*,#1411,.T.);
#1857=ORIENTED_EDGE('',*,*,#1407,.F.);
#1858=ORIENTED_EDGE('',*,*,#1412,.F.);
#1859=ORIENTED_EDGE('',*,*,#1413,.T.);
#1860=ORIENTED_EDGE('',*,*,#1414,.T.);
#1861=ORIENTED_EDGE('',*,*,#1410,.F.);
#1862=ORIENTED_EDGE('',*,*,#1415,.F.);
#1863=ORIENTED_EDGE('',*,*,#1416,.T.);
#1864=ORIENTED_EDGE('',*,*,#1417,.T.);
#1865=ORIENTED_EDGE('',*,*,#1413,.F.);
#1866=ORIENTED_EDGE('',*,*,#1418,.F.);
#1867=ORIENTED_EDGE('',*,*,#1419,.T.);
#1868=ORIENTED_EDGE('',*,*,#1420,.T.);
#1869=ORIENTED_EDGE('',*,*,#1416,.F.);
#1870=ORIENTED_EDGE('',*,*,#1421,.F.);
#1871=ORIENTED_EDGE('',*,*,#1422,.T.);
#1872=ORIENTED_EDGE('',*,*,#1423,.T.);
#1873=ORIENTED_EDGE('',*,*,#1419,.F.);
#1874=ORIENTED_EDGE('',*,*,#1424,.F.);
#1875=ORIENTED_EDGE('',*,*,#1425,.T.);
#1876=ORIENTED_EDGE('',*,*,#1426,.T.);
#1877=ORIENTED_EDGE('',*,*,#1422,.F.);
#1878=ORIENTED_EDGE('',*,*,#1427,.F.);
#1879=ORIENTED_EDGE('',*,*,#1428,.T.);
#1880=ORIENTED_EDGE('',*,*,#1429,.T.);
#1881=ORIENTED_EDGE('',*,*,#1425,.F.);
#1882=ORIENTED_EDGE('',*,*,#1430,.F.);
#1883=ORIENTED_EDGE('',*,*,#1431,.T.);
#1884=ORIENTED_EDGE('',*,*,#1432,.T.);
#1885=ORIENTED_EDGE('',*,*,#1428,.F.);
#1886=ORIENTED_EDGE('',*,*,#1433,.F.);
#1887=ORIENTED_EDGE('',*,*,#1434,.T.);
#1888=ORIENTED_EDGE('',*,*,#1435,.T.);
#1889=ORIENTED_EDGE('',*,*,#1431,.F.);
#1890=ORIENTED_EDGE('',*,*,#1436,.F.);
#1891=ORIENTED_EDGE('',*,*,#1437,.T.);
#1892=ORIENTED_EDGE('',*,*,#1438,.T.);
#1893=ORIENTED_EDGE('',*,*,#1434,.F.);
#1894=ORIENTED_EDGE('',*,*,#1439,.F.);
#1895=ORIENTED_EDGE('',*,*,#1440,.T.);
#1896=ORIENTED_EDGE('',*,*,#1441,.T.);
#1897=ORIENTED_EDGE('',*,*,#1437,.F.);
#1898=ORIENTED_EDGE('',*,*,#1442,.F.);
#1899=ORIENTED_EDGE('',*,*,#1443,.T.);
#1900=ORIENTED_EDGE('',*,*,#1444,.T.);
#1901=ORIENTED_EDGE('',*,*,#1440,.F.);
#1902=ORIENTED_EDGE('',*,*,#1445,.F.);
#1903=ORIENTED_EDGE('',*,*,#1446,.T.);
#1904=ORIENTED_EDGE('',*,*,#1447,.T.);
#1905=ORIENTED_EDGE('',*,*,#1443,.F.);
#1906=ORIENTED_EDGE('',*,*,#1448,.F.);
#1907=ORIENTED_EDGE('',*,*,#1449,.T.);
#1908=ORIENTED_EDGE('',*,*,#1450,.T.);
#1909=ORIENTED_EDGE('',*,*,#1446,.F.);
#1910=ORIENTED_EDGE('',*,*,#1451,.F.);
#1911=ORIENTED_EDGE('',*,*,#1452,.T.);
#1912=ORIENTED_EDGE('',*,*,#1453,.T.);
#1913=ORIENTED_EDGE('',*,*,#1449,.F.);
#1914=ORIENTED_EDGE('',*,*,#1454,.F.);
#1915=ORIENTED_EDGE('',*,*,#1455,.T.);
#1916=ORIENTED_EDGE('',*,*,#1456,.T.);
#1917=ORIENTED_EDGE('',*,*,#1452,.F.);
#1918=ORIENTED_EDGE('',*,*,#1457,.F.);
#1919=ORIENTED_EDGE('',*,*,#1458,.T.);
#1920=ORIENTED_EDGE('',*,*,#1459,.T.);
#1921=ORIENTED_EDGE('',*,*,#1455,.F.);
#1922=ORIENTED_EDGE('',*,*,#1460,.F.);
#1923=ORIENTED_EDGE('',*,*,#1461,.T.);
#1924=ORIENTED_EDGE('',*,*,#1462,.T.);
#1925=ORIENTED_EDGE('',*,*,#1458,.F.);
#1926=ORIENTED_EDGE('',*,*,#1463,.F.);
#1927=ORIENTED_EDGE('',*,*,#1464,.T.);
#1928=ORIENTED_EDGE('',*,*,#1465,.T.);
#1929=ORIENTED_EDGE('',*,*,#1461,.F.);
#1930=ORIENTED_EDGE('',*,*,#1466,.F.);
#1931=ORIENTED_EDGE('',*,*,#1467,.T.);
#1932=ORIENTED_EDGE('',*,*,#1468,.T.);
#1933=ORIENTED_EDGE('',*,*,#1464,.F.);
#1934=ORIENTED_EDGE('',*,*,#1469,.F.);
#1935=ORIENTED_EDGE('',*,*,#1470,.T.);
#1936=ORIENTED_EDGE('',*,*,#1471,.T.);
#1937=ORIENTED_EDGE('',*,*,#1467,.F.);
#1938=ORIENTED_EDGE('',*,*,#1472,.F.);
#1939=ORIENTED_EDGE('',*,*,#1473,.T.);
#1940=ORIENTED_EDGE('',*,*,#1474,.T.);
#1941=ORIENTED_EDGE('',*,*,#1470,.F.);
#1942=ORIENTED_EDGE('',*,*,#1475,.F.);
#1943=ORIENTED_EDGE('',*,*,#1476,.T.);
#1944=ORIENTED_EDGE('',*,*,#1477,.T.);
#1945=ORIENTED_EDGE('',*,*,#1473,.F.);
#1946=ORIENTED_EDGE('',*,*,#1478,.F.);
#1947=ORIENTED_EDGE('',*,*,#1479,.T.);
#1948=ORIENTED_EDGE('',*,*,#1480,.T.);
#1949=ORIENTED_EDGE('',*,*,#1476,.F.);
#1950=ORIENTED_EDGE('',*,*,#1481,.F.);
#1951=ORIENTED_EDGE('',*,*,#1482,.T.);
#1952=ORIENTED_EDGE('',*,*,#1483,.T.);
#1953=ORIENTED_EDGE('',*,*,#1479,.F.);
#1954=ORIENTED_EDGE('',*,*,#1484,.F.);
#1955=ORIENTED_EDGE('',*,*,#1485,.T.);
#1956=ORIENTED_EDGE('',*,*,#1486,.T.);
#1957=ORIENTED_EDGE('',*,*,#1482,.F.);
#1958=ORIENTED_EDGE('',*,*,#1487,.F.);
#1959=ORIENTED_EDGE('',*,*,#1488,.T.);
#1960=ORIENTED_EDGE('',*,*,#1489,.T.);
#1961=ORIENTED_EDGE('',*,*,#1485,.F.);
#1962=ORIENTED_EDGE('',*,*,#1490,.F.);
#1963=ORIENTED_EDGE('',*,*,#1491,.T.);
#1964=ORIENTED_EDGE('',*,*,#1492,.T.);
#1965=ORIENTED_EDGE('',*,*,#1488,.F.);
#1966=ORIENTED_EDGE('',*,*,#1493,.F.);
#1967=ORIENTED_EDGE('',*,*,#1494,.T.);
#1968=ORIENTED_EDGE('',*,*,#1495,.T.);
#1969=ORIENTED_EDGE('',*,*,#1491,.F.);
#1970=ORIENTED_EDGE('',*,*,#1496,.F.);
#1971=ORIENTED_EDGE('',*,*,#1497,.T.);
#1972=ORIENTED_EDGE('',*,*,#1498,.T.);
#1973=ORIENTED_EDGE('',*,*,#1494,.F.);
#1974=ORIENTED_EDGE('',*,*,#1499,.F.);
#1975=ORIENTED_EDGE('',*,*,#1500,.T.);
#1976=ORIENTED_EDGE('',*,*,#1501,.T.);
#1977=ORIENTED_EDGE('',*,*,#1497,.F.);
#1978=ORIENTED_EDGE('',*,*,#1502,.F.);
#1979=ORIENTED_EDGE('',*,*,#1503,.T.);
#1980=ORIENTED_EDGE('',*,*,#1504,.T.);
#1981=ORIENTED_EDGE('',*,*,#1500,.F.);
#1982=ORIENTED_EDGE('',*,*,#1505,.F.);
#1983=ORIENTED_EDGE('',*,*,#1506,.T.);
#1984=ORIENTED_EDGE('',*,*,#1507,.T.);
#1985=ORIENTED_EDGE('',*,*,#1503,.F.);
#1986=ORIENTED_EDGE('',*,*,#1508,.F.);
#1987=ORIENTED_EDGE('',*,*,#1509,.T.);
#1988=ORIENTED_EDGE('',*,*,#1510,.T.);
#1989=ORIENTED_EDGE('',*,*,#1506,.F.);
#1990=ORIENTED_EDGE('',*,*,#1511,.F.);
#1991=ORIENTED_EDGE('',*,*,#1512,.T.);
#1992=ORIENTED_EDGE('',*,*,#1513,.T.);
#1993=ORIENTED_EDGE('',*,*,#1509,.F.);
#1994=ORIENTED_EDGE('',*,*,#1514,.F.);
#1995=ORIENTED_EDGE('',*,*,#1515,.T.);
#1996=ORIENTED_EDGE('',*,*,#1516,.T.);
#1997=ORIENTED_EDGE('',*,*,#1512,.F.);
#1998=ORIENTED_EDGE('',*,*,#1517,.F.);
#1999=ORIENTED_EDGE('',*,*,#1518,.F.);
#2000=ORIENTED_EDGE('',*,*,#1519,.F.);
#2001=ORIENTED_EDGE('',*,*,#1520,.F.);
#2002=ORIENTED_EDGE('',*,*,#1521,.T.);
#2003=ORIENTED_EDGE('',*,*,#1522,.T.);
#2004=ORIENTED_EDGE('',*,*,#1523,.T.);
#2005=ORIENTED_EDGE('',*,*,#1524,.F.);
#2006=ORIENTED_EDGE('',*,*,#1525,.F.);
#2007=ORIENTED_EDGE('',*,*,#1526,.T.);
#2008=ORIENTED_EDGE('',*,*,#1527,.T.);
#2009=ORIENTED_EDGE('',*,*,#1522,.F.);
#2010=ORIENTED_EDGE('',*,*,#1528,.F.);
#2011=ORIENTED_EDGE('',*,*,#1529,.T.);
#2012=ORIENTED_EDGE('',*,*,#1530,.T.);
#2013=ORIENTED_EDGE('',*,*,#1526,.F.);
#2014=ORIENTED_EDGE('',*,*,#1531,.F.);
#2015=ORIENTED_EDGE('',*,*,#1532,.T.);
#2016=ORIENTED_EDGE('',*,*,#1533,.T.);
#2017=ORIENTED_EDGE('',*,*,#1529,.F.);
#2018=ORIENTED_EDGE('',*,*,#1534,.F.);
#2019=ORIENTED_EDGE('',*,*,#1535,.T.);
#2020=ORIENTED_EDGE('',*,*,#1536,.T.);
#2021=ORIENTED_EDGE('',*,*,#1532,.F.);
#2022=ORIENTED_EDGE('',*,*,#1537,.F.);
#2023=ORIENTED_EDGE('',*,*,#1538,.T.);
#2024=ORIENTED_EDGE('',*,*,#1539,.T.);
#2025=ORIENTED_EDGE('',*,*,#1535,.F.);
#2026=ORIENTED_EDGE('',*,*,#1540,.F.);
#2027=ORIENTED_EDGE('',*,*,#1541,.T.);
#2028=ORIENTED_EDGE('',*,*,#1542,.T.);
#2029=ORIENTED_EDGE('',*,*,#1538,.F.);
#2030=ORIENTED_EDGE('',*,*,#1543,.F.);
#2031=ORIENTED_EDGE('',*,*,#1544,.T.);
#2032=ORIENTED_EDGE('',*,*,#1545,.T.);
#2033=ORIENTED_EDGE('',*,*,#1541,.F.);
#2034=ORIENTED_EDGE('',*,*,#1546,.F.);
#2035=ORIENTED_EDGE('',*,*,#1547,.T.);
#2036=ORIENTED_EDGE('',*,*,#1548,.T.);
#2037=ORIENTED_EDGE('',*,*,#1544,.F.);
#2038=ORIENTED_EDGE('',*,*,#1549,.F.);
#2039=ORIENTED_EDGE('',*,*,#1550,.T.);
#2040=ORIENTED_EDGE('',*,*,#1551,.T.);
#2041=ORIENTED_EDGE('',*,*,#1547,.F.);
#2042=ORIENTED_EDGE('',*,*,#1552,.F.);
#2043=ORIENTED_EDGE('',*,*,#1553,.T.);
#2044=ORIENTED_EDGE('',*,*,#1554,.T.);
#2045=ORIENTED_EDGE('',*,*,#1550,.F.);
#2046=ORIENTED_EDGE('',*,*,#1555,.F.);
#2047=ORIENTED_EDGE('',*,*,#1556,.T.);
#2048=ORIENTED_EDGE('',*,*,#1557,.T.);
#2049=ORIENTED_EDGE('',*,*,#1553,.F.);
#2050=ORIENTED_EDGE('',*,*,#1558,.F.);
#2051=ORIENTED_EDGE('',*,*,#1559,.T.);
#2052=ORIENTED_EDGE('',*,*,#1560,.T.);
#2053=ORIENTED_EDGE('',*,*,#1556,.F.);
#2054=ORIENTED_EDGE('',*,*,#1561,.F.);
#2055=ORIENTED_EDGE('',*,*,#1562,.T.);
#2056=ORIENTED_EDGE('',*,*,#1563,.T.);
#2057=ORIENTED_EDGE('',*,*,#1559,.F.);
#2058=ORIENTED_EDGE('',*,*,#1564,.F.);
#2059=ORIENTED_EDGE('',*,*,#1565,.T.);
#2060=ORIENTED_EDGE('',*,*,#1566,.T.);
#2061=ORIENTED_EDGE('',*,*,#1562,.F.);
#2062=ORIENTED_EDGE('',*,*,#1567,.F.);
#2063=ORIENTED_EDGE('',*,*,#1568,.T.);
#2064=ORIENTED_EDGE('',*,*,#1569,.T.);
#2065=ORIENTED_EDGE('',*,*,#1565,.F.);
#2066=ORIENTED_EDGE('',*,*,#1570,.F.);
#2067=ORIENTED_EDGE('',*,*,#1571,.T.);
#2068=ORIENTED_EDGE('',*,*,#1572,.T.);
#2069=ORIENTED_EDGE('',*,*,#1568,.F.);
#2070=ORIENTED_EDGE('',*,*,#1573,.F.);
#2071=ORIENTED_EDGE('',*,*,#1574,.T.);
#2072=ORIENTED_EDGE('',*,*,#1575,.T.);
#2073=ORIENTED_EDGE('',*,*,#1571,.F.);
#2074=ORIENTED_EDGE('',*,*,#1576,.F.);
#2075=ORIENTED_EDGE('',*,*,#1577,.T.);
#2076=ORIENTED_EDGE('',*,*,#1578,.T.);
#2077=ORIENTED_EDGE('',*,*,#1574,.F.);
#2078=ORIENTED_EDGE('',*,*,#1579,.F.);
#2079=ORIENTED_EDGE('',*,*,#1580,.T.);
#2080=ORIENTED_EDGE('',*,*,#1581,.T.);
#2081=ORIENTED_EDGE('',*,*,#1577,.F.);
#2082=ORIENTED_EDGE('',*,*,#1582,.F.);
#2083=ORIENTED_EDGE('',*,*,#1583,.T.);
#2084=ORIENTED_EDGE('',*,*,#1584,.T.);
#2085=ORIENTED_EDGE('',*,*,#1580,.F.);
#2086=ORIENTED_EDGE('',*,*,#1585,.F.);
#2087=ORIENTED_EDGE('',*,*,#1586,.T.);
#2088=ORIENTED_EDGE('',*,*,#1587,.T.);
#2089=ORIENTED_EDGE('',*,*,#1583,.F.);
#2090=ORIENTED_EDGE('',*,*,#1588,.F.);
#2091=ORIENTED_EDGE('',*,*,#1589,.T.);
#2092=ORIENTED_EDGE('',*,*,#1590,.T.);
#2093=ORIENTED_EDGE('',*,*,#1586,.F.);
#2094=ORIENTED_EDGE('',*,*,#1591,.F.);
#2095=ORIENTED_EDGE('',*,*,#1592,.T.);
#2096=ORIENTED_EDGE('',*,*,#1593,.T.);
#2097=ORIENTED_EDGE('',*,*,#1589,.F.);
#2098=ORIENTED_EDGE('',*,*,#1594,.F.);
#2099=ORIENTED_EDGE('',*,*,#1595,.T.);
#2100=ORIENTED_EDGE('',*,*,#1596,.T.);
#2101=ORIENTED_EDGE('',*,*,#1592,.F.);
#2102=ORIENTED_EDGE('',*,*,#1597,.F.);
#2103=ORIENTED_EDGE('',*,*,#1598,.T.);
#2104=ORIENTED_EDGE('',*,*,#1599,.T.);
#2105=ORIENTED_EDGE('',*,*,#1595,.F.);
#2106=ORIENTED_EDGE('',*,*,#1600,.F.);
#2107=ORIENTED_EDGE('',*,*,#1601,.T.);
#2108=ORIENTED_EDGE('',*,*,#1602,.T.);
#2109=ORIENTED_EDGE('',*,*,#1598,.F.);
#2110=ORIENTED_EDGE('',*,*,#1603,.F.);
#2111=ORIENTED_EDGE('',*,*,#1604,.T.);
#2112=ORIENTED_EDGE('',*,*,#1605,.T.);
#2113=ORIENTED_EDGE('',*,*,#1601,.F.);
#2114=ORIENTED_EDGE('',*,*,#1606,.F.);
#2115=ORIENTED_EDGE('',*,*,#1607,.T.);
#2116=ORIENTED_EDGE('',*,*,#1608,.T.);
#2117=ORIENTED_EDGE('',*,*,#1604,.F.);
#2118=ORIENTED_EDGE('',*,*,#1609,.F.);
#2119=ORIENTED_EDGE('',*,*,#1610,.T.);
#2120=ORIENTED_EDGE('',*,*,#1611,.T.);
#2121=ORIENTED_EDGE('',*,*,#1607,.F.);
#2122=ORIENTED_EDGE('',*,*,#1612,.F.);
#2123=ORIENTED_EDGE('',*,*,#1613,.T.);
#2124=ORIENTED_EDGE('',*,*,#1614,.T.);
#2125=ORIENTED_EDGE('',*,*,#1610,.F.);
#2126=ORIENTED_EDGE('',*,*,#1615,.F.);
#2127=ORIENTED_EDGE('',*,*,#1616,.T.);
#2128=ORIENTED_EDGE('',*,*,#1617,.T.);
#2129=ORIENTED_EDGE('',*,*,#1613,.F.);
#2130=ORIENTED_EDGE('',*,*,#1618,.F.);
#2131=ORIENTED_EDGE('',*,*,#1619,.T.);
#2132=ORIENTED_EDGE('',*,*,#1620,.T.);
#2133=ORIENTED_EDGE('',*,*,#1616,.F.);
#2134=ORIENTED_EDGE('',*,*,#1621,.F.);
#2135=ORIENTED_EDGE('',*,*,#1622,.T.);
#2136=ORIENTED_EDGE('',*,*,#1623,.T.);
#2137=ORIENTED_EDGE('',*,*,#1619,.F.);
#2138=ORIENTED_EDGE('',*,*,#1624,.F.);
#2139=ORIENTED_EDGE('',*,*,#1625,.T.);
#2140=ORIENTED_EDGE('',*,*,#1626,.T.);
#2141=ORIENTED_EDGE('',*,*,#1622,.F.);
#2142=ORIENTED_EDGE('',*,*,#1627,.F.);
#2143=ORIENTED_EDGE('',*,*,#1628,.T.);
#2144=ORIENTED_EDGE('',*,*,#1629,.T.);
#2145=ORIENTED_EDGE('',*,*,#1625,.F.);
#2146=ORIENTED_EDGE('',*,*,#1630,.F.);
#2147=ORIENTED_EDGE('',*,*,#1631,.T.);
#2148=ORIENTED_EDGE('',*,*,#1632,.T.);
#2149=ORIENTED_EDGE('',*,*,#1628,.F.);
#2150=ORIENTED_EDGE('',*,*,#1633,.F.);
#2151=ORIENTED_EDGE('',*,*,#1634,.T.);
#2152=ORIENTED_EDGE('',*,*,#1635,.T.);
#2153=ORIENTED_EDGE('',*,*,#1631,.F.);
#2154=ORIENTED_EDGE('',*,*,#1636,.F.);
#2155=ORIENTED_EDGE('',*,*,#1637,.T.);
#2156=ORIENTED_EDGE('',*,*,#1638,.T.);
#2157=ORIENTED_EDGE('',*,*,#1634,.F.);
#2158=ORIENTED_EDGE('',*,*,#1639,.F.);
#2159=ORIENTED_EDGE('',*,*,#1640,.T.);
#2160=ORIENTED_EDGE('',*,*,#1641,.T.);
#2161=ORIENTED_EDGE('',*,*,#1637,.F.);
#2162=ORIENTED_EDGE('',*,*,#1642,.F.);
#2163=ORIENTED_EDGE('',*,*,#1643,.T.);
#2164=ORIENTED_EDGE('',*,*,#1644,.T.);
#2165=ORIENTED_EDGE('',*,*,#1640,.F.);
#2166=ORIENTED_EDGE('',*,*,#1645,.F.);
#2167=ORIENTED_EDGE('',*,*,#1646,.T.);
#2168=ORIENTED_EDGE('',*,*,#1647,.T.);
#2169=ORIENTED_EDGE('',*,*,#1643,.F.);
#2170=ORIENTED_EDGE('',*,*,#1648,.F.);
#2171=ORIENTED_EDGE('',*,*,#1649,.T.);
#2172=ORIENTED_EDGE('',*,*,#1650,.T.);
#2173=ORIENTED_EDGE('',*,*,#1646,.F.);
#2174=ORIENTED_EDGE('',*,*,#1651,.F.);
#2175=ORIENTED_EDGE('',*,*,#1652,.T.);
#2176=ORIENTED_EDGE('',*,*,#1653,.T.);
#2177=ORIENTED_EDGE('',*,*,#1649,.F.);
#2178=ORIENTED_EDGE('',*,*,#1654,.F.);
#2179=ORIENTED_EDGE('',*,*,#1655,.T.);
#2180=ORIENTED_EDGE('',*,*,#1656,.T.);
#2181=ORIENTED_EDGE('',*,*,#1652,.F.);
#2182=ORIENTED_EDGE('',*,*,#1657,.F.);
#2183=ORIENTED_EDGE('',*,*,#1658,.T.);
#2184=ORIENTED_EDGE('',*,*,#1659,.T.);
#2185=ORIENTED_EDGE('',*,*,#1655,.F.);
#2186=ORIENTED_EDGE('',*,*,#1660,.F.);
#2187=ORIENTED_EDGE('',*,*,#1661,.T.);
#2188=ORIENTED_EDGE('',*,*,#1662,.T.);
#2189=ORIENTED_EDGE('',*,*,#1658,.F.);
#2190=ORIENTED_EDGE('',*,*,#1663,.F.);
#2191=ORIENTED_EDGE('',*,*,#1664,.T.);
#2192=ORIENTED_EDGE('',*,*,#1665,.T.);
#2193=ORIENTED_EDGE('',*,*,#1661,.F.);
#2194=ORIENTED_EDGE('',*,*,#1666,.F.);
#2195=ORIENTED_EDGE('',*,*,#1667,.T.);
#2196=ORIENTED_EDGE('',*,*,#1668,.T.);
#2197=ORIENTED_EDGE('',*,*,#1669,.T.);
#2198=ORIENTED_EDGE('',*,*,#1670,.F.);
#2199=ORIENTED_EDGE('',*,*,#1671,.F.);
#2200=ORIENTED_EDGE('',*,*,#1672,.F.);
#2201=ORIENTED_EDGE('',*,*,#1673,.T.);
#2202=ORIENTED_EDGE('',*,*,#1668,.F.);
#2203=ORIENTED_EDGE('',*,*,#1674,.T.);
#2204=ORIENTED_EDGE('',*,*,#1675,.T.);
#2205=ORIENTED_EDGE('',*,*,#1676,.T.);
#2206=ORIENTED_EDGE('',*,*,#1677,.T.);
#2207=ORIENTED_EDGE('',*,*,#1676,.F.);
#2208=ORIENTED_EDGE('',*,*,#1678,.F.);
#2209=ORIENTED_EDGE('',*,*,#1679,.F.);
#2210=ORIENTED_EDGE('',*,*,#1680,.F.);
#2211=ORIENTED_EDGE('',*,*,#1681,.F.);
#2212=ORIENTED_EDGE('',*,*,#1670,.T.);
#2213=ORIENTED_EDGE('',*,*,#1682,.T.);
#2214=ORIENTED_EDGE('',*,*,#1664,.F.);
#2215=ORIENTED_EDGE('',*,*,#1683,.F.);
#2216=ORIENTED_EDGE('',*,*,#1684,.T.);
#2217=ORIENTED_EDGE('',*,*,#1685,.F.);
#2218=ORIENTED_EDGE('',*,*,#1686,.T.);
#2219=ORIENTED_EDGE('',*,*,#1524,.T.);
#2220=ORIENTED_EDGE('',*,*,#1687,.T.);
#2221=ORIENTED_EDGE('',*,*,#1688,.T.);
#2222=ORIENTED_EDGE('',*,*,#1667,.F.);
#2223=ORIENTED_EDGE('',*,*,#1677,.F.);
#2224=ORIENTED_EDGE('',*,*,#1689,.T.);
#2225=ORIENTED_EDGE('',*,*,#1684,.F.);
#2226=ORIENTED_EDGE('',*,*,#1689,.F.);
#2227=ORIENTED_EDGE('',*,*,#1690,.T.);
#2228=ORIENTED_EDGE('',*,*,#1672,.T.);
#2229=ORIENTED_EDGE('',*,*,#1691,.T.);
#2230=ORIENTED_EDGE('',*,*,#1520,.T.);
#2231=ORIENTED_EDGE('',*,*,#1692,.T.);
#2232=ORIENTED_EDGE('',*,*,#1372,.T.);
#2233=ORIENTED_EDGE('',*,*,#1693,.T.);
#2234=ORIENTED_EDGE('',*,*,#1694,.T.);
#2235=ORIENTED_EDGE('',*,*,#1690,.F.);
#2236=ORIENTED_EDGE('',*,*,#1519,.T.);
#2237=ORIENTED_EDGE('',*,*,#1695,.T.);
#2238=ORIENTED_EDGE('',*,*,#1517,.T.);
#2239=ORIENTED_EDGE('',*,*,#1514,.T.);
#2240=ORIENTED_EDGE('',*,*,#1511,.T.);
#2241=ORIENTED_EDGE('',*,*,#1508,.T.);
#2242=ORIENTED_EDGE('',*,*,#1505,.T.);
#2243=ORIENTED_EDGE('',*,*,#1502,.T.);
#2244=ORIENTED_EDGE('',*,*,#1499,.T.);
#2245=ORIENTED_EDGE('',*,*,#1496,.T.);
#2246=ORIENTED_EDGE('',*,*,#1493,.T.);
#2247=ORIENTED_EDGE('',*,*,#1490,.T.);
#2248=ORIENTED_EDGE('',*,*,#1487,.T.);
#2249=ORIENTED_EDGE('',*,*,#1484,.T.);
#2250=ORIENTED_EDGE('',*,*,#1481,.T.);
#2251=ORIENTED_EDGE('',*,*,#1478,.T.);
#2252=ORIENTED_EDGE('',*,*,#1475,.T.);
#2253=ORIENTED_EDGE('',*,*,#1472,.T.);
#2254=ORIENTED_EDGE('',*,*,#1469,.T.);
#2255=ORIENTED_EDGE('',*,*,#1466,.T.);
#2256=ORIENTED_EDGE('',*,*,#1463,.T.);
#2257=ORIENTED_EDGE('',*,*,#1460,.T.);
#2258=ORIENTED_EDGE('',*,*,#1457,.T.);
#2259=ORIENTED_EDGE('',*,*,#1454,.T.);
#2260=ORIENTED_EDGE('',*,*,#1451,.T.);
#2261=ORIENTED_EDGE('',*,*,#1448,.T.);
#2262=ORIENTED_EDGE('',*,*,#1445,.T.);
#2263=ORIENTED_EDGE('',*,*,#1442,.T.);
#2264=ORIENTED_EDGE('',*,*,#1439,.T.);
#2265=ORIENTED_EDGE('',*,*,#1436,.T.);
#2266=ORIENTED_EDGE('',*,*,#1433,.T.);
#2267=ORIENTED_EDGE('',*,*,#1430,.T.);
#2268=ORIENTED_EDGE('',*,*,#1427,.T.);
#2269=ORIENTED_EDGE('',*,*,#1424,.T.);
#2270=ORIENTED_EDGE('',*,*,#1421,.T.);
#2271=ORIENTED_EDGE('',*,*,#1418,.T.);
#2272=ORIENTED_EDGE('',*,*,#1415,.T.);
#2273=ORIENTED_EDGE('',*,*,#1412,.T.);
#2274=ORIENTED_EDGE('',*,*,#1409,.T.);
#2275=ORIENTED_EDGE('',*,*,#1406,.T.);
#2276=ORIENTED_EDGE('',*,*,#1403,.T.);
#2277=ORIENTED_EDGE('',*,*,#1400,.T.);
#2278=ORIENTED_EDGE('',*,*,#1397,.T.);
#2279=ORIENTED_EDGE('',*,*,#1394,.T.);
#2280=ORIENTED_EDGE('',*,*,#1391,.T.);
#2281=ORIENTED_EDGE('',*,*,#1388,.T.);
#2282=ORIENTED_EDGE('',*,*,#1385,.T.);
#2283=ORIENTED_EDGE('',*,*,#1382,.T.);
#2284=ORIENTED_EDGE('',*,*,#1379,.T.);
#2285=ORIENTED_EDGE('',*,*,#1376,.T.);
#2286=ORIENTED_EDGE('',*,*,#1373,.T.);
#2287=ORIENTED_EDGE('',*,*,#1692,.F.);
#2288=ORIENTED_EDGE('',*,*,#1523,.F.);
#2289=ORIENTED_EDGE('',*,*,#1527,.F.);
#2290=ORIENTED_EDGE('',*,*,#1530,.F.);
#2291=ORIENTED_EDGE('',*,*,#1533,.F.);
#2292=ORIENTED_EDGE('',*,*,#1536,.F.);
#2293=ORIENTED_EDGE('',*,*,#1539,.F.);
#2294=ORIENTED_EDGE('',*,*,#1542,.F.);
#2295=ORIENTED_EDGE('',*,*,#1545,.F.);
#2296=ORIENTED_EDGE('',*,*,#1548,.F.);
#2297=ORIENTED_EDGE('',*,*,#1551,.F.);
#2298=ORIENTED_EDGE('',*,*,#1554,.F.);
#2299=ORIENTED_EDGE('',*,*,#1557,.F.);
#2300=ORIENTED_EDGE('',*,*,#1560,.F.);
#2301=ORIENTED_EDGE('',*,*,#1563,.F.);
#2302=ORIENTED_EDGE('',*,*,#1566,.F.);
#2303=ORIENTED_EDGE('',*,*,#1569,.F.);
#2304=ORIENTED_EDGE('',*,*,#1572,.F.);
#2305=ORIENTED_EDGE('',*,*,#1575,.F.);
#2306=ORIENTED_EDGE('',*,*,#1578,.F.);
#2307=ORIENTED_EDGE('',*,*,#1581,.F.);
#2308=ORIENTED_EDGE('',*,*,#1584,.F.);
#2309=ORIENTED_EDGE('',*,*,#1587,.F.);
#2310=ORIENTED_EDGE('',*,*,#1590,.F.);
#2311=ORIENTED_EDGE('',*,*,#1593,.F.);
#2312=ORIENTED_EDGE('',*,*,#1596,.F.);
#2313=ORIENTED_EDGE('',*,*,#1599,.F.);
#2314=ORIENTED_EDGE('',*,*,#1602,.F.);
#2315=ORIENTED_EDGE('',*,*,#1605,.F.);
#2316=ORIENTED_EDGE('',*,*,#1608,.F.);
#2317=ORIENTED_EDGE('',*,*,#1611,.F.);
#2318=ORIENTED_EDGE('',*,*,#1614,.F.);
#2319=ORIENTED_EDGE('',*,*,#1617,.F.);
#2320=ORIENTED_EDGE('',*,*,#1620,.F.);
#2321=ORIENTED_EDGE('',*,*,#1623,.F.);
#2322=ORIENTED_EDGE('',*,*,#1626,.F.);
#2323=ORIENTED_EDGE('',*,*,#1629,.F.);
#2324=ORIENTED_EDGE('',*,*,#1632,.F.);
#2325=ORIENTED_EDGE('',*,*,#1635,.F.);
#2326=ORIENTED_EDGE('',*,*,#1638,.F.);
#2327=ORIENTED_EDGE('',*,*,#1641,.F.);
#2328=ORIENTED_EDGE('',*,*,#1644,.F.);
#2329=ORIENTED_EDGE('',*,*,#1647,.F.);
#2330=ORIENTED_EDGE('',*,*,#1650,.F.);
#2331=ORIENTED_EDGE('',*,*,#1653,.F.);
#2332=ORIENTED_EDGE('',*,*,#1656,.F.);
#2333=ORIENTED_EDGE('',*,*,#1659,.F.);
#2334=ORIENTED_EDGE('',*,*,#1662,.F.);
#2335=ORIENTED_EDGE('',*,*,#1665,.F.);
#2336=ORIENTED_EDGE('',*,*,#1682,.F.);
#2337=ORIENTED_EDGE('',*,*,#1669,.F.);
#2338=ORIENTED_EDGE('',*,*,#1673,.F.);
#2339=ORIENTED_EDGE('',*,*,#1518,.T.);
#2340=ORIENTED_EDGE('',*,*,#1696,.T.);
#2341=ORIENTED_EDGE('',*,*,#1515,.F.);
#2342=ORIENTED_EDGE('',*,*,#1695,.F.);
#2343=ORIENTED_EDGE('',*,*,#1691,.F.);
#2344=ORIENTED_EDGE('',*,*,#1671,.T.);
#2345=ORIENTED_EDGE('',*,*,#1683,.T.);
#2346=ORIENTED_EDGE('',*,*,#1666,.T.);
#2347=ORIENTED_EDGE('',*,*,#1663,.T.);
#2348=ORIENTED_EDGE('',*,*,#1660,.T.);
#2349=ORIENTED_EDGE('',*,*,#1657,.T.);
#2350=ORIENTED_EDGE('',*,*,#1654,.T.);
#2351=ORIENTED_EDGE('',*,*,#1651,.T.);
#2352=ORIENTED_EDGE('',*,*,#1648,.T.);
#2353=ORIENTED_EDGE('',*,*,#1645,.T.);
#2354=ORIENTED_EDGE('',*,*,#1642,.T.);
#2355=ORIENTED_EDGE('',*,*,#1639,.T.);
#2356=ORIENTED_EDGE('',*,*,#1636,.T.);
#2357=ORIENTED_EDGE('',*,*,#1633,.T.);
#2358=ORIENTED_EDGE('',*,*,#1630,.T.);
#2359=ORIENTED_EDGE('',*,*,#1627,.T.);
#2360=ORIENTED_EDGE('',*,*,#1624,.T.);
#2361=ORIENTED_EDGE('',*,*,#1621,.T.);
#2362=ORIENTED_EDGE('',*,*,#1618,.T.);
#2363=ORIENTED_EDGE('',*,*,#1615,.T.);
#2364=ORIENTED_EDGE('',*,*,#1612,.T.);
#2365=ORIENTED_EDGE('',*,*,#1609,.T.);
#2366=ORIENTED_EDGE('',*,*,#1606,.T.);
#2367=ORIENTED_EDGE('',*,*,#1603,.T.);
#2368=ORIENTED_EDGE('',*,*,#1600,.T.);
#2369=ORIENTED_EDGE('',*,*,#1597,.T.);
#2370=ORIENTED_EDGE('',*,*,#1594,.T.);
#2371=ORIENTED_EDGE('',*,*,#1591,.T.);
#2372=ORIENTED_EDGE('',*,*,#1588,.T.);
#2373=ORIENTED_EDGE('',*,*,#1585,.T.);
#2374=ORIENTED_EDGE('',*,*,#1582,.T.);
#2375=ORIENTED_EDGE('',*,*,#1579,.T.);
#2376=ORIENTED_EDGE('',*,*,#1576,.T.);
#2377=ORIENTED_EDGE('',*,*,#1573,.T.);
#2378=ORIENTED_EDGE('',*,*,#1570,.T.);
#2379=ORIENTED_EDGE('',*,*,#1567,.T.);
#2380=ORIENTED_EDGE('',*,*,#1564,.T.);
#2381=ORIENTED_EDGE('',*,*,#1561,.T.);
#2382=ORIENTED_EDGE('',*,*,#1558,.T.);
#2383=ORIENTED_EDGE('',*,*,#1555,.T.);
#2384=ORIENTED_EDGE('',*,*,#1552,.T.);
#2385=ORIENTED_EDGE('',*,*,#1549,.T.);
#2386=ORIENTED_EDGE('',*,*,#1546,.T.);
#2387=ORIENTED_EDGE('',*,*,#1543,.T.);
#2388=ORIENTED_EDGE('',*,*,#1540,.T.);
#2389=ORIENTED_EDGE('',*,*,#1537,.T.);
#2390=ORIENTED_EDGE('',*,*,#1534,.T.);
#2391=ORIENTED_EDGE('',*,*,#1531,.T.);
#2392=ORIENTED_EDGE('',*,*,#1528,.T.);
#2393=ORIENTED_EDGE('',*,*,#1525,.T.);
#2394=ORIENTED_EDGE('',*,*,#1697,.T.);
#2395=ORIENTED_EDGE('',*,*,#1693,.F.);
#2396=ORIENTED_EDGE('',*,*,#1371,.F.);
#2397=ORIENTED_EDGE('',*,*,#1375,.F.);
#2398=ORIENTED_EDGE('',*,*,#1378,.F.);
#2399=ORIENTED_EDGE('',*,*,#1381,.F.);
#2400=ORIENTED_EDGE('',*,*,#1384,.F.);
#2401=ORIENTED_EDGE('',*,*,#1387,.F.);
#2402=ORIENTED_EDGE('',*,*,#1390,.F.);
#2403=ORIENTED_EDGE('',*,*,#1393,.F.);
#2404=ORIENTED_EDGE('',*,*,#1396,.F.);
#2405=ORIENTED_EDGE('',*,*,#1399,.F.);
#2406=ORIENTED_EDGE('',*,*,#1402,.F.);
#2407=ORIENTED_EDGE('',*,*,#1405,.F.);
#2408=ORIENTED_EDGE('',*,*,#1408,.F.);
#2409=ORIENTED_EDGE('',*,*,#1411,.F.);
#2410=ORIENTED_EDGE('',*,*,#1414,.F.);
#2411=ORIENTED_EDGE('',*,*,#1417,.F.);
#2412=ORIENTED_EDGE('',*,*,#1420,.F.);
#2413=ORIENTED_EDGE('',*,*,#1423,.F.);
#2414=ORIENTED_EDGE('',*,*,#1426,.F.);
#2415=ORIENTED_EDGE('',*,*,#1429,.F.);
#2416=ORIENTED_EDGE('',*,*,#1432,.F.);
#2417=ORIENTED_EDGE('',*,*,#1435,.F.);
#2418=ORIENTED_EDGE('',*,*,#1438,.F.);
#2419=ORIENTED_EDGE('',*,*,#1441,.F.);
#2420=ORIENTED_EDGE('',*,*,#1444,.F.);
#2421=ORIENTED_EDGE('',*,*,#1447,.F.);
#2422=ORIENTED_EDGE('',*,*,#1450,.F.);
#2423=ORIENTED_EDGE('',*,*,#1453,.F.);
#2424=ORIENTED_EDGE('',*,*,#1456,.F.);
#2425=ORIENTED_EDGE('',*,*,#1459,.F.);
#2426=ORIENTED_EDGE('',*,*,#1462,.F.);
#2427=ORIENTED_EDGE('',*,*,#1465,.F.);
#2428=ORIENTED_EDGE('',*,*,#1468,.F.);
#2429=ORIENTED_EDGE('',*,*,#1471,.F.);
#2430=ORIENTED_EDGE('',*,*,#1474,.F.);
#2431=ORIENTED_EDGE('',*,*,#1477,.F.);
#2432=ORIENTED_EDGE('',*,*,#1480,.F.);
#2433=ORIENTED_EDGE('',*,*,#1483,.F.);
#2434=ORIENTED_EDGE('',*,*,#1486,.F.);
#2435=ORIENTED_EDGE('',*,*,#1489,.F.);
#2436=ORIENTED_EDGE('',*,*,#1492,.F.);
#2437=ORIENTED_EDGE('',*,*,#1495,.F.);
#2438=ORIENTED_EDGE('',*,*,#1498,.F.);
#2439=ORIENTED_EDGE('',*,*,#1501,.F.);
#2440=ORIENTED_EDGE('',*,*,#1504,.F.);
#2441=ORIENTED_EDGE('',*,*,#1507,.F.);
#2442=ORIENTED_EDGE('',*,*,#1510,.F.);
#2443=ORIENTED_EDGE('',*,*,#1513,.F.);
#2444=ORIENTED_EDGE('',*,*,#1516,.F.);
#2445=ORIENTED_EDGE('',*,*,#1696,.F.);
#2446=ORIENTED_EDGE('',*,*,#1521,.F.);
#2447=ORIENTED_EDGE('',*,*,#1687,.F.);
#2448=ORIENTED_EDGE('',*,*,#1694,.F.);
#2449=ORIENTED_EDGE('',*,*,#1697,.F.);
#2450=ORIENTED_EDGE('',*,*,#1678,.T.);
#2451=ORIENTED_EDGE('',*,*,#1698,.T.);
#2452=ORIENTED_EDGE('',*,*,#1699,.T.);
#2453=ORIENTED_EDGE('',*,*,#1698,.F.);
#2454=ORIENTED_EDGE('',*,*,#1679,.T.);
#2455=ORIENTED_EDGE('',*,*,#1699,.F.);
#2456=ORIENTED_EDGE('',*,*,#1680,.T.);
#2457=ORIENTED_EDGE('',*,*,#1700,.T.);
#2458=ORIENTED_EDGE('',*,*,#1701,.F.);
#2459=ORIENTED_EDGE('',*,*,#1700,.F.);
#2460=ORIENTED_EDGE('',*,*,#1681,.T.);
#2461=ORIENTED_EDGE('',*,*,#1701,.T.);
#2462=ORIENTED_EDGE('',*,*,#1688,.F.);
#2463=ORIENTED_EDGE('',*,*,#1702,.T.);
#2464=ORIENTED_EDGE('',*,*,#1685,.T.);
#2465=ORIENTED_EDGE('',*,*,#1702,.F.);
#2466=ORIENTED_EDGE('',*,*,#1674,.F.);
#2467=ORIENTED_EDGE('',*,*,#1675,.F.);
#2468=ORIENTED_EDGE('',*,*,#1703,.T.);
#2469=ORIENTED_EDGE('',*,*,#1686,.F.);
#2470=ORIENTED_EDGE('',*,*,#1703,.F.);
#2669=CYLINDRICAL_SURFACE('',#3040,104.958734125);
#2670=CYLINDRICAL_SURFACE('',#3041,104.958734125);
#2671=CYLINDRICAL_SURFACE('',#3042,104.958734125);
#2672=CYLINDRICAL_SURFACE('',#3043,104.958734125);
#2673=CYLINDRICAL_SURFACE('',#3044,104.958734125);
#2674=CYLINDRICAL_SURFACE('',#3045,104.958734125);
#2675=CYLINDRICAL_SURFACE('',#3046,104.958734125);
#2676=CYLINDRICAL_SURFACE('',#3047,104.958734125);
#2677=CYLINDRICAL_SURFACE('',#3048,104.958734125);
#2678=CYLINDRICAL_SURFACE('',#3049,104.958734125);
#2679=CYLINDRICAL_SURFACE('',#3050,104.958734125);
#2680=CYLINDRICAL_SURFACE('',#3051,104.958734125);
#2681=CYLINDRICAL_SURFACE('',#3052,104.958734125);
#2682=CYLINDRICAL_SURFACE('',#3053,104.958734125);
#2683=CYLINDRICAL_SURFACE('',#3054,104.958734125);
#2684=CYLINDRICAL_SURFACE('',#3055,104.958734125);
#2685=CYLINDRICAL_SURFACE('',#3056,104.958734125);
#2686=CYLINDRICAL_SURFACE('',#3057,104.958734125);
#2687=CYLINDRICAL_SURFACE('',#3058,104.958734125);
#2688=CYLINDRICAL_SURFACE('',#3059,104.958734125);
#2689=CYLINDRICAL_SURFACE('',#3060,104.958734125);
#2690=CYLINDRICAL_SURFACE('',#3061,104.958734125);
#2691=CYLINDRICAL_SURFACE('',#3062,104.958734125);
#2692=CYLINDRICAL_SURFACE('',#3063,104.958734125);
#2693=CYLINDRICAL_SURFACE('',#3064,104.958734125);
#2694=CYLINDRICAL_SURFACE('',#3065,104.958734125);
#2695=CYLINDRICAL_SURFACE('',#3066,104.958734125);
#2696=CYLINDRICAL_SURFACE('',#3067,104.958734125);
#2697=CYLINDRICAL_SURFACE('',#3068,104.958734125);
#2698=CYLINDRICAL_SURFACE('',#3069,104.958734125);
#2699=CYLINDRICAL_SURFACE('',#3070,104.958734125);
#2700=CYLINDRICAL_SURFACE('',#3071,104.958734125);
#2701=CYLINDRICAL_SURFACE('',#3072,104.958734125);
#2702=CYLINDRICAL_SURFACE('',#3073,104.958734125);
#2703=CYLINDRICAL_SURFACE('',#3074,104.958734125);
#2704=CYLINDRICAL_SURFACE('',#3075,104.958734125);
#2705=CYLINDRICAL_SURFACE('',#3076,104.958734125);
#2706=CYLINDRICAL_SURFACE('',#3077,104.958734125);
#2707=CYLINDRICAL_SURFACE('',#3078,104.958734125);
#2708=CYLINDRICAL_SURFACE('',#3079,104.958734125);
#2709=CYLINDRICAL_SURFACE('',#3080,104.958734125);
#2710=CYLINDRICAL_SURFACE('',#3081,104.958734125);
#2711=CYLINDRICAL_SURFACE('',#3082,104.958734125);
#2712=CYLINDRICAL_SURFACE('',#3083,104.958734125);
#2713=CYLINDRICAL_SURFACE('',#3084,104.958734125);
#2714=CYLINDRICAL_SURFACE('',#3085,104.958734125);
#2715=CYLINDRICAL_SURFACE('',#3086,104.958734125);
#2716=CYLINDRICAL_SURFACE('',#3087,104.958734125);
#2717=CYLINDRICAL_SURFACE('',#3088,104.958734125);
#2718=CYLINDRICAL_SURFACE('',#3089,104.958734125);
#2719=CYLINDRICAL_SURFACE('',#3090,105.5);
#2720=CYLINDRICAL_SURFACE('',#3092,105.5);
#2721=CYLINDRICAL_SURFACE('',#3093,105.5);
#2722=CYLINDRICAL_SURFACE('',#3094,105.5);
#2723=CYLINDRICAL_SURFACE('',#3095,105.5);
#2724=CYLINDRICAL_SURFACE('',#3096,105.5);
#2725=CYLINDRICAL_SURFACE('',#3097,105.5);
#2726=CYLINDRICAL_SURFACE('',#3098,105.5);
#2727=CYLINDRICAL_SURFACE('',#3099,105.5);
#2728=CYLINDRICAL_SURFACE('',#3100,105.5);
#2729=CYLINDRICAL_SURFACE('',#3101,105.5);
#2730=CYLINDRICAL_SURFACE('',#3102,105.5);
#2731=CYLINDRICAL_SURFACE('',#3103,105.5);
#2732=CYLINDRICAL_SURFACE('',#3104,105.5);
#2733=CYLINDRICAL_SURFACE('',#3105,105.5);
#2734=CYLINDRICAL_SURFACE('',#3106,105.5);
#2735=CYLINDRICAL_SURFACE('',#3107,105.5);
#2736=CYLINDRICAL_SURFACE('',#3108,105.5);
#2737=CYLINDRICAL_SURFACE('',#3109,105.5);
#2738=CYLINDRICAL_SURFACE('',#3110,105.5);
#2739=CYLINDRICAL_SURFACE('',#3111,105.5);
#2740=CYLINDRICAL_SURFACE('',#3112,105.5);
#2741=CYLINDRICAL_SURFACE('',#3113,105.5);
#2742=CYLINDRICAL_SURFACE('',#3114,105.5);
#2743=CYLINDRICAL_SURFACE('',#3115,105.5);
#2744=CYLINDRICAL_SURFACE('',#3116,105.5);
#2745=CYLINDRICAL_SURFACE('',#3117,105.5);
#2746=CYLINDRICAL_SURFACE('',#3118,105.5);
#2747=CYLINDRICAL_SURFACE('',#3119,105.5);
#2748=CYLINDRICAL_SURFACE('',#3120,105.5);
#2749=CYLINDRICAL_SURFACE('',#3121,105.5);
#2750=CYLINDRICAL_SURFACE('',#3122,105.5);
#2751=CYLINDRICAL_SURFACE('',#3123,105.5);
#2752=CYLINDRICAL_SURFACE('',#3124,105.5);
#2753=CYLINDRICAL_SURFACE('',#3125,105.5);
#2754=CYLINDRICAL_SURFACE('',#3126,105.5);
#2755=CYLINDRICAL_SURFACE('',#3127,105.5);
#2756=CYLINDRICAL_SURFACE('',#3128,105.5);
#2757=CYLINDRICAL_SURFACE('',#3129,105.5);
#2758=CYLINDRICAL_SURFACE('',#3130,105.5);
#2759=CYLINDRICAL_SURFACE('',#3131,105.5);
#2760=CYLINDRICAL_SURFACE('',#3132,105.5);
#2761=CYLINDRICAL_SURFACE('',#3133,105.5);
#2762=CYLINDRICAL_SURFACE('',#3134,105.5);
#2763=CYLINDRICAL_SURFACE('',#3135,105.5);
#2764=CYLINDRICAL_SURFACE('',#3136,105.5);
#2765=CYLINDRICAL_SURFACE('',#3137,105.5);
#2766=CYLINDRICAL_SURFACE('',#3138,105.5);
#2767=CYLINDRICAL_SURFACE('',#3139,105.5);
#2768=CYLINDRICAL_SURFACE('',#3141,120.5);
#2769=CYLINDRICAL_SURFACE('',#3145,105.5);
#2770=CYLINDRICAL_SURFACE('',#3157,104.958734125);
#2771=CYLINDRICAL_SURFACE('',#3158,105.5);
#2772=CYLINDRICAL_SURFACE('',#3159,9.99999999999999);
#2773=CYLINDRICAL_SURFACE('',#3162,9.99999999999999);
#2794=ADVANCED_FACE('',(#207),#2669,.F.);
#2795=ADVANCED_FACE('',(#208),#2670,.F.);
#2796=ADVANCED_FACE('',(#209),#2671,.F.);
#2797=ADVANCED_FACE('',(#210),#2672,.F.);
#2798=ADVANCED_FACE('',(#211),#2673,.F.);
#2799=ADVANCED_FACE('',(#212),#2674,.F.);
#2800=ADVANCED_FACE('',(#213),#2675,.F.);
#2801=ADVANCED_FACE('',(#214),#2676,.F.);
#2802=ADVANCED_FACE('',(#215),#2677,.F.);
#2803=ADVANCED_FACE('',(#216),#2678,.F.);
#2804=ADVANCED_FACE('',(#217),#2679,.F.);
#2805=ADVANCED_FACE('',(#218),#2680,.F.);
#2806=ADVANCED_FACE('',(#219),#2681,.F.);
#2807=ADVANCED_FACE('',(#220),#2682,.F.);
#2808=ADVANCED_FACE('',(#221),#2683,.F.);
#2809=ADVANCED_FACE('',(#222),#2684,.F.);
#2810=ADVANCED_FACE('',(#223),#2685,.F.);
#2811=ADVANCED_FACE('',(#224),#2686,.F.);
#2812=ADVANCED_FACE('',(#225),#2687,.F.);
#2813=ADVANCED_FACE('',(#226),#2688,.F.);
#2814=ADVANCED_FACE('',(#227),#2689,.F.);
#2815=ADVANCED_FACE('',(#228),#2690,.F.);
#2816=ADVANCED_FACE('',(#229),#2691,.F.);
#2817=ADVANCED_FACE('',(#230),#2692,.F.);
#2818=ADVANCED_FACE('',(#231),#2693,.F.);
#2819=ADVANCED_FACE('',(#232),#2694,.F.);
#2820=ADVANCED_FACE('',(#233),#2695,.F.);
#2821=ADVANCED_FACE('',(#234),#2696,.F.);
#2822=ADVANCED_FACE('',(#235),#2697,.F.);
#2823=ADVANCED_FACE('',(#236),#2698,.F.);
#2824=ADVANCED_FACE('',(#237),#2699,.F.);
#2825=ADVANCED_FACE('',(#238),#2700,.F.);
#2826=ADVANCED_FACE('',(#239),#2701,.F.);
#2827=ADVANCED_FACE('',(#240),#2702,.F.);
#2828=ADVANCED_FACE('',(#241),#2703,.F.);
#2829=ADVANCED_FACE('',(#242),#2704,.F.);
#2830=ADVANCED_FACE('',(#243),#2705,.F.);
#2831=ADVANCED_FACE('',(#244),#2706,.F.);
#2832=ADVANCED_FACE('',(#245),#2707,.F.);
#2833=ADVANCED_FACE('',(#246),#2708,.F.);
#2834=ADVANCED_FACE('',(#247),#2709,.F.);
#2835=ADVANCED_FACE('',(#248),#2710,.F.);
#2836=ADVANCED_FACE('',(#249),#2711,.F.);
#2837=ADVANCED_FACE('',(#250),#2712,.F.);
#2838=ADVANCED_FACE('',(#251),#2713,.F.);
#2839=ADVANCED_FACE('',(#252),#2714,.F.);
#2840=ADVANCED_FACE('',(#253),#2715,.F.);
#2841=ADVANCED_FACE('',(#254),#2716,.F.);
#2842=ADVANCED_FACE('',(#255),#2717,.F.);
#2843=ADVANCED_FACE('',(#256),#2718,.F.);
#2844=ADVANCED_FACE('',(#257),#2719,.F.);
#2845=ADVANCED_FACE('',(#258),#2720,.F.);
#2846=ADVANCED_FACE('',(#259),#2721,.F.);
#2847=ADVANCED_FACE('',(#260),#2722,.F.);
#2848=ADVANCED_FACE('',(#261),#2723,.F.);
#2849=ADVANCED_FACE('',(#262),#2724,.F.);
#2850=ADVANCED_FACE('',(#263),#2725,.F.);
#2851=ADVANCED_FACE('',(#264),#2726,.F.);
#2852=ADVANCED_FACE('',(#265),#2727,.F.);
#2853=ADVANCED_FACE('',(#266),#2728,.F.);
#2854=ADVANCED_FACE('',(#267),#2729,.F.);
#2855=ADVANCED_FACE('',(#268),#2730,.F.);
#2856=ADVANCED_FACE('',(#269),#2731,.F.);
#2857=ADVANCED_FACE('',(#270),#2732,.F.);
#2858=ADVANCED_FACE('',(#271),#2733,.F.);
#2859=ADVANCED_FACE('',(#272),#2734,.F.);
#2860=ADVANCED_FACE('',(#273),#2735,.F.);
#2861=ADVANCED_FACE('',(#274),#2736,.F.);
#2862=ADVANCED_FACE('',(#275),#2737,.F.);
#2863=ADVANCED_FACE('',(#276),#2738,.F.);
#2864=ADVANCED_FACE('',(#277),#2739,.F.);
#2865=ADVANCED_FACE('',(#278),#2740,.F.);
#2866=ADVANCED_FACE('',(#279),#2741,.F.);
#2867=ADVANCED_FACE('',(#280),#2742,.F.);
#2868=ADVANCED_FACE('',(#281),#2743,.F.);
#2869=ADVANCED_FACE('',(#282),#2744,.F.);
#2870=ADVANCED_FACE('',(#283),#2745,.F.);
#2871=ADVANCED_FACE('',(#284),#2746,.F.);
#2872=ADVANCED_FACE('',(#285),#2747,.F.);
#2873=ADVANCED_FACE('',(#286),#2748,.F.);
#2874=ADVANCED_FACE('',(#287),#2749,.F.);
#2875=ADVANCED_FACE('',(#288),#2750,.F.);
#2876=ADVANCED_FACE('',(#289),#2751,.F.);
#2877=ADVANCED_FACE('',(#290),#2752,.F.);
#2878=ADVANCED_FACE('',(#291),#2753,.F.);
#2879=ADVANCED_FACE('',(#292),#2754,.F.);
#2880=ADVANCED_FACE('',(#293),#2755,.F.);
#2881=ADVANCED_FACE('',(#294),#2756,.F.);
#2882=ADVANCED_FACE('',(#295),#2757,.F.);
#2883=ADVANCED_FACE('',(#296),#2758,.F.);
#2884=ADVANCED_FACE('',(#297),#2759,.F.);
#2885=ADVANCED_FACE('',(#298),#2760,.F.);
#2886=ADVANCED_FACE('',(#299),#2761,.F.);
#2887=ADVANCED_FACE('',(#300),#2762,.F.);
#2888=ADVANCED_FACE('',(#301),#2763,.F.);
#2889=ADVANCED_FACE('',(#302),#2764,.F.);
#2890=ADVANCED_FACE('',(#303),#2765,.F.);
#2891=ADVANCED_FACE('',(#304),#2766,.F.);
#2892=ADVANCED_FACE('',(#305),#2767,.F.);
#2893=ADVANCED_FACE('',(#306,#112,#113),#2768,.T.);
#2894=ADVANCED_FACE('',(#307),#2769,.F.);
#2895=ADVANCED_FACE('',(#308,#114),#80,.T.);
#2896=ADVANCED_FACE('',(#309,#115),#81,.F.);
#2897=ADVANCED_FACE('',(#310,#116),#82,.T.);
#2898=ADVANCED_FACE('',(#311),#74,.T.);
#2899=ADVANCED_FACE('',(#312),#83,.T.);
#2900=ADVANCED_FACE('',(#313),#84,.T.);
#2901=ADVANCED_FACE('',(#314),#69,.F.);
#2902=ADVANCED_FACE('',(#315),#2770,.F.);
#2903=ADVANCED_FACE('',(#316),#70,.F.);
#2904=ADVANCED_FACE('',(#317),#2771,.T.);
#2905=ADVANCED_FACE('',(#318),#2772,.F.);
#2906=ADVANCED_FACE('',(#319),#85,.T.);
#2907=ADVANCED_FACE('',(#320),#2773,.F.);
#2908=ADVANCED_FACE('',(#321),#86,.T.);
#2909=ADVANCED_FACE('',(#322),#75,.F.);
#2910=ADVANCED_FACE('',(#323),#76,.T.);
#2964=CLOSED_SHELL('',(#2794,#2795,#2796,#2797,#2798,#2799,#2800,#2801,
#2802,#2803,#2804,#2805,#2806,#2807,#2808,#2809,#2810,#2811,#2812,#2813,
#2814,#2815,#2816,#2817,#2818,#2819,#2820,#2821,#2822,#2823,#2824,#2825,
#2826,#2827,#2828,#2829,#2830,#2831,#2832,#2833,#2834,#2835,#2836,#2837,
#2838,#2839,#2840,#2841,#2842,#2843,#2844,#2845,#2846,#2847,#2848,#2849,
#2850,#2851,#2852,#2853,#2854,#2855,#2856,#2857,#2858,#2859,#2860,#2861,
#2862,#2863,#2864,#2865,#2866,#2867,#2868,#2869,#2870,#2871,#2872,#2873,
#2874,#2875,#2876,#2877,#2878,#2879,#2880,#2881,#2882,#2883,#2884,#2885,
#2886,#2887,#2888,#2889,#2890,#2891,#2892,#2893,#2894,#2895,#2896,#2897,
#2898,#2899,#2900,#2901,#2902,#2903,#2904,#2905,#2906,#2907,#2908,#2909,
#2910));
#3039=AXIS2_PLACEMENT_3D('',#3907,#3280,#3281);
#3040=AXIS2_PLACEMENT_3D('',#3908,#3282,#3283);
#3041=AXIS2_PLACEMENT_3D('',#3933,#3286,#3287);
#3042=AXIS2_PLACEMENT_3D('',#3971,#3289,#3290);
#3043=AXIS2_PLACEMENT_3D('',#4009,#3292,#3293);
#3044=AXIS2_PLACEMENT_3D('',#4047,#3295,#3296);
#3045=AXIS2_PLACEMENT_3D('',#4085,#3298,#3299);
#3046=AXIS2_PLACEMENT_3D('',#4123,#3301,#3302);
#3047=AXIS2_PLACEMENT_3D('',#4161,#3304,#3305);
#3048=AXIS2_PLACEMENT_3D('',#4199,#3307,#3308);
#3049=AXIS2_PLACEMENT_3D('',#4237,#3310,#3311);
#3050=AXIS2_PLACEMENT_3D('',#4275,#3313,#3314);
#3051=AXIS2_PLACEMENT_3D('',#4313,#3316,#3317);
#3052=AXIS2_PLACEMENT_3D('',#4351,#3319,#3320);
#3053=AXIS2_PLACEMENT_3D('',#4389,#3322,#3323);
#3054=AXIS2_PLACEMENT_3D('',#4427,#3325,#3326);
#3055=AXIS2_PLACEMENT_3D('',#4465,#3328,#3329);
#3056=AXIS2_PLACEMENT_3D('',#4503,#3331,#3332);
#3057=AXIS2_PLACEMENT_3D('',#4541,#3334,#3335);
#3058=AXIS2_PLACEMENT_3D('',#4579,#3337,#3338);
#3059=AXIS2_PLACEMENT_3D('',#4617,#3340,#3341);
#3060=AXIS2_PLACEMENT_3D('',#4655,#3343,#3344);
#3061=AXIS2_PLACEMENT_3D('',#4693,#3346,#3347);
#3062=AXIS2_PLACEMENT_3D('',#4731,#3349,#3350);
#3063=AXIS2_PLACEMENT_3D('',#4769,#3352,#3353);
#3064=AXIS2_PLACEMENT_3D('',#4807,#3355,#3356);
#3065=AXIS2_PLACEMENT_3D('',#4845,#3358,#3359);
#3066=AXIS2_PLACEMENT_3D('',#4883,#3361,#3362);
#3067=AXIS2_PLACEMENT_3D('',#4921,#3364,#3365);
#3068=AXIS2_PLACEMENT_3D('',#4959,#3367,#3368);
#3069=AXIS2_PLACEMENT_3D('',#4997,#3370,#3371);
#3070=AXIS2_PLACEMENT_3D('',#5035,#3373,#3374);
#3071=AXIS2_PLACEMENT_3D('',#5073,#3376,#3377);
#3072=AXIS2_PLACEMENT_3D('',#5111,#3379,#3380);
#3073=AXIS2_PLACEMENT_3D('',#5149,#3382,#3383);
#3074=AXIS2_PLACEMENT_3D('',#5187,#3385,#3386);
#3075=AXIS2_PLACEMENT_3D('',#5225,#3388,#3389);
#3076=AXIS2_PLACEMENT_3D('',#5263,#3391,#3392);
#3077=AXIS2_PLACEMENT_3D('',#5301,#3394,#3395);
#3078=AXIS2_PLACEMENT_3D('',#5339,#3397,#3398);
#3079=AXIS2_PLACEMENT_3D('',#5377,#3400,#3401);
#3080=AXIS2_PLACEMENT_3D('',#5415,#3403,#3404);
#3081=AXIS2_PLACEMENT_3D('',#5453,#3406,#3407);
#3082=AXIS2_PLACEMENT_3D('',#5491,#3409,#3410);
#3083=AXIS2_PLACEMENT_3D('',#5529,#3412,#3413);
#3084=AXIS2_PLACEMENT_3D('',#5567,#3415,#3416);
#3085=AXIS2_PLACEMENT_3D('',#5605,#3418,#3419);
#3086=AXIS2_PLACEMENT_3D('',#5643,#3421,#3422);
#3087=AXIS2_PLACEMENT_3D('',#5681,#3424,#3425);
#3088=AXIS2_PLACEMENT_3D('',#5719,#3427,#3428);
#3089=AXIS2_PLACEMENT_3D('',#5757,#3430,#3431);
#3090=AXIS2_PLACEMENT_3D('',#5782,#3434,#3435);
#3091=AXIS2_PLACEMENT_3D('',#5793,#3437,#3438);
#3092=AXIS2_PLACEMENT_3D('',#5801,#3439,#3440);
#3093=AXIS2_PLACEMENT_3D('',#5839,#3442,#3443);
#3094=AXIS2_PLACEMENT_3D('',#5877,#3445,#3446);
#3095=AXIS2_PLACEMENT_3D('',#5915,#3448,#3449);
#3096=AXIS2_PLACEMENT_3D('',#5953,#3451,#3452);
#3097=AXIS2_PLACEMENT_3D('',#5991,#3454,#3455);
#3098=AXIS2_PLACEMENT_3D('',#6029,#3457,#3458);
#3099=AXIS2_PLACEMENT_3D('',#6067,#3460,#3461);
#3100=AXIS2_PLACEMENT_3D('',#6105,#3463,#3464);
#3101=AXIS2_PLACEMENT_3D('',#6143,#3466,#3467);
#3102=AXIS2_PLACEMENT_3D('',#6181,#3469,#3470);
#3103=AXIS2_PLACEMENT_3D('',#6219,#3472,#3473);
#3104=AXIS2_PLACEMENT_3D('',#6257,#3475,#3476);
#3105=AXIS2_PLACEMENT_3D('',#6295,#3478,#3479);
#3106=AXIS2_PLACEMENT_3D('',#6333,#3481,#3482);
#3107=AXIS2_PLACEMENT_3D('',#6371,#3484,#3485);
#3108=AXIS2_PLACEMENT_3D('',#6409,#3487,#3488);
#3109=AXIS2_PLACEMENT_3D('',#6447,#3490,#3491);
#3110=AXIS2_PLACEMENT_3D('',#6485,#3493,#3494);
#3111=AXIS2_PLACEMENT_3D('',#6523,#3496,#3497);
#3112=AXIS2_PLACEMENT_3D('',#6561,#3499,#3500);
#3113=AXIS2_PLACEMENT_3D('',#6599,#3502,#3503);
#3114=AXIS2_PLACEMENT_3D('',#6637,#3505,#3506);
#3115=AXIS2_PLACEMENT_3D('',#6675,#3508,#3509);
#3116=AXIS2_PLACEMENT_3D('',#6713,#3511,#3512);
#3117=AXIS2_PLACEMENT_3D('',#6751,#3514,#3515);
#3118=AXIS2_PLACEMENT_3D('',#6789,#3517,#3518);
#3119=AXIS2_PLACEMENT_3D('',#6827,#3520,#3521);
#3120=AXIS2_PLACEMENT_3D('',#6865,#3523,#3524);
#3121=AXIS2_PLACEMENT_3D('',#6903,#3526,#3527);
#3122=AXIS2_PLACEMENT_3D('',#6941,#3529,#3530);
#3123=AXIS2_PLACEMENT_3D('',#6979,#3532,#3533);
#3124=AXIS2_PLACEMENT_3D('',#7017,#3535,#3536);
#3125=AXIS2_PLACEMENT_3D('',#7055,#3538,#3539);
#3126=AXIS2_PLACEMENT_3D('',#7093,#3541,#3542);
#3127=AXIS2_PLACEMENT_3D('',#7131,#3544,#3545);
#3128=AXIS2_PLACEMENT_3D('',#7169,#3547,#3548);
#3129=AXIS2_PLACEMENT_3D('',#7207,#3550,#3551);
#3130=AXIS2_PLACEMENT_3D('',#7245,#3553,#3554);
#3131=AXIS2_PLACEMENT_3D('',#7283,#3556,#3557);
#3132=AXIS2_PLACEMENT_3D('',#7321,#3559,#3560);
#3133=AXIS2_PLACEMENT_3D('',#7359,#3562,#3563);
#3134=AXIS2_PLACEMENT_3D('',#7397,#3565,#3566);
#3135=AXIS2_PLACEMENT_3D('',#7435,#3568,#3569);
#3136=AXIS2_PLACEMENT_3D('',#7473,#3571,#3572);
#3137=AXIS2_PLACEMENT_3D('',#7511,#3574,#3575);
#3138=AXIS2_PLACEMENT_3D('',#7549,#3577,#3578);
#3139=AXIS2_PLACEMENT_3D('',#7587,#3580,#3581);
#3140=AXIS2_PLACEMENT_3D('',#7589,#3582,#3583);
#3141=AXIS2_PLACEMENT_3D('',#7641,#3587,#3588);
#3142=AXIS2_PLACEMENT_3D('',#7644,#3589,#3590);
#3143=AXIS2_PLACEMENT_3D('',#7645,#3591,#3592);
#3144=AXIS2_PLACEMENT_3D('',#7648,#3594,#3595);
#3145=AXIS2_PLACEMENT_3D('',#7725,#3596,#3597);
#3146=AXIS2_PLACEMENT_3D('',#7760,#3598,#3599);
#3147=AXIS2_PLACEMENT_3D('',#7762,#3600,#3601);
#3148=AXIS2_PLACEMENT_3D('',#7764,#3602,#3603);
#3149=AXIS2_PLACEMENT_3D('',#7765,#3604,#3605);
#3150=AXIS2_PLACEMENT_3D('',#7767,#3606,#3607);
#3151=AXIS2_PLACEMENT_3D('',#7768,#3608,#3609);
#3152=AXIS2_PLACEMENT_3D('',#7769,#3610,#3611);
#3153=AXIS2_PLACEMENT_3D('',#7771,#3612,#3613);
#3154=AXIS2_PLACEMENT_3D('',#7772,#3614,#3615);
#3155=AXIS2_PLACEMENT_3D('',#7774,#3617,#3618);
#3156=AXIS2_PLACEMENT_3D('',#7777,#3621,#3622);
#3157=AXIS2_PLACEMENT_3D('',#9401,#3626,#3627);
#3158=AXIS2_PLACEMENT_3D('',#11036,#3628,#3629);
#3159=AXIS2_PLACEMENT_3D('',#11037,#3630,#3631);
#3160=AXIS2_PLACEMENT_3D('',#11040,#3633,#3634);
#3161=AXIS2_PLACEMENT_3D('',#11041,#3635,#3636);
#3162=AXIS2_PLACEMENT_3D('',#11042,#3637,#3638);
#3163=AXIS2_PLACEMENT_3D('',#11045,#3640,#3641);
#3164=AXIS2_PLACEMENT_3D('',#11046,#3642,#3643);
#3165=AXIS2_PLACEMENT_3D('',#11047,#3644,#3645);
#3166=AXIS2_PLACEMENT_3D('',#11049,#3647,#3648);
#3280=DIRECTION('axis',(0.,0.,1.));
#3281=DIRECTION('refdir',(1.,0.,0.));
#3282=DIRECTION('center_axis',(0.,-1.,0.));
#3283=DIRECTION('ref_axis',(-1.,0.,5.80458639773891E-16));
#3284=DIRECTION('',(0.,-1.,0.));
#3285=DIRECTION('',(0.,-1.,0.));
#3286=DIRECTION('center_axis',(0.,-1.,0.));
#3287=DIRECTION('ref_axis',(-1.,0.,5.80458639773891E-16));
#3288=DIRECTION('',(0.,-1.,0.));
#3289=DIRECTION('center_axis',(0.,-1.,0.));
#3290=DIRECTION('ref_axis',(-1.,0.,5.80458639773891E-16));
#3291=DIRECTION('',(0.,-1.,0.));
#3292=DIRECTION('center_axis',(0.,-1.,0.));
#3293=DIRECTION('ref_axis',(-1.,0.,5.80458639773891E-16));
#3294=DIRECTION('',(0.,-1.,0.));
#3295=DIRECTION('center_axis',(0.,-1.,0.));
#3296=DIRECTION('ref_axis',(-1.,0.,5.80458639773891E-16));
#3297=DIRECTION('',(0.,-1.,0.));
#3298=DIRECTION('center_axis',(0.,-1.,0.));
#3299=DIRECTION('ref_axis',(-1.,0.,5.80458639773891E-16));
#3300=DIRECTION('',(0.,-1.,0.));
#3301=DIRECTION('center_axis',(0.,-1.,0.));
#3302=DIRECTION('ref_axis',(-1.,0.,5.80458639773891E-16));
#3303=DIRECTION('',(0.,-1.,0.));
#3304=DIRECTION('center_axis',(0.,-1.,0.));
#3305=DIRECTION('ref_axis',(-1.,0.,5.80458639773891E-16));
#3306=DIRECTION('',(0.,-1.,0.));
#3307=DIRECTION('center_axis',(0.,-1.,0.));
#3308=DIRECTION('ref_axis',(-1.,0.,5.80458639773891E-16));
#3309=DIRECTION('',(0.,-1.,0.));
#3310=DIRECTION('center_axis',(0.,-1.,0.));
#3311=DIRECTION('ref_axis',(-1.,0.,5.80458639773891E-16));
#3312=DIRECTION('',(0.,-1.,0.));
#3313=DIRECTION('center_axis',(0.,-1.,0.));
#3314=DIRECTION('ref_axis',(-1.,0.,5.80458639773891E-16));
#3315=DIRECTION('',(0.,-1.,0.));
#3316=DIRECTION('center_axis',(0.,-1.,0.));
#3317=DIRECTION('ref_axis',(-1.,0.,5.80458639773891E-16));
#3318=DIRECTION('',(0.,-1.,0.));
#3319=DIRECTION('center_axis',(0.,-1.,0.));
#3320=DIRECTION('ref_axis',(-1.,0.,5.80458639773891E-16));
#3321=DIRECTION('',(0.,-1.,0.));
#3322=DIRECTION('center_axis',(0.,-1.,0.));
#3323=DIRECTION('ref_axis',(-1.,0.,5.80458639773891E-16));
#3324=DIRECTION('',(0.,-1.,0.));
#3325=DIRECTION('center_axis',(0.,-1.,0.));
#3326=DIRECTION('ref_axis',(-1.,0.,5.80458639773891E-16));
#3327=DIRECTION('',(0.,-1.,0.));
#3328=DIRECTION('center_axis',(0.,-1.,0.));
#3329=DIRECTION('ref_axis',(-1.,0.,5.80458639773891E-16));
#3330=DIRECTION('',(0.,-1.,0.));
#3331=DIRECTION('center_axis',(0.,-1.,0.));
#3332=DIRECTION('ref_axis',(-1.,0.,5.80458639773891E-16));
#3333=DIRECTION('',(0.,-1.,0.));
#3334=DIRECTION('center_axis',(0.,-1.,0.));
#3335=DIRECTION('ref_axis',(-1.,0.,5.80458639773891E-16));
#3336=DIRECTION('',(0.,-1.,0.));
#3337=DIRECTION('center_axis',(0.,-1.,0.));
#3338=DIRECTION('ref_axis',(-1.,0.,5.80458639773891E-16));
#3339=DIRECTION('',(0.,-1.,0.));
#3340=DIRECTION('center_axis',(0.,-1.,0.));
#3341=DIRECTION('ref_axis',(-1.,0.,5.80458639773891E-16));
#3342=DIRECTION('',(0.,-1.,0.));
#3343=DIRECTION('center_axis',(0.,-1.,0.));
#3344=DIRECTION('ref_axis',(-1.,0.,5.80458639773891E-16));
#3345=DIRECTION('',(0.,-1.,0.));
#3346=DIRECTION('center_axis',(0.,-1.,0.));
#3347=DIRECTION('ref_axis',(-1.,0.,5.80458639773891E-16));
#3348=DIRECTION('',(0.,-1.,0.));
#3349=DIRECTION('center_axis',(0.,-1.,0.));
#3350=DIRECTION('ref_axis',(-1.,0.,5.80458639773891E-16));
#3351=DIRECTION('',(0.,-1.,0.));
#3352=DIRECTION('center_axis',(0.,-1.,0.));
#3353=DIRECTION('ref_axis',(-1.,0.,5.80458639773891E-16));
#3354=DIRECTION('',(0.,-1.,0.));
#3355=DIRECTION('center_axis',(0.,-1.,0.));
#3356=DIRECTION('ref_axis',(-1.,0.,5.80458639773891E-16));
#3357=DIRECTION('',(0.,-1.,0.));
#3358=DIRECTION('center_axis',(0.,-1.,0.));
#3359=DIRECTION('ref_axis',(-1.,0.,5.80458639773891E-16));
#3360=DIRECTION('',(0.,-1.,0.));
#3361=DIRECTION('center_axis',(0.,-1.,0.));
#3362=DIRECTION('ref_axis',(-1.,0.,5.80458639773891E-16));
#3363=DIRECTION('',(0.,-1.,0.));
#3364=DIRECTION('center_axis',(0.,-1.,0.));
#3365=DIRECTION('ref_axis',(-1.,0.,5.80458639773891E-16));
#3366=DIRECTION('',(0.,-1.,0.));
#3367=DIRECTION('center_axis',(0.,-1.,0.));
#3368=DIRECTION('ref_axis',(-1.,0.,5.80458639773891E-16));
#3369=DIRECTION('',(0.,-1.,0.));
#3370=DIRECTION('center_axis',(0.,-1.,0.));
#3371=DIRECTION('ref_axis',(-1.,0.,5.80458639773891E-16));
#3372=DIRECTION('',(0.,-1.,0.));
#3373=DIRECTION('center_axis',(0.,-1.,0.));
#3374=DIRECTION('ref_axis',(-1.,0.,5.80458639773891E-16));
#3375=DIRECTION('',(0.,-1.,0.));
#3376=DIRECTION('center_axis',(0.,-1.,0.));
#3377=DIRECTION('ref_axis',(-1.,0.,5.80458639773891E-16));
#3378=DIRECTION('',(0.,-1.,0.));
#3379=DIRECTION('center_axis',(0.,-1.,0.));
#3380=DIRECTION('ref_axis',(-1.,0.,5.80458639773891E-16));
#3381=DIRECTION('',(0.,-1.,0.));
#3382=DIRECTION('center_axis',(0.,-1.,0.));
#3383=DIRECTION('ref_axis',(-1.,0.,5.80458639773891E-16));
#3384=DIRECTION('',(0.,-1.,0.));
#3385=DIRECTION('center_axis',(0.,-1.,0.));
#3386=DIRECTION('ref_axis',(-1.,0.,5.80458639773891E-16));
#3387=DIRECTION('',(0.,-1.,0.));
#3388=DIRECTION('center_axis',(0.,-1.,0.));
#3389=DIRECTION('ref_axis',(-1.,0.,5.80458639773891E-16));
#3390=DIRECTION('',(0.,-1.,0.));
#3391=DIRECTION('center_axis',(0.,-1.,0.));
#3392=DIRECTION('ref_axis',(-1.,0.,5.80458639773891E-16));
#3393=DIRECTION('',(0.,-1.,0.));
#3394=DIRECTION('center_axis',(0.,-1.,0.));
#3395=DIRECTION('ref_axis',(-1.,0.,5.80458639773891E-16));
#3396=DIRECTION('',(0.,-1.,0.));
#3397=DIRECTION('center_axis',(0.,-1.,0.));
#3398=DIRECTION('ref_axis',(-1.,0.,5.80458639773891E-16));
#3399=DIRECTION('',(0.,-1.,0.));
#3400=DIRECTION('center_axis',(0.,-1.,0.));
#3401=DIRECTION('ref_axis',(-1.,0.,5.80458639773891E-16));
#3402=DIRECTION('',(0.,-1.,0.));
#3403=DIRECTION('center_axis',(0.,-1.,0.));
#3404=DIRECTION('ref_axis',(-1.,0.,5.80458639773891E-16));
#3405=DIRECTION('',(0.,-1.,0.));
#3406=DIRECTION('center_axis',(0.,-1.,0.));
#3407=DIRECTION('ref_axis',(-1.,0.,5.80458639773891E-16));
#3408=DIRECTION('',(0.,-1.,0.));
#3409=DIRECTION('center_axis',(0.,-1.,0.));
#3410=DIRECTION('ref_axis',(-1.,0.,5.80458639773891E-16));
#3411=DIRECTION('',(0.,-1.,0.));
#3412=DIRECTION('center_axis',(0.,-1.,0.));
#3413=DIRECTION('ref_axis',(-1.,0.,5.80458639773891E-16));
#3414=DIRECTION('',(0.,-1.,0.));
#3415=DIRECTION('center_axis',(0.,-1.,0.));
#3416=DIRECTION('ref_axis',(-1.,0.,5.80458639773891E-16));
#3417=DIRECTION('',(0.,-1.,0.));
#3418=DIRECTION('center_axis',(0.,-1.,0.));
#3419=DIRECTION('ref_axis',(-1.,0.,5.80458639773891E-16));
#3420=DIRECTION('',(0.,-1.,0.));
#3421=DIRECTION('center_axis',(0.,-1.,0.));
#3422=DIRECTION('ref_axis',(-1.,0.,5.80458639773891E-16));
#3423=DIRECTION('',(0.,-1.,0.));
#3424=DIRECTION('center_axis',(0.,-1.,0.));
#3425=DIRECTION('ref_axis',(-1.,0.,5.80458639773891E-16));
#3426=DIRECTION('',(0.,-1.,0.));
#3427=DIRECTION('center_axis',(0.,-1.,0.));
#3428=DIRECTION('ref_axis',(-1.,0.,5.80458639773891E-16));
#3429=DIRECTION('',(0.,-1.,0.));
#3430=DIRECTION('center_axis',(0.,-1.,0.));
#3431=DIRECTION('ref_axis',(-1.,0.,5.80458639773891E-16));
#3432=DIRECTION('',(0.,-1.,0.));
#3433=DIRECTION('',(0.,1.,0.));
#3434=DIRECTION('center_axis',(0.,-1.,0.));
#3435=DIRECTION('ref_axis',(0.,0.,-1.));
#3436=DIRECTION('',(0.,-1.,0.));
#3437=DIRECTION('center_axis',(0.,1.,0.));
#3438=DIRECTION('ref_axis',(0.,0.,1.));
#3439=DIRECTION('center_axis',(0.,-1.,0.));
#3440=DIRECTION('ref_axis',(0.,0.,-1.));
#3441=DIRECTION('',(0.,-1.,0.));
#3442=DIRECTION('center_axis',(0.,-1.,0.));
#3443=DIRECTION('ref_axis',(0.,0.,-1.));
#3444=DIRECTION('',(0.,-1.,0.));
#3445=DIRECTION('center_axis',(0.,-1.,0.));
#3446=DIRECTION('ref_axis',(0.,0.,-1.));
#3447=DIRECTION('',(0.,-1.,0.));
#3448=DIRECTION('center_axis',(0.,-1.,0.));
#3449=DIRECTION('ref_axis',(0.,0.,-1.));
#3450=DIRECTION('',(0.,-1.,0.));
#3451=DIRECTION('center_axis',(0.,-1.,0.));
#3452=DIRECTION('ref_axis',(0.,0.,-1.));
#3453=DIRECTION('',(0.,-1.,0.));
#3454=DIRECTION('center_axis',(0.,-1.,0.));
#3455=DIRECTION('ref_axis',(0.,0.,-1.));
#3456=DIRECTION('',(0.,-1.,0.));
#3457=DIRECTION('center_axis',(0.,-1.,0.));
#3458=DIRECTION('ref_axis',(0.,0.,-1.));
#3459=DIRECTION('',(0.,-1.,0.));
#3460=DIRECTION('center_axis',(0.,-1.,0.));
#3461=DIRECTION('ref_axis',(0.,0.,-1.));
#3462=DIRECTION('',(0.,-1.,0.));
#3463=DIRECTION('center_axis',(0.,-1.,0.));
#3464=DIRECTION('ref_axis',(0.,0.,-1.));
#3465=DIRECTION('',(0.,-1.,0.));
#3466=DIRECTION('center_axis',(0.,-1.,0.));
#3467=DIRECTION('ref_axis',(0.,0.,-1.));
#3468=DIRECTION('',(0.,-1.,0.));
#3469=DIRECTION('center_axis',(0.,-1.,0.));
#3470=DIRECTION('ref_axis',(0.,0.,-1.));
#3471=DIRECTION('',(0.,-1.,0.));
#3472=DIRECTION('center_axis',(0.,-1.,0.));
#3473=DIRECTION('ref_axis',(0.,0.,-1.));
#3474=DIRECTION('',(0.,-1.,0.));
#3475=DIRECTION('center_axis',(0.,-1.,0.));
#3476=DIRECTION('ref_axis',(0.,0.,-1.));
#3477=DIRECTION('',(0.,-1.,0.));
#3478=DIRECTION('center_axis',(0.,-1.,0.));
#3479=DIRECTION('ref_axis',(0.,0.,-1.));
#3480=DIRECTION('',(0.,-1.,0.));
#3481=DIRECTION('center_axis',(0.,-1.,0.));
#3482=DIRECTION('ref_axis',(0.,0.,-1.));
#3483=DIRECTION('',(0.,-1.,0.));
#3484=DIRECTION('center_axis',(0.,-1.,0.));
#3485=DIRECTION('ref_axis',(0.,0.,-1.));
#3486=DIRECTION('',(0.,-1.,0.));
#3487=DIRECTION('center_axis',(0.,-1.,0.));
#3488=DIRECTION('ref_axis',(0.,0.,-1.));
#3489=DIRECTION('',(0.,-1.,0.));
#3490=DIRECTION('center_axis',(0.,-1.,0.));
#3491=DIRECTION('ref_axis',(0.,0.,-1.));
#3492=DIRECTION('',(0.,-1.,0.));
#3493=DIRECTION('center_axis',(0.,-1.,0.));
#3494=DIRECTION('ref_axis',(0.,0.,-1.));
#3495=DIRECTION('',(0.,-1.,0.));
#3496=DIRECTION('center_axis',(0.,-1.,0.));
#3497=DIRECTION('ref_axis',(0.,0.,-1.));
#3498=DIRECTION('',(0.,-1.,0.));
#3499=DIRECTION('center_axis',(0.,-1.,0.));
#3500=DIRECTION('ref_axis',(0.,0.,-1.));
#3501=DIRECTION('',(0.,-1.,0.));
#3502=DIRECTION('center_axis',(0.,-1.,0.));
#3503=DIRECTION('ref_axis',(0.,0.,-1.));
#3504=DIRECTION('',(0.,-1.,0.));
#3505=DIRECTION('center_axis',(0.,-1.,0.));
#3506=DIRECTION('ref_axis',(0.,0.,-1.));
#3507=DIRECTION('',(0.,-1.,0.));
#3508=DIRECTION('center_axis',(0.,-1.,0.));
#3509=DIRECTION('ref_axis',(0.,0.,-1.));
#3510=DIRECTION('',(0.,-1.,0.));
#3511=DIRECTION('center_axis',(0.,-1.,0.));
#3512=DIRECTION('ref_axis',(0.,0.,-1.));
#3513=DIRECTION('',(0.,-1.,0.));
#3514=DIRECTION('center_axis',(0.,-1.,0.));
#3515=DIRECTION('ref_axis',(0.,0.,-1.));
#3516=DIRECTION('',(0.,-1.,0.));
#3517=DIRECTION('center_axis',(0.,-1.,0.));
#3518=DIRECTION('ref_axis',(0.,0.,-1.));
#3519=DIRECTION('',(0.,-1.,0.));
#3520=DIRECTION('center_axis',(0.,-1.,0.));
#3521=DIRECTION('ref_axis',(0.,0.,-1.));
#3522=DIRECTION('',(0.,-1.,0.));
#3523=DIRECTION('center_axis',(0.,-1.,0.));
#3524=DIRECTION('ref_axis',(0.,0.,-1.));
#3525=DIRECTION('',(0.,-1.,0.));
#3526=DIRECTION('center_axis',(0.,-1.,0.));
#3527=DIRECTION('ref_axis',(0.,0.,-1.));
#3528=DIRECTION('',(0.,-1.,0.));
#3529=DIRECTION('center_axis',(0.,-1.,0.));
#3530=DIRECTION('ref_axis',(0.,0.,-1.));
#3531=DIRECTION('',(0.,-1.,0.));
#3532=DIRECTION('center_axis',(0.,-1.,0.));
#3533=DIRECTION('ref_axis',(0.,0.,-1.));
#3534=DIRECTION('',(0.,-1.,0.));
#3535=DIRECTION('center_axis',(0.,-1.,0.));
#3536=DIRECTION('ref_axis',(0.,0.,-1.));
#3537=DIRECTION('',(0.,-1.,0.));
#3538=DIRECTION('center_axis',(0.,-1.,0.));
#3539=DIRECTION('ref_axis',(0.,0.,-1.));
#3540=DIRECTION('',(0.,-1.,0.));
#3541=DIRECTION('center_axis',(0.,-1.,0.));
#3542=DIRECTION('ref_axis',(0.,0.,-1.));
#3543=DIRECTION('',(0.,-1.,0.));
#3544=DIRECTION('center_axis',(0.,-1.,0.));
#3545=DIRECTION('ref_axis',(0.,0.,-1.));
#3546=DIRECTION('',(0.,-1.,0.));
#3547=DIRECTION('center_axis',(0.,-1.,0.));
#3548=DIRECTION('ref_axis',(0.,0.,-1.));
#3549=DIRECTION('',(0.,-1.,0.));
#3550=DIRECTION('center_axis',(0.,-1.,0.));
#3551=DIRECTION('ref_axis',(0.,0.,-1.));
#3552=DIRECTION('',(0.,-1.,0.));
#3553=DIRECTION('center_axis',(0.,-1.,0.));
#3554=DIRECTION('ref_axis',(0.,0.,-1.));
#3555=DIRECTION('',(0.,-1.,0.));
#3556=DIRECTION('center_axis',(0.,-1.,0.));
#3557=DIRECTION('ref_axis',(0.,0.,-1.));
#3558=DIRECTION('',(0.,-1.,0.));
#3559=DIRECTION('center_axis',(0.,-1.,0.));
#3560=DIRECTION('ref_axis',(0.,0.,-1.));
#3561=DIRECTION('',(0.,-1.,0.));
#3562=DIRECTION('center_axis',(0.,-1.,0.));
#3563=DIRECTION('ref_axis',(0.,0.,-1.));
#3564=DIRECTION('',(0.,-1.,0.));
#3565=DIRECTION('center_axis',(0.,-1.,0.));
#3566=DIRECTION('ref_axis',(0.,0.,-1.));
#3567=DIRECTION('',(0.,-1.,0.));
#3568=DIRECTION('center_axis',(0.,-1.,0.));
#3569=DIRECTION('ref_axis',(0.,0.,-1.));
#3570=DIRECTION('',(0.,-1.,0.));
#3571=DIRECTION('center_axis',(0.,-1.,0.));
#3572=DIRECTION('ref_axis',(0.,0.,-1.));
#3573=DIRECTION('',(0.,-1.,0.));
#3574=DIRECTION('center_axis',(0.,-1.,0.));
#3575=DIRECTION('ref_axis',(0.,0.,-1.));
#3576=DIRECTION('',(0.,-1.,0.));
#3577=DIRECTION('center_axis',(0.,-1.,0.));
#3578=DIRECTION('ref_axis',(0.,0.,-1.));
#3579=DIRECTION('',(0.,-1.,0.));
#3580=DIRECTION('center_axis',(0.,-1.,0.));
#3581=DIRECTION('ref_axis',(0.,0.,-1.));
#3582=DIRECTION('center_axis',(0.,1.,0.));
#3583=DIRECTION('ref_axis',(0.,0.,1.));
#3584=DIRECTION('',(0.,-1.,0.));
#3585=DIRECTION('',(0.,-1.,0.));
#3586=DIRECTION('',(0.,-1.,0.));
#3587=DIRECTION('center_axis',(0.,-1.,0.));
#3588=DIRECTION('ref_axis',(0.,0.,-1.));
#3589=DIRECTION('center_axis',(0.,1.,0.));
#3590=DIRECTION('ref_axis',(0.,0.,1.));
#3591=DIRECTION('center_axis',(0.,1.,0.));
#3592=DIRECTION('ref_axis',(0.,0.,1.));
#3593=DIRECTION('',(0.,1.,0.));
#3594=DIRECTION('center_axis',(0.,1.,0.));
#3595=DIRECTION('ref_axis',(0.,0.,1.));
#3596=DIRECTION('center_axis',(0.,-1.,0.));
#3597=DIRECTION('ref_axis',(0.,0.,-1.));
#3598=DIRECTION('center_axis',(0.,1.,0.));
#3599=DIRECTION('ref_axis',(0.,0.,1.));
#3600=DIRECTION('center_axis',(0.,1.,0.));
#3601=DIRECTION('ref_axis',(0.,0.,1.));
#3602=DIRECTION('center_axis',(0.,1.,0.));
#3603=DIRECTION('ref_axis',(0.,0.,1.));
#3604=DIRECTION('center_axis',(0.,1.,0.));
#3605=DIRECTION('ref_axis',(0.,0.,1.));
#3606=DIRECTION('center_axis',(0.,1.,0.));
#3607=DIRECTION('ref_axis',(0.,0.,1.));
#3608=DIRECTION('center_axis',(0.,1.,0.));
#3609=DIRECTION('ref_axis',(0.,0.,1.));
#3610=DIRECTION('center_axis',(0.,1.,0.));
#3611=DIRECTION('ref_axis',(0.,0.,1.));
#3612=DIRECTION('center_axis',(0.,1.,0.));
#3613=DIRECTION('ref_axis',(0.,0.,1.));
#3614=DIRECTION('center_axis',(0.,-1.,0.));
#3615=DIRECTION('ref_axis',(0.,0.,-1.));
#3616=DIRECTION('',(5.17558101501968E-17,0.906307787036649,-0.422618261740701));
#3617=DIRECTION('center_axis',(0.,0.,1.));
#3618=DIRECTION('ref_axis',(1.,0.,0.));
#3619=DIRECTION('',(-0.866025403784442,0.499999999999994,0.));
#3620=DIRECTION('',(0.866025403784448,0.499999999999983,0.));
#3621=DIRECTION('center_axis',(0.,0.,-1.));
#3622=DIRECTION('ref_axis',(-1.,0.,0.));
#3623=DIRECTION('',(0.866025403784442,-0.499999999999995,0.));
#3624=DIRECTION('',(-0.866025403784444,-0.499999999999991,0.));
#3625=DIRECTION('',(0.,1.,0.));
#3626=DIRECTION('center_axis',(0.,-1.,0.));
#3627=DIRECTION('ref_axis',(-1.,0.,5.80458639773891E-16));
#3628=DIRECTION('center_axis',(0.,-1.,0.));
#3629=DIRECTION('ref_axis',(0.923879529047881,0.,0.382683440726491));
#3630=DIRECTION('center_axis',(-1.,0.,0.));
#3631=DIRECTION('ref_axis',(0.,0.,1.));
#3632=DIRECTION('',(-1.,0.,0.));
#3633=DIRECTION('center_axis',(-1.,0.,0.));
#3634=DIRECTION('ref_axis',(0.,0.,1.));
#3635=DIRECTION('center_axis',(1.,0.,0.));
#3636=DIRECTION('ref_axis',(0.,0.,-1.));
#3637=DIRECTION('center_axis',(1.,0.,0.));
#3638=DIRECTION('ref_axis',(0.,0.,1.));
#3639=DIRECTION('',(1.,0.,0.));
#3640=DIRECTION('center_axis',(-1.,0.,0.));
#3641=DIRECTION('ref_axis',(0.,0.,1.));
#3642=DIRECTION('center_axis',(-1.,0.,0.));
#3643=DIRECTION('ref_axis',(0.,0.,1.));
#3644=DIRECTION('center_axis',(0.,1.,0.));
#3645=DIRECTION('ref_axis',(0.,0.,1.));
#3646=DIRECTION('',(-1.70437892618156E-17,0.99026806874157,-0.139173100960066));
#3647=DIRECTION('center_axis',(0.,1.,0.));
#3648=DIRECTION('ref_axis',(0.,0.,1.));
#3649=DIRECTION('',(6.1232339957367E-17,-0.866025403784442,0.499999999999995));
#3907=CARTESIAN_POINT('',(0.,0.,0.));
#3908=CARTESIAN_POINT('Origin',(-7.105427357601E-14,49.5625000013656,-6.0924204042587E-14));
#3909=CARTESIAN_POINT('',(104.958734125,0.187500001365581,-6.0924204042587E-14));
#3910=CARTESIAN_POINT('',(104.958734125,-0.0624999986344188,-6.0924204042587E-14));
#3911=CARTESIAN_POINT('',(104.958734125,49.5625000013656,-1.089946703063E-13));
#3912=CARTESIAN_POINT('',(-104.958734125,-0.562499998634419,0.));
#3913=CARTESIAN_POINT('Ctrl Pts',(104.958734125,-0.0624999986344188,-1.28537377788739E-14));
#3914=CARTESIAN_POINT('Ctrl Pts',(104.958734125,-0.124999998634419,43.4753311640868));
#3915=CARTESIAN_POINT('Ctrl Pts',(74.2170326445434,-0.187499998634419,74.2170326445434));
#3916=CARTESIAN_POINT('Ctrl Pts',(43.4753311640869,-0.249999998634419,104.958734125));
#3917=CARTESIAN_POINT('Ctrl Pts',(1.92806066683109E-14,-0.312499998634419,
104.958734125));
#3918=CARTESIAN_POINT('Ctrl Pts',(-43.4753311640868,-0.374999998634419,
104.958734125));
#3919=CARTESIAN_POINT('Ctrl Pts',(-74.2170326445434,-0.437499998634419,
74.2170326445434));
#3920=CARTESIAN_POINT('Ctrl Pts',(-104.958734125,-0.499999998634419,43.4753311640869));
#3921=CARTESIAN_POINT('Ctrl Pts',(-104.958734125,-0.562499998634419,0.));
#3922=CARTESIAN_POINT('',(-104.958734125,-0.312499998634419,0.));
#3923=CARTESIAN_POINT('',(-104.958734125,-0.312499998634419,0.));
#3924=CARTESIAN_POINT('Ctrl Pts',(104.958734125,0.187500001365581,-1.28537377788739E-14));
#3925=CARTESIAN_POINT('Ctrl Pts',(104.958734125,0.125000001365581,43.4753311640868));
#3926=CARTESIAN_POINT('Ctrl Pts',(74.2170326445434,0.0625000013655813,74.2170326445434));
#3927=CARTESIAN_POINT('Ctrl Pts',(43.4753311640869,1.36558125918285E-9,
104.958734125));
#3928=CARTESIAN_POINT('Ctrl Pts',(1.92806066683109E-14,-0.0624999986344188,
104.958734125));
#3929=CARTESIAN_POINT('Ctrl Pts',(-43.4753311640868,-0.124999998634419,
104.958734125));
#3930=CARTESIAN_POINT('Ctrl Pts',(-74.2170326445434,-0.187499998634419,
74.2170326445434));
#3931=CARTESIAN_POINT('Ctrl Pts',(-104.958734125,-0.249999998634419,43.4753311640869));
#3932=CARTESIAN_POINT('Ctrl Pts',(-104.958734125,-0.312499998634419,0.));
#3933=CARTESIAN_POINT('Origin',(-7.105427357601E-14,49.5625000013656,-6.0924204042587E-14));
#3934=CARTESIAN_POINT('',(104.958734125,1.18750000136558,-6.0924204042587E-14));
#3935=CARTESIAN_POINT('',(104.958734125,0.937500001365582,-6.0924204042587E-14));
#3936=CARTESIAN_POINT('',(104.958734125,49.5625000013656,-1.089946703063E-13));
#3937=CARTESIAN_POINT('Ctrl Pts',(104.958734125,0.937500001365582,-1.28537377788739E-14));
#3938=CARTESIAN_POINT('Ctrl Pts',(104.958734125,0.875000001365582,43.4753311640868));
#3939=CARTESIAN_POINT('Ctrl Pts',(74.2170326445434,0.812500001365582,74.2170326445434));
#3940=CARTESIAN_POINT('Ctrl Pts',(43.4753311640869,0.750000001365582,104.958734125));
#3941=CARTESIAN_POINT('Ctrl Pts',(1.92806066683109E-14,0.687500001365582,
104.958734125));
#3942=CARTESIAN_POINT('Ctrl Pts',(-43.4753311640868,0.625000001365582,104.958734125));
#3943=CARTESIAN_POINT('Ctrl Pts',(-74.2170326445434,0.562500001365582,74.2170326445434));
#3944=CARTESIAN_POINT('Ctrl Pts',(-104.958734125,0.500000001365582,43.4753311640869));
#3945=CARTESIAN_POINT('Ctrl Pts',(-104.958734125,0.437500001365582,0.));
#3946=CARTESIAN_POINT('Ctrl Pts',(-104.958734125,0.375000001365582,-43.4753311640868));
#3947=CARTESIAN_POINT('Ctrl Pts',(-74.2170326445434,0.312500001365582,-74.2170326445434));
#3948=CARTESIAN_POINT('Ctrl Pts',(-43.4753311640868,0.250000001365581,-104.958734125));
#3949=CARTESIAN_POINT('Ctrl Pts',(-6.42686888943697E-15,0.187500001365581,
-104.958734125));
#3950=CARTESIAN_POINT('Ctrl Pts',(43.4753311640868,0.125000001365581,-104.958734125));
#3951=CARTESIAN_POINT('Ctrl Pts',(74.2170326445434,0.0625000013655813,-74.2170326445434));
#3952=CARTESIAN_POINT('Ctrl Pts',(104.958734125,1.36558125918285E-9,-43.4753311640868));
#3953=CARTESIAN_POINT('Ctrl Pts',(104.958734125,-0.0624999986344188,-1.28537377788739E-14));
#3954=CARTESIAN_POINT('Ctrl Pts',(104.958734125,1.18750000136558,-1.28537377788739E-14));
#3955=CARTESIAN_POINT('Ctrl Pts',(104.958734125,1.12500000136558,43.4753311640868));
#3956=CARTESIAN_POINT('Ctrl Pts',(74.2170326445434,1.06250000136558,74.2170326445434));
#3957=CARTESIAN_POINT('Ctrl Pts',(43.4753311640869,1.00000000136558,104.958734125));
#3958=CARTESIAN_POINT('Ctrl Pts',(1.92806066683109E-14,0.937500001365582,
104.958734125));
#3959=CARTESIAN_POINT('Ctrl Pts',(-43.4753311640868,0.875000001365582,104.958734125));
#3960=CARTESIAN_POINT('Ctrl Pts',(-74.2170326445434,0.812500001365582,74.2170326445434));
#3961=CARTESIAN_POINT('Ctrl Pts',(-104.958734125,0.750000001365582,43.4753311640869));
#3962=CARTESIAN_POINT('Ctrl Pts',(-104.958734125,0.687500001365582,0.));
#3963=CARTESIAN_POINT('Ctrl Pts',(-104.958734125,0.625000001365582,-43.4753311640868));
#3964=CARTESIAN_POINT('Ctrl Pts',(-74.2170326445434,0.562500001365582,-74.2170326445434));
#3965=CARTESIAN_POINT('Ctrl Pts',(-43.4753311640868,0.500000001365582,-104.958734125));
#3966=CARTESIAN_POINT('Ctrl Pts',(-6.42686888943697E-15,0.437500001365582,
-104.958734125));
#3967=CARTESIAN_POINT('Ctrl Pts',(43.4753311640868,0.375000001365582,-104.958734125));
#3968=CARTESIAN_POINT('Ctrl Pts',(74.2170326445434,0.312500001365582,-74.2170326445434));
#3969=CARTESIAN_POINT('Ctrl Pts',(104.958734125,0.250000001365581,-43.4753311640868));
#3970=CARTESIAN_POINT('Ctrl Pts',(104.958734125,0.187500001365581,-1.28537377788739E-14));
#3971=CARTESIAN_POINT('Origin',(-7.105427357601E-14,49.5625000013656,-6.0924204042587E-14));
#3972=CARTESIAN_POINT('',(104.958734125,2.18750000136558,-6.0924204042587E-14));
#3973=CARTESIAN_POINT('',(104.958734125,1.93750000136558,-6.0924204042587E-14));
#3974=CARTESIAN_POINT('',(104.958734125,49.5625000013656,-1.089946703063E-13));
#3975=CARTESIAN_POINT('Ctrl Pts',(104.958734125,1.93750000136558,-1.28537377788739E-14));
#3976=CARTESIAN_POINT('Ctrl Pts',(104.958734125,1.87500000136558,43.4753311640868));
#3977=CARTESIAN_POINT('Ctrl Pts',(74.2170326445434,1.81250000136558,74.2170326445434));
#3978=CARTESIAN_POINT('Ctrl Pts',(43.4753311640869,1.75000000136558,104.958734125));
#3979=CARTESIAN_POINT('Ctrl Pts',(1.92806066683109E-14,1.68750000136558,
104.958734125));
#3980=CARTESIAN_POINT('Ctrl Pts',(-43.4753311640868,1.62500000136558,104.958734125));
#3981=CARTESIAN_POINT('Ctrl Pts',(-74.2170326445434,1.56250000136558,74.2170326445434));
#3982=CARTESIAN_POINT('Ctrl Pts',(-104.958734125,1.50000000136558,43.4753311640869));
#3983=CARTESIAN_POINT('Ctrl Pts',(-104.958734125,1.43750000136558,0.));
#3984=CARTESIAN_POINT('Ctrl Pts',(-104.958734125,1.37500000136558,-43.4753311640868));
#3985=CARTESIAN_POINT('Ctrl Pts',(-74.2170326445434,1.31250000136558,-74.2170326445434));
#3986=CARTESIAN_POINT('Ctrl Pts',(-43.4753311640868,1.25000000136558,-104.958734125));
#3987=CARTESIAN_POINT('Ctrl Pts',(-6.42686888943697E-15,1.18750000136558,
-104.958734125));
#3988=CARTESIAN_POINT('Ctrl Pts',(43.4753311640868,1.12500000136558,-104.958734125));
#3989=CARTESIAN_POINT('Ctrl Pts',(74.2170326445434,1.06250000136558,-74.2170326445434));
#3990=CARTESIAN_POINT('Ctrl Pts',(104.958734125,1.00000000136558,-43.4753311640868));
#3991=CARTESIAN_POINT('Ctrl Pts',(104.958734125,0.937500001365582,-1.28537377788739E-14));
#3992=CARTESIAN_POINT('Ctrl Pts',(104.958734125,2.18750000136558,-1.28537377788739E-14));
#3993=CARTESIAN_POINT('Ctrl Pts',(104.958734125,2.12500000136558,43.4753311640868));
#3994=CARTESIAN_POINT('Ctrl Pts',(74.2170326445434,2.06250000136558,74.2170326445434));
#3995=CARTESIAN_POINT('Ctrl Pts',(43.4753311640869,2.00000000136558,104.958734125));
#3996=CARTESIAN_POINT('Ctrl Pts',(1.92806066683109E-14,1.93750000136558,
104.958734125));
#3997=CARTESIAN_POINT('Ctrl Pts',(-43.4753311640868,1.87500000136558,104.958734125));
#3998=CARTESIAN_POINT('Ctrl Pts',(-74.2170326445434,1.81250000136558,74.2170326445434));
#3999=CARTESIAN_POINT('Ctrl Pts',(-104.958734125,1.75000000136558,43.4753311640869));
#4000=CARTESIAN_POINT('Ctrl Pts',(-104.958734125,1.68750000136558,0.));
#4001=CARTESIAN_POINT('Ctrl Pts',(-104.958734125,1.62500000136558,-43.4753311640868));
#4002=CARTESIAN_POINT('Ctrl Pts',(-74.2170326445434,1.56250000136558,-74.2170326445434));
#4003=CARTESIAN_POINT('Ctrl Pts',(-43.4753311640868,1.50000000136558,-104.958734125));
#4004=CARTESIAN_POINT('Ctrl Pts',(-6.42686888943697E-15,1.43750000136558,
-104.958734125));
#4005=CARTESIAN_POINT('Ctrl Pts',(43.4753311640868,1.37500000136558,-104.958734125));
#4006=CARTESIAN_POINT('Ctrl Pts',(74.2170326445434,1.31250000136558,-74.2170326445434));
#4007=CARTESIAN_POINT('Ctrl Pts',(104.958734125,1.25000000136558,-43.4753311640868));
#4008=CARTESIAN_POINT('Ctrl Pts',(104.958734125,1.18750000136558,-1.28537377788739E-14));
#4009=CARTESIAN_POINT('Origin',(-7.105427357601E-14,49.5625000013656,-6.0924204042587E-14));
#4010=CARTESIAN_POINT('',(104.958734125,3.18750000136558,-6.0924204042587E-14));
#4011=CARTESIAN_POINT('',(104.958734125,2.93750000136558,-6.0924204042587E-14));
#4012=CARTESIAN_POINT('',(104.958734125,49.5625000013656,-1.089946703063E-13));
#4013=CARTESIAN_POINT('Ctrl Pts',(104.958734125,2.93750000136558,-1.28537377788739E-14));
#4014=CARTESIAN_POINT('Ctrl Pts',(104.958734125,2.87500000136558,43.4753311640868));
#4015=CARTESIAN_POINT('Ctrl Pts',(74.2170326445434,2.81250000136558,74.2170326445434));
#4016=CARTESIAN_POINT('Ctrl Pts',(43.4753311640869,2.75000000136558,104.958734125));
#4017=CARTESIAN_POINT('Ctrl Pts',(1.92806066683109E-14,2.68750000136558,
104.958734125));
#4018=CARTESIAN_POINT('Ctrl Pts',(-43.4753311640868,2.62500000136558,104.958734125));
#4019=CARTESIAN_POINT('Ctrl Pts',(-74.2170326445434,2.56250000136558,74.2170326445434));
#4020=CARTESIAN_POINT('Ctrl Pts',(-104.958734125,2.50000000136558,43.4753311640869));
#4021=CARTESIAN_POINT('Ctrl Pts',(-104.958734125,2.43750000136558,0.));
#4022=CARTESIAN_POINT('Ctrl Pts',(-104.958734125,2.37500000136558,-43.4753311640868));
#4023=CARTESIAN_POINT('Ctrl Pts',(-74.2170326445434,2.31250000136558,-74.2170326445434));
#4024=CARTESIAN_POINT('Ctrl Pts',(-43.4753311640868,2.25000000136558,-104.958734125));
#4025=CARTESIAN_POINT('Ctrl Pts',(-6.42686888943697E-15,2.18750000136558,
-104.958734125));
#4026=CARTESIAN_POINT('Ctrl Pts',(43.4753311640868,2.12500000136558,-104.958734125));
#4027=CARTESIAN_POINT('Ctrl Pts',(74.2170326445434,2.06250000136558,-74.2170326445434));
#4028=CARTESIAN_POINT('Ctrl Pts',(104.958734125,2.00000000136558,-43.4753311640868));
#4029=CARTESIAN_POINT('Ctrl Pts',(104.958734125,1.93750000136558,-1.28537377788739E-14));
#4030=CARTESIAN_POINT('Ctrl Pts',(104.958734125,3.18750000136558,-1.28537377788739E-14));
#4031=CARTESIAN_POINT('Ctrl Pts',(104.958734125,3.12500000136558,43.4753311640868));
#4032=CARTESIAN_POINT('Ctrl Pts',(74.2170326445434,3.06250000136558,74.2170326445434));
#4033=CARTESIAN_POINT('Ctrl Pts',(43.4753311640869,3.00000000136558,104.958734125));
#4034=CARTESIAN_POINT('Ctrl Pts',(1.92806066683109E-14,2.93750000136558,
104.958734125));
#4035=CARTESIAN_POINT('Ctrl Pts',(-43.4753311640868,2.87500000136558,104.958734125));
#4036=CARTESIAN_POINT('Ctrl Pts',(-74.2170326445434,2.81250000136558,74.2170326445434));
#4037=CARTESIAN_POINT('Ctrl Pts',(-104.958734125,2.75000000136558,43.4753311640869));
#4038=CARTESIAN_POINT('Ctrl Pts',(-104.958734125,2.68750000136558,0.));
#4039=CARTESIAN_POINT('Ctrl Pts',(-104.958734125,2.62500000136558,-43.4753311640868));
#4040=CARTESIAN_POINT('Ctrl Pts',(-74.2170326445434,2.56250000136558,-74.2170326445434));
#4041=CARTESIAN_POINT('Ctrl Pts',(-43.4753311640868,2.50000000136558,-104.958734125));
#4042=CARTESIAN_POINT('Ctrl Pts',(-6.42686888943697E-15,2.43750000136558,
-104.958734125));
#4043=CARTESIAN_POINT('Ctrl Pts',(43.4753311640868,2.37500000136558,-104.958734125));
#4044=CARTESIAN_POINT('Ctrl Pts',(74.2170326445434,2.31250000136558,-74.2170326445434));
#4045=CARTESIAN_POINT('Ctrl Pts',(104.958734125,2.25000000136558,-43.4753311640868));
#4046=CARTESIAN_POINT('Ctrl Pts',(104.958734125,2.18750000136558,-1.28537377788739E-14));
#4047=CARTESIAN_POINT('Origin',(-7.105427357601E-14,49.5625000013656,-6.0924204042587E-14));
#4048=CARTESIAN_POINT('',(104.958734125,4.18750000136558,-6.0924204042587E-14));
#4049=CARTESIAN_POINT('',(104.958734125,3.93750000136558,-6.0924204042587E-14));
#4050=CARTESIAN_POINT('',(104.958734125,49.5625000013656,-1.089946703063E-13));
#4051=CARTESIAN_POINT('Ctrl Pts',(104.958734125,3.93750000136558,-1.28537377788739E-14));
#4052=CARTESIAN_POINT('Ctrl Pts',(104.958734125,3.87500000136558,43.4753311640868));
#4053=CARTESIAN_POINT('Ctrl Pts',(74.2170326445434,3.81250000136558,74.2170326445434));
#4054=CARTESIAN_POINT('Ctrl Pts',(43.4753311640869,3.75000000136558,104.958734125));
#4055=CARTESIAN_POINT('Ctrl Pts',(1.92806066683109E-14,3.68750000136558,
104.958734125));
#4056=CARTESIAN_POINT('Ctrl Pts',(-43.4753311640868,3.62500000136558,104.958734125));
#4057=CARTESIAN_POINT('Ctrl Pts',(-74.2170326445434,3.56250000136558,74.2170326445434));
#4058=CARTESIAN_POINT('Ctrl Pts',(-104.958734125,3.50000000136558,43.4753311640869));
#4059=CARTESIAN_POINT('Ctrl Pts',(-104.958734125,3.43750000136558,0.));
#4060=CARTESIAN_POINT('Ctrl Pts',(-104.958734125,3.37500000136558,-43.4753311640868));
#4061=CARTESIAN_POINT('Ctrl Pts',(-74.2170326445434,3.31250000136558,-74.2170326445434));
#4062=CARTESIAN_POINT('Ctrl Pts',(-43.4753311640868,3.25000000136558,-104.958734125));
#4063=CARTESIAN_POINT('Ctrl Pts',(-6.42686888943697E-15,3.18750000136558,
-104.958734125));
#4064=CARTESIAN_POINT('Ctrl Pts',(43.4753311640868,3.12500000136558,-104.958734125));
#4065=CARTESIAN_POINT('Ctrl Pts',(74.2170326445434,3.06250000136558,-74.2170326445434));
#4066=CARTESIAN_POINT('Ctrl Pts',(104.958734125,3.00000000136558,-43.4753311640868));
#4067=CARTESIAN_POINT('Ctrl Pts',(104.958734125,2.93750000136558,-1.28537377788739E-14));
#4068=CARTESIAN_POINT('Ctrl Pts',(104.958734125,4.18750000136558,-1.28537377788739E-14));
#4069=CARTESIAN_POINT('Ctrl Pts',(104.958734125,4.12500000136558,43.4753311640868));
#4070=CARTESIAN_POINT('Ctrl Pts',(74.2170326445434,4.06250000136558,74.2170326445434));
#4071=CARTESIAN_POINT('Ctrl Pts',(43.4753311640869,4.00000000136558,104.958734125));
#4072=CARTESIAN_POINT('Ctrl Pts',(1.92806066683109E-14,3.93750000136558,
104.958734125));
#4073=CARTESIAN_POINT('Ctrl Pts',(-43.4753311640868,3.87500000136558,104.958734125));
#4074=CARTESIAN_POINT('Ctrl Pts',(-74.2170326445434,3.81250000136558,74.2170326445434));
#4075=CARTESIAN_POINT('Ctrl Pts',(-104.958734125,3.75000000136558,43.4753311640869));
#4076=CARTESIAN_POINT('Ctrl Pts',(-104.958734125,3.68750000136558,0.));
#4077=CARTESIAN_POINT('Ctrl Pts',(-104.958734125,3.62500000136558,-43.4753311640868));
#4078=CARTESIAN_POINT('Ctrl Pts',(-74.2170326445434,3.56250000136558,-74.2170326445434));
#4079=CARTESIAN_POINT('Ctrl Pts',(-43.4753311640868,3.50000000136558,-104.958734125));
#4080=CARTESIAN_POINT('Ctrl Pts',(-6.42686888943697E-15,3.43750000136558,
-104.958734125));
#4081=CARTESIAN_POINT('Ctrl Pts',(43.4753311640868,3.37500000136558,-104.958734125));
#4082=CARTESIAN_POINT('Ctrl Pts',(74.2170326445434,3.31250000136558,-74.2170326445434));
#4083=CARTESIAN_POINT('Ctrl Pts',(104.958734125,3.25000000136558,-43.4753311640868));
#4084=CARTESIAN_POINT('Ctrl Pts',(104.958734125,3.18750000136558,-1.28537377788739E-14));
#4085=CARTESIAN_POINT('Origin',(-7.105427357601E-14,49.5625000013656,-6.0924204042587E-14));
#4086=CARTESIAN_POINT('',(104.958734125,5.18750000136559,-6.0924204042587E-14));
#4087=CARTESIAN_POINT('',(104.958734125,4.93750000136559,-6.0924204042587E-14));
#4088=CARTESIAN_POINT('',(104.958734125,49.5625000013656,-1.089946703063E-13));
#4089=CARTESIAN_POINT('Ctrl Pts',(104.958734125,4.93750000136559,-1.28537377788739E-14));
#4090=CARTESIAN_POINT('Ctrl Pts',(104.958734125,4.87500000136559,43.4753311640868));
#4091=CARTESIAN_POINT('Ctrl Pts',(74.2170326445434,4.81250000136559,74.2170326445434));
#4092=CARTESIAN_POINT('Ctrl Pts',(43.4753311640869,4.75000000136558,104.958734125));
#4093=CARTESIAN_POINT('Ctrl Pts',(1.92806066683109E-14,4.68750000136558,
104.958734125));
#4094=CARTESIAN_POINT('Ctrl Pts',(-43.4753311640868,4.62500000136559,104.958734125));
#4095=CARTESIAN_POINT('Ctrl Pts',(-74.2170326445434,4.56250000136558,74.2170326445434));
#4096=CARTESIAN_POINT('Ctrl Pts',(-104.958734125,4.50000000136558,43.4753311640869));
#4097=CARTESIAN_POINT('Ctrl Pts',(-104.958734125,4.43750000136558,0.));
#4098=CARTESIAN_POINT('Ctrl Pts',(-104.958734125,4.37500000136558,-43.4753311640868));
#4099=CARTESIAN_POINT('Ctrl Pts',(-74.2170326445434,4.31250000136558,-74.2170326445434));
#4100=CARTESIAN_POINT('Ctrl Pts',(-43.4753311640868,4.25000000136558,-104.958734125));
#4101=CARTESIAN_POINT('Ctrl Pts',(-6.42686888943697E-15,4.18750000136558,
-104.958734125));
#4102=CARTESIAN_POINT('Ctrl Pts',(43.4753311640868,4.12500000136558,-104.958734125));
#4103=CARTESIAN_POINT('Ctrl Pts',(74.2170326445434,4.06250000136558,-74.2170326445434));
#4104=CARTESIAN_POINT('Ctrl Pts',(104.958734125,4.00000000136558,-43.4753311640868));
#4105=CARTESIAN_POINT('Ctrl Pts',(104.958734125,3.93750000136558,-1.28537377788739E-14));
#4106=CARTESIAN_POINT('Ctrl Pts',(104.958734125,5.18750000136559,-1.28537377788739E-14));
#4107=CARTESIAN_POINT('Ctrl Pts',(104.958734125,5.12500000136559,43.4753311640868));
#4108=CARTESIAN_POINT('Ctrl Pts',(74.2170326445434,5.06250000136559,74.2170326445434));
#4109=CARTESIAN_POINT('Ctrl Pts',(43.4753311640869,5.00000000136558,104.958734125));
#4110=CARTESIAN_POINT('Ctrl Pts',(1.92806066683109E-14,4.93750000136559,
104.958734125));
#4111=CARTESIAN_POINT('Ctrl Pts',(-43.4753311640868,4.87500000136559,104.958734125));
#4112=CARTESIAN_POINT('Ctrl Pts',(-74.2170326445434,4.81250000136559,74.2170326445434));
#4113=CARTESIAN_POINT('Ctrl Pts',(-104.958734125,4.75000000136558,43.4753311640869));
#4114=CARTESIAN_POINT('Ctrl Pts',(-104.958734125,4.68750000136558,0.));
#4115=CARTESIAN_POINT('Ctrl Pts',(-104.958734125,4.62500000136559,-43.4753311640868));
#4116=CARTESIAN_POINT('Ctrl Pts',(-74.2170326445434,4.56250000136558,-74.2170326445434));
#4117=CARTESIAN_POINT('Ctrl Pts',(-43.4753311640868,4.50000000136558,-104.958734125));
#4118=CARTESIAN_POINT('Ctrl Pts',(-6.42686888943697E-15,4.43750000136558,
-104.958734125));
#4119=CARTESIAN_POINT('Ctrl Pts',(43.4753311640868,4.37500000136558,-104.958734125));
#4120=CARTESIAN_POINT('Ctrl Pts',(74.2170326445434,4.31250000136558,-74.2170326445434));
#4121=CARTESIAN_POINT('Ctrl Pts',(104.958734125,4.25000000136558,-43.4753311640868));
#4122=CARTESIAN_POINT('Ctrl Pts',(104.958734125,4.18750000136558,-1.28537377788739E-14));
#4123=CARTESIAN_POINT('Origin',(-7.105427357601E-14,49.5625000013656,-6.0924204042587E-14));
#4124=CARTESIAN_POINT('',(104.958734125,6.18750000136558,-6.0924204042587E-14));
#4125=CARTESIAN_POINT('',(104.958734125,5.93750000136558,-6.0924204042587E-14));
#4126=CARTESIAN_POINT('',(104.958734125,49.5625000013656,-1.089946703063E-13));
#4127=CARTESIAN_POINT('Ctrl Pts',(104.958734125,5.93750000136558,-1.28537377788739E-14));
#4128=CARTESIAN_POINT('Ctrl Pts',(104.958734125,5.87500000136558,43.4753311640868));
#4129=CARTESIAN_POINT('Ctrl Pts',(74.2170326445434,5.81250000136558,74.2170326445434));
#4130=CARTESIAN_POINT('Ctrl Pts',(43.4753311640869,5.75000000136558,104.958734125));
#4131=CARTESIAN_POINT('Ctrl Pts',(1.92806066683109E-14,5.68750000136558,
104.958734125));
#4132=CARTESIAN_POINT('Ctrl Pts',(-43.4753311640868,5.62500000136558,104.958734125));
#4133=CARTESIAN_POINT('Ctrl Pts',(-74.2170326445434,5.56250000136558,74.2170326445434));
#4134=CARTESIAN_POINT('Ctrl Pts',(-104.958734125,5.50000000136558,43.4753311640869));
#4135=CARTESIAN_POINT('Ctrl Pts',(-104.958734125,5.43750000136559,0.));
#4136=CARTESIAN_POINT('Ctrl Pts',(-104.958734125,5.37500000136559,-43.4753311640868));
#4137=CARTESIAN_POINT('Ctrl Pts',(-74.2170326445434,5.31250000136558,-74.2170326445434));
#4138=CARTESIAN_POINT('Ctrl Pts',(-43.4753311640868,5.25000000136559,-104.958734125));
#4139=CARTESIAN_POINT('Ctrl Pts',(-6.42686888943697E-15,5.18750000136559,
-104.958734125));
#4140=CARTESIAN_POINT('Ctrl Pts',(43.4753311640868,5.12500000136559,-104.958734125));
#4141=CARTESIAN_POINT('Ctrl Pts',(74.2170326445434,5.06250000136559,-74.2170326445434));
#4142=CARTESIAN_POINT('Ctrl Pts',(104.958734125,5.00000000136558,-43.4753311640868));
#4143=CARTESIAN_POINT('Ctrl Pts',(104.958734125,4.93750000136559,-1.28537377788739E-14));
#4144=CARTESIAN_POINT('Ctrl Pts',(104.958734125,6.18750000136558,-1.28537377788739E-14));
#4145=CARTESIAN_POINT('Ctrl Pts',(104.958734125,6.12500000136558,43.4753311640868));
#4146=CARTESIAN_POINT('Ctrl Pts',(74.2170326445434,6.06250000136558,74.2170326445434));
#4147=CARTESIAN_POINT('Ctrl Pts',(43.4753311640869,6.00000000136558,104.958734125));
#4148=CARTESIAN_POINT('Ctrl Pts',(1.92806066683109E-14,5.93750000136558,
104.958734125));
#4149=CARTESIAN_POINT('Ctrl Pts',(-43.4753311640868,5.87500000136558,104.958734125));
#4150=CARTESIAN_POINT('Ctrl Pts',(-74.2170326445434,5.81250000136558,74.2170326445434));
#4151=CARTESIAN_POINT('Ctrl Pts',(-104.958734125,5.75000000136558,43.4753311640869));
#4152=CARTESIAN_POINT('Ctrl Pts',(-104.958734125,5.68750000136559,0.));
#4153=CARTESIAN_POINT('Ctrl Pts',(-104.958734125,5.62500000136559,-43.4753311640868));
#4154=CARTESIAN_POINT('Ctrl Pts',(-74.2170326445434,5.56250000136559,-74.2170326445434));
#4155=CARTESIAN_POINT('Ctrl Pts',(-43.4753311640868,5.50000000136559,-104.958734125));
#4156=CARTESIAN_POINT('Ctrl Pts',(-6.42686888943697E-15,5.43750000136559,
-104.958734125));
#4157=CARTESIAN_POINT('Ctrl Pts',(43.4753311640868,5.37500000136559,-104.958734125));
#4158=CARTESIAN_POINT('Ctrl Pts',(74.2170326445434,5.31250000136558,-74.2170326445434));
#4159=CARTESIAN_POINT('Ctrl Pts',(104.958734125,5.25000000136559,-43.4753311640868));
#4160=CARTESIAN_POINT('Ctrl Pts',(104.958734125,5.18750000136559,-1.28537377788739E-14));
#4161=CARTESIAN_POINT('Origin',(-7.105427357601E-14,49.5625000013656,-6.0924204042587E-14));
#4162=CARTESIAN_POINT('',(104.958734125,7.18750000136558,-6.0924204042587E-14));
#4163=CARTESIAN_POINT('',(104.958734125,6.93750000136558,-6.0924204042587E-14));
#4164=CARTESIAN_POINT('',(104.958734125,49.5625000013656,-1.089946703063E-13));
#4165=CARTESIAN_POINT('Ctrl Pts',(104.958734125,6.93750000136558,-1.28537377788739E-14));
#4166=CARTESIAN_POINT('Ctrl Pts',(104.958734125,6.87500000136558,43.4753311640868));
#4167=CARTESIAN_POINT('Ctrl Pts',(74.2170326445434,6.81250000136558,74.2170326445434));
#4168=CARTESIAN_POINT('Ctrl Pts',(43.4753311640869,6.75000000136558,104.958734125));
#4169=CARTESIAN_POINT('Ctrl Pts',(1.92806066683109E-14,6.68750000136558,
104.958734125));
#4170=CARTESIAN_POINT('Ctrl Pts',(-43.4753311640868,6.62500000136558,104.958734125));
#4171=CARTESIAN_POINT('Ctrl Pts',(-74.2170326445434,6.56250000136558,74.2170326445434));
#4172=CARTESIAN_POINT('Ctrl Pts',(-104.958734125,6.50000000136558,43.4753311640869));
#4173=CARTESIAN_POINT('Ctrl Pts',(-104.958734125,6.43750000136558,0.));
#4174=CARTESIAN_POINT('Ctrl Pts',(-104.958734125,6.37500000136558,-43.4753311640868));
#4175=CARTESIAN_POINT('Ctrl Pts',(-74.2170326445434,6.31250000136558,-74.2170326445434));
#4176=CARTESIAN_POINT('Ctrl Pts',(-43.4753311640868,6.25000000136558,-104.958734125));
#4177=CARTESIAN_POINT('Ctrl Pts',(-6.42686888943697E-15,6.18750000136558,
-104.958734125));
#4178=CARTESIAN_POINT('Ctrl Pts',(43.4753311640868,6.12500000136558,-104.958734125));
#4179=CARTESIAN_POINT('Ctrl Pts',(74.2170326445434,6.06250000136558,-74.2170326445434));
#4180=CARTESIAN_POINT('Ctrl Pts',(104.958734125,6.00000000136558,-43.4753311640868));
#4181=CARTESIAN_POINT('Ctrl Pts',(104.958734125,5.93750000136558,-1.28537377788739E-14));
#4182=CARTESIAN_POINT('Ctrl Pts',(104.958734125,7.18750000136558,-1.28537377788739E-14));
#4183=CARTESIAN_POINT('Ctrl Pts',(104.958734125,7.12500000136558,43.4753311640868));
#4184=CARTESIAN_POINT('Ctrl Pts',(74.2170326445434,7.06250000136558,74.2170326445434));
#4185=CARTESIAN_POINT('Ctrl Pts',(43.4753311640869,7.00000000136558,104.958734125));
#4186=CARTESIAN_POINT('Ctrl Pts',(1.92806066683109E-14,6.93750000136558,
104.958734125));
#4187=CARTESIAN_POINT('Ctrl Pts',(-43.4753311640868,6.87500000136558,104.958734125));
#4188=CARTESIAN_POINT('Ctrl Pts',(-74.2170326445434,6.81250000136558,74.2170326445434));
#4189=CARTESIAN_POINT('Ctrl Pts',(-104.958734125,6.75000000136558,43.4753311640869));
#4190=CARTESIAN_POINT('Ctrl Pts',(-104.958734125,6.68750000136558,0.));
#4191=CARTESIAN_POINT('Ctrl Pts',(-104.958734125,6.62500000136558,-43.4753311640868));
#4192=CARTESIAN_POINT('Ctrl Pts',(-74.2170326445434,6.56250000136558,-74.2170326445434));
#4193=CARTESIAN_POINT('Ctrl Pts',(-43.4753311640868,6.50000000136558,-104.958734125));
#4194=CARTESIAN_POINT('Ctrl Pts',(-6.42686888943697E-15,6.43750000136558,
-104.958734125));
#4195=CARTESIAN_POINT('Ctrl Pts',(43.4753311640868,6.37500000136558,-104.958734125));
#4196=CARTESIAN_POINT('Ctrl Pts',(74.2170326445434,6.31250000136558,-74.2170326445434));
#4197=CARTESIAN_POINT('Ctrl Pts',(104.958734125,6.25000000136558,-43.4753311640868));
#4198=CARTESIAN_POINT('Ctrl Pts',(104.958734125,6.18750000136558,-1.28537377788739E-14));
#4199=CARTESIAN_POINT('Origin',(-7.105427357601E-14,49.5625000013656,-6.0924204042587E-14));
#4200=CARTESIAN_POINT('',(104.958734125,8.18750000136558,-6.0924204042587E-14));
#4201=CARTESIAN_POINT('',(104.958734125,7.93750000136558,-6.0924204042587E-14));
#4202=CARTESIAN_POINT('',(104.958734125,49.5625000013656,-1.089946703063E-13));
#4203=CARTESIAN_POINT('Ctrl Pts',(104.958734125,7.93750000136558,-1.28537377788739E-14));
#4204=CARTESIAN_POINT('Ctrl Pts',(104.958734125,7.87500000136558,43.4753311640868));
#4205=CARTESIAN_POINT('Ctrl Pts',(74.2170326445434,7.81250000136558,74.2170326445434));
#4206=CARTESIAN_POINT('Ctrl Pts',(43.4753311640869,7.75000000136558,104.958734125));
#4207=CARTESIAN_POINT('Ctrl Pts',(1.92806066683109E-14,7.68750000136558,
104.958734125));
#4208=CARTESIAN_POINT('Ctrl Pts',(-43.4753311640868,7.62500000136558,104.958734125));
#4209=CARTESIAN_POINT('Ctrl Pts',(-74.2170326445434,7.56250000136558,74.2170326445434));
#4210=CARTESIAN_POINT('Ctrl Pts',(-104.958734125,7.50000000136558,43.4753311640869));
#4211=CARTESIAN_POINT('Ctrl Pts',(-104.958734125,7.43750000136558,0.));
#4212=CARTESIAN_POINT('Ctrl Pts',(-104.958734125,7.37500000136558,-43.4753311640868));
#4213=CARTESIAN_POINT('Ctrl Pts',(-74.2170326445434,7.31250000136558,-74.2170326445434));
#4214=CARTESIAN_POINT('Ctrl Pts',(-43.4753311640868,7.25000000136558,-104.958734125));
#4215=CARTESIAN_POINT('Ctrl Pts',(-6.42686888943697E-15,7.18750000136558,
-104.958734125));
#4216=CARTESIAN_POINT('Ctrl Pts',(43.4753311640868,7.12500000136558,-104.958734125));
#4217=CARTESIAN_POINT('Ctrl Pts',(74.2170326445434,7.06250000136558,-74.2170326445434));
#4218=CARTESIAN_POINT('Ctrl Pts',(104.958734125,7.00000000136558,-43.4753311640868));
#4219=CARTESIAN_POINT('Ctrl Pts',(104.958734125,6.93750000136558,-1.28537377788739E-14));
#4220=CARTESIAN_POINT('Ctrl Pts',(104.958734125,8.18750000136558,-1.28537377788739E-14));
#4221=CARTESIAN_POINT('Ctrl Pts',(104.958734125,8.12500000136558,43.4753311640868));
#4222=CARTESIAN_POINT('Ctrl Pts',(74.2170326445434,8.06250000136558,74.2170326445434));
#4223=CARTESIAN_POINT('Ctrl Pts',(43.4753311640869,8.00000000136558,104.958734125));
#4224=CARTESIAN_POINT('Ctrl Pts',(1.92806066683109E-14,7.93750000136558,
104.958734125));
#4225=CARTESIAN_POINT('Ctrl Pts',(-43.4753311640868,7.87500000136558,104.958734125));
#4226=CARTESIAN_POINT('Ctrl Pts',(-74.2170326445434,7.81250000136558,74.2170326445434));
#4227=CARTESIAN_POINT('Ctrl Pts',(-104.958734125,7.75000000136558,43.4753311640869));
#4228=CARTESIAN_POINT('Ctrl Pts',(-104.958734125,7.68750000136558,0.));
#4229=CARTESIAN_POINT('Ctrl Pts',(-104.958734125,7.62500000136558,-43.4753311640868));
#4230=CARTESIAN_POINT('Ctrl Pts',(-74.2170326445434,7.56250000136558,-74.2170326445434));
#4231=CARTESIAN_POINT('Ctrl Pts',(-43.4753311640868,7.50000000136558,-104.958734125));
#4232=CARTESIAN_POINT('Ctrl Pts',(-6.42686888943697E-15,7.43750000136558,
-104.958734125));
#4233=CARTESIAN_POINT('Ctrl Pts',(43.4753311640868,7.37500000136558,-104.958734125));
#4234=CARTESIAN_POINT('Ctrl Pts',(74.2170326445434,7.31250000136558,-74.2170326445434));
#4235=CARTESIAN_POINT('Ctrl Pts',(104.958734125,7.25000000136558,-43.4753311640868));
#4236=CARTESIAN_POINT('Ctrl Pts',(104.958734125,7.18750000136558,-1.28537377788739E-14));
#4237=CARTESIAN_POINT('Origin',(-7.105427357601E-14,49.5625000013656,-6.0924204042587E-14));
#4238=CARTESIAN_POINT('',(104.958734125,9.18750000136558,-6.0924204042587E-14));
#4239=CARTESIAN_POINT('',(104.958734125,8.93750000136558,-6.0924204042587E-14));
#4240=CARTESIAN_POINT('',(104.958734125,49.5625000013656,-1.089946703063E-13));
#4241=CARTESIAN_POINT('Ctrl Pts',(104.958734125,8.93750000136558,-1.28537377788739E-14));
#4242=CARTESIAN_POINT('Ctrl Pts',(104.958734125,8.87500000136558,43.4753311640868));
#4243=CARTESIAN_POINT('Ctrl Pts',(74.2170326445434,8.81250000136558,74.2170326445434));
#4244=CARTESIAN_POINT('Ctrl Pts',(43.4753311640869,8.75000000136558,104.958734125));
#4245=CARTESIAN_POINT('Ctrl Pts',(1.92806066683109E-14,8.68750000136558,
104.958734125));
#4246=CARTESIAN_POINT('Ctrl Pts',(-43.4753311640868,8.62500000136558,104.958734125));
#4247=CARTESIAN_POINT('Ctrl Pts',(-74.2170326445434,8.56250000136558,74.2170326445434));
#4248=CARTESIAN_POINT('Ctrl Pts',(-104.958734125,8.50000000136558,43.4753311640869));
#4249=CARTESIAN_POINT('Ctrl Pts',(-104.958734125,8.43750000136558,0.));
#4250=CARTESIAN_POINT('Ctrl Pts',(-104.958734125,8.37500000136558,-43.4753311640868));
#4251=CARTESIAN_POINT('Ctrl Pts',(-74.2170326445434,8.31250000136558,-74.2170326445434));
#4252=CARTESIAN_POINT('Ctrl Pts',(-43.4753311640868,8.25000000136558,-104.958734125));
#4253=CARTESIAN_POINT('Ctrl Pts',(-6.42686888943697E-15,8.18750000136558,
-104.958734125));
#4254=CARTESIAN_POINT('Ctrl Pts',(43.4753311640868,8.12500000136558,-104.958734125));
#4255=CARTESIAN_POINT('Ctrl Pts',(74.2170326445434,8.06250000136558,-74.2170326445434));
#4256=CARTESIAN_POINT('Ctrl Pts',(104.958734125,8.00000000136558,-43.4753311640868));
#4257=CARTESIAN_POINT('Ctrl Pts',(104.958734125,7.93750000136558,-1.28537377788739E-14));
#4258=CARTESIAN_POINT('Ctrl Pts',(104.958734125,9.18750000136558,-1.28537377788739E-14));
#4259=CARTESIAN_POINT('Ctrl Pts',(104.958734125,9.12500000136558,43.4753311640868));
#4260=CARTESIAN_POINT('Ctrl Pts',(74.2170326445434,9.06250000136558,74.2170326445434));
#4261=CARTESIAN_POINT('Ctrl Pts',(43.4753311640869,9.00000000136558,104.958734125));
#4262=CARTESIAN_POINT('Ctrl Pts',(1.92806066683109E-14,8.93750000136558,
104.958734125));
#4263=CARTESIAN_POINT('Ctrl Pts',(-43.4753311640868,8.87500000136558,104.958734125));
#4264=CARTESIAN_POINT('Ctrl Pts',(-74.2170326445434,8.81250000136558,74.2170326445434));
#4265=CARTESIAN_POINT('Ctrl Pts',(-104.958734125,8.75000000136558,43.4753311640869));
#4266=CARTESIAN_POINT('Ctrl Pts',(-104.958734125,8.68750000136558,0.));
#4267=CARTESIAN_POINT('Ctrl Pts',(-104.958734125,8.62500000136558,-43.4753311640868));
#4268=CARTESIAN_POINT('Ctrl Pts',(-74.2170326445434,8.56250000136558,-74.2170326445434));
#4269=CARTESIAN_POINT('Ctrl Pts',(-43.4753311640868,8.50000000136558,-104.958734125));
#4270=CARTESIAN_POINT('Ctrl Pts',(-6.42686888943697E-15,8.43750000136558,
-104.958734125));
#4271=CARTESIAN_POINT('Ctrl Pts',(43.4753311640868,8.37500000136558,-104.958734125));
#4272=CARTESIAN_POINT('Ctrl Pts',(74.2170326445434,8.31250000136558,-74.2170326445434));
#4273=CARTESIAN_POINT('Ctrl Pts',(104.958734125,8.25000000136558,-43.4753311640868));
#4274=CARTESIAN_POINT('Ctrl Pts',(104.958734125,8.18750000136558,-1.28537377788739E-14));
#4275=CARTESIAN_POINT('Origin',(-7.105427357601E-14,49.5625000013656,-6.0924204042587E-14));
#4276=CARTESIAN_POINT('',(104.958734125,10.1875000013656,-6.0924204042587E-14));
#4277=CARTESIAN_POINT('',(104.958734125,9.93750000136558,-6.0924204042587E-14));
#4278=CARTESIAN_POINT('',(104.958734125,49.5625000013656,-1.089946703063E-13));
#4279=CARTESIAN_POINT('Ctrl Pts',(104.958734125,9.93750000136558,-1.28537377788739E-14));
#4280=CARTESIAN_POINT('Ctrl Pts',(104.958734125,9.87500000136558,43.4753311640868));
#4281=CARTESIAN_POINT('Ctrl Pts',(74.2170326445434,9.81250000136558,74.2170326445434));
#4282=CARTESIAN_POINT('Ctrl Pts',(43.4753311640869,9.75000000136558,104.958734125));
#4283=CARTESIAN_POINT('Ctrl Pts',(1.92806066683109E-14,9.68750000136558,
104.958734125));
#4284=CARTESIAN_POINT('Ctrl Pts',(-43.4753311640868,9.62500000136558,104.958734125));
#4285=CARTESIAN_POINT('Ctrl Pts',(-74.2170326445434,9.56250000136558,74.2170326445434));
#4286=CARTESIAN_POINT('Ctrl Pts',(-104.958734125,9.50000000136558,43.4753311640869));
#4287=CARTESIAN_POINT('Ctrl Pts',(-104.958734125,9.43750000136558,0.));
#4288=CARTESIAN_POINT('Ctrl Pts',(-104.958734125,9.37500000136558,-43.4753311640868));
#4289=CARTESIAN_POINT('Ctrl Pts',(-74.2170326445434,9.31250000136558,-74.2170326445434));
#4290=CARTESIAN_POINT('Ctrl Pts',(-43.4753311640868,9.25000000136558,-104.958734125));
#4291=CARTESIAN_POINT('Ctrl Pts',(-6.42686888943697E-15,9.18750000136558,
-104.958734125));
#4292=CARTESIAN_POINT('Ctrl Pts',(43.4753311640868,9.12500000136558,-104.958734125));
#4293=CARTESIAN_POINT('Ctrl Pts',(74.2170326445434,9.06250000136558,-74.2170326445434));
#4294=CARTESIAN_POINT('Ctrl Pts',(104.958734125,9.00000000136558,-43.4753311640868));
#4295=CARTESIAN_POINT('Ctrl Pts',(104.958734125,8.93750000136558,-1.28537377788739E-14));
#4296=CARTESIAN_POINT('Ctrl Pts',(104.958734125,10.1875000013656,-1.28537377788739E-14));
#4297=CARTESIAN_POINT('Ctrl Pts',(104.958734125,10.1250000013656,43.4753311640868));
#4298=CARTESIAN_POINT('Ctrl Pts',(74.2170326445434,10.0625000013656,74.2170326445434));
#4299=CARTESIAN_POINT('Ctrl Pts',(43.4753311640869,10.0000000013656,104.958734125));
#4300=CARTESIAN_POINT('Ctrl Pts',(1.92806066683109E-14,9.93750000136558,
104.958734125));
#4301=CARTESIAN_POINT('Ctrl Pts',(-43.4753311640868,9.87500000136558,104.958734125));
#4302=CARTESIAN_POINT('Ctrl Pts',(-74.2170326445434,9.81250000136558,74.2170326445434));
#4303=CARTESIAN_POINT('Ctrl Pts',(-104.958734125,9.75000000136558,43.4753311640869));
#4304=CARTESIAN_POINT('Ctrl Pts',(-104.958734125,9.68750000136558,0.));
#4305=CARTESIAN_POINT('Ctrl Pts',(-104.958734125,9.62500000136558,-43.4753311640868));
#4306=CARTESIAN_POINT('Ctrl Pts',(-74.2170326445434,9.56250000136558,-74.2170326445434));
#4307=CARTESIAN_POINT('Ctrl Pts',(-43.4753311640868,9.50000000136558,-104.958734125));
#4308=CARTESIAN_POINT('Ctrl Pts',(-6.42686888943697E-15,9.43750000136558,
-104.958734125));
#4309=CARTESIAN_POINT('Ctrl Pts',(43.4753311640868,9.37500000136558,-104.958734125));
#4310=CARTESIAN_POINT('Ctrl Pts',(74.2170326445434,9.31250000136558,-74.2170326445434));
#4311=CARTESIAN_POINT('Ctrl Pts',(104.958734125,9.25000000136558,-43.4753311640868));
#4312=CARTESIAN_POINT('Ctrl Pts',(104.958734125,9.18750000136558,-1.28537377788739E-14));
#4313=CARTESIAN_POINT('Origin',(-7.105427357601E-14,49.5625000013656,-6.0924204042587E-14));
#4314=CARTESIAN_POINT('',(104.958734125,11.1875000013656,-6.0924204042587E-14));
#4315=CARTESIAN_POINT('',(104.958734125,10.9375000013656,-6.0924204042587E-14));
#4316=CARTESIAN_POINT('',(104.958734125,49.5625000013656,-1.089946703063E-13));
#4317=CARTESIAN_POINT('Ctrl Pts',(104.958734125,10.9375000013656,-1.28537377788739E-14));
#4318=CARTESIAN_POINT('Ctrl Pts',(104.958734125,10.8750000013656,43.4753311640868));
#4319=CARTESIAN_POINT('Ctrl Pts',(74.2170326445434,10.8125000013656,74.2170326445434));
#4320=CARTESIAN_POINT('Ctrl Pts',(43.4753311640869,10.7500000013656,104.958734125));
#4321=CARTESIAN_POINT('Ctrl Pts',(1.92806066683109E-14,10.6875000013656,
104.958734125));
#4322=CARTESIAN_POINT('Ctrl Pts',(-43.4753311640868,10.6250000013656,104.958734125));
#4323=CARTESIAN_POINT('Ctrl Pts',(-74.2170326445434,10.5625000013656,74.2170326445434));
#4324=CARTESIAN_POINT('Ctrl Pts',(-104.958734125,10.5000000013656,43.4753311640869));
#4325=CARTESIAN_POINT('Ctrl Pts',(-104.958734125,10.4375000013656,0.));
#4326=CARTESIAN_POINT('Ctrl Pts',(-104.958734125,10.3750000013656,-43.4753311640868));
#4327=CARTESIAN_POINT('Ctrl Pts',(-74.2170326445434,10.3125000013656,-74.2170326445434));
#4328=CARTESIAN_POINT('Ctrl Pts',(-43.4753311640868,10.2500000013656,-104.958734125));
#4329=CARTESIAN_POINT('Ctrl Pts',(-6.42686888943697E-15,10.1875000013656,
-104.958734125));
#4330=CARTESIAN_POINT('Ctrl Pts',(43.4753311640868,10.1250000013656,-104.958734125));
#4331=CARTESIAN_POINT('Ctrl Pts',(74.2170326445434,10.0625000013656,-74.2170326445434));
#4332=CARTESIAN_POINT('Ctrl Pts',(104.958734125,10.0000000013656,-43.4753311640868));
#4333=CARTESIAN_POINT('Ctrl Pts',(104.958734125,9.93750000136558,-1.28537377788739E-14));
#4334=CARTESIAN_POINT('Ctrl Pts',(104.958734125,11.1875000013656,-1.28537377788739E-14));
#4335=CARTESIAN_POINT('Ctrl Pts',(104.958734125,11.1250000013656,43.4753311640868));
#4336=CARTESIAN_POINT('Ctrl Pts',(74.2170326445434,11.0625000013656,74.2170326445434));
#4337=CARTESIAN_POINT('Ctrl Pts',(43.4753311640869,11.0000000013656,104.958734125));
#4338=CARTESIAN_POINT('Ctrl Pts',(1.92806066683109E-14,10.9375000013656,
104.958734125));
#4339=CARTESIAN_POINT('Ctrl Pts',(-43.4753311640868,10.8750000013656,104.958734125));
#4340=CARTESIAN_POINT('Ctrl Pts',(-74.2170326445434,10.8125000013656,74.2170326445434));
#4341=CARTESIAN_POINT('Ctrl Pts',(-104.958734125,10.7500000013656,43.4753311640869));
#4342=CARTESIAN_POINT('Ctrl Pts',(-104.958734125,10.6875000013656,0.));
#4343=CARTESIAN_POINT('Ctrl Pts',(-104.958734125,10.6250000013656,-43.4753311640868));
#4344=CARTESIAN_POINT('Ctrl Pts',(-74.2170326445434,10.5625000013656,-74.2170326445434));
#4345=CARTESIAN_POINT('Ctrl Pts',(-43.4753311640868,10.5000000013656,-104.958734125));
#4346=CARTESIAN_POINT('Ctrl Pts',(-6.42686888943697E-15,10.4375000013656,
-104.958734125));
#4347=CARTESIAN_POINT('Ctrl Pts',(43.4753311640868,10.3750000013656,-104.958734125));
#4348=CARTESIAN_POINT('Ctrl Pts',(74.2170326445434,10.3125000013656,-74.2170326445434));
#4349=CARTESIAN_POINT('Ctrl Pts',(104.958734125,10.2500000013656,-43.4753311640868));
#4350=CARTESIAN_POINT('Ctrl Pts',(104.958734125,10.1875000013656,-1.28537377788739E-14));
#4351=CARTESIAN_POINT('Origin',(-7.105427357601E-14,49.5625000013656,-6.0924204042587E-14));
#4352=CARTESIAN_POINT('',(104.958734125,12.1875000013656,-6.0924204042587E-14));
#4353=CARTESIAN_POINT('',(104.958734125,11.9375000013656,-6.0924204042587E-14));
#4354=CARTESIAN_POINT('',(104.958734125,49.5625000013656,-1.089946703063E-13));
#4355=CARTESIAN_POINT('Ctrl Pts',(104.958734125,11.9375000013656,-1.28537377788739E-14));
#4356=CARTESIAN_POINT('Ctrl Pts',(104.958734125,11.8750000013656,43.4753311640868));
#4357=CARTESIAN_POINT('Ctrl Pts',(74.2170326445434,11.8125000013656,74.2170326445434));
#4358=CARTESIAN_POINT('Ctrl Pts',(43.4753311640869,11.7500000013656,104.958734125));
#4359=CARTESIAN_POINT('Ctrl Pts',(1.92806066683109E-14,11.6875000013656,
104.958734125));
#4360=CARTESIAN_POINT('Ctrl Pts',(-43.4753311640868,11.6250000013656,104.958734125));
#4361=CARTESIAN_POINT('Ctrl Pts',(-74.2170326445434,11.5625000013656,74.2170326445434));
#4362=CARTESIAN_POINT('Ctrl Pts',(-104.958734125,11.5000000013656,43.4753311640869));
#4363=CARTESIAN_POINT('Ctrl Pts',(-104.958734125,11.4375000013656,0.));
#4364=CARTESIAN_POINT('Ctrl Pts',(-104.958734125,11.3750000013656,-43.4753311640868));
#4365=CARTESIAN_POINT('Ctrl Pts',(-74.2170326445434,11.3125000013656,-74.2170326445434));
#4366=CARTESIAN_POINT('Ctrl Pts',(-43.4753311640868,11.2500000013656,-104.958734125));
#4367=CARTESIAN_POINT('Ctrl Pts',(-6.42686888943697E-15,11.1875000013656,
-104.958734125));
#4368=CARTESIAN_POINT('Ctrl Pts',(43.4753311640868,11.1250000013656,-104.958734125));
#4369=CARTESIAN_POINT('Ctrl Pts',(74.2170326445434,11.0625000013656,-74.2170326445434));
#4370=CARTESIAN_POINT('Ctrl Pts',(104.958734125,11.0000000013656,-43.4753311640868));
#4371=CARTESIAN_POINT('Ctrl Pts',(104.958734125,10.9375000013656,-1.28537377788739E-14));
#4372=CARTESIAN_POINT('Ctrl Pts',(104.958734125,12.1875000013656,-1.28537377788739E-14));
#4373=CARTESIAN_POINT('Ctrl Pts',(104.958734125,12.1250000013656,43.4753311640868));
#4374=CARTESIAN_POINT('Ctrl Pts',(74.2170326445434,12.0625000013656,74.2170326445434));
#4375=CARTESIAN_POINT('Ctrl Pts',(43.4753311640869,12.0000000013656,104.958734125));
#4376=CARTESIAN_POINT('Ctrl Pts',(1.92806066683109E-14,11.9375000013656,
104.958734125));
#4377=CARTESIAN_POINT('Ctrl Pts',(-43.4753311640868,11.8750000013656,104.958734125));
#4378=CARTESIAN_POINT('Ctrl Pts',(-74.2170326445434,11.8125000013656,74.2170326445434));
#4379=CARTESIAN_POINT('Ctrl Pts',(-104.958734125,11.7500000013656,43.4753311640869));
#4380=CARTESIAN_POINT('Ctrl Pts',(-104.958734125,11.6875000013656,0.));
#4381=CARTESIAN_POINT('Ctrl Pts',(-104.958734125,11.6250000013656,-43.4753311640868));
#4382=CARTESIAN_POINT('Ctrl Pts',(-74.2170326445434,11.5625000013656,-74.2170326445434));
#4383=CARTESIAN_POINT('Ctrl Pts',(-43.4753311640868,11.5000000013656,-104.958734125));
#4384=CARTESIAN_POINT('Ctrl Pts',(-6.42686888943697E-15,11.4375000013656,
-104.958734125));
#4385=CARTESIAN_POINT('Ctrl Pts',(43.4753311640868,11.3750000013656,-104.958734125));
#4386=CARTESIAN_POINT('Ctrl Pts',(74.2170326445434,11.3125000013656,-74.2170326445434));
#4387=CARTESIAN_POINT('Ctrl Pts',(104.958734125,11.2500000013656,-43.4753311640868));
#4388=CARTESIAN_POINT('Ctrl Pts',(104.958734125,11.1875000013656,-1.28537377788739E-14));
#4389=CARTESIAN_POINT('Origin',(-7.105427357601E-14,49.5625000013656,-6.0924204042587E-14));
#4390=CARTESIAN_POINT('',(104.958734125,13.1875000013656,-6.0924204042587E-14));
#4391=CARTESIAN_POINT('',(104.958734125,12.9375000013656,-6.0924204042587E-14));
#4392=CARTESIAN_POINT('',(104.958734125,49.5625000013656,-1.089946703063E-13));
#4393=CARTESIAN_POINT('Ctrl Pts',(104.958734125,12.9375000013656,-1.28537377788739E-14));
#4394=CARTESIAN_POINT('Ctrl Pts',(104.958734125,12.8750000013656,43.4753311640868));
#4395=CARTESIAN_POINT('Ctrl Pts',(74.2170326445434,12.8125000013656,74.2170326445434));
#4396=CARTESIAN_POINT('Ctrl Pts',(43.4753311640869,12.7500000013656,104.958734125));
#4397=CARTESIAN_POINT('Ctrl Pts',(1.92806066683109E-14,12.6875000013656,
104.958734125));
#4398=CARTESIAN_POINT('Ctrl Pts',(-43.4753311640868,12.6250000013656,104.958734125));
#4399=CARTESIAN_POINT('Ctrl Pts',(-74.2170326445434,12.5625000013656,74.2170326445434));
#4400=CARTESIAN_POINT('Ctrl Pts',(-104.958734125,12.5000000013656,43.4753311640869));
#4401=CARTESIAN_POINT('Ctrl Pts',(-104.958734125,12.4375000013656,0.));
#4402=CARTESIAN_POINT('Ctrl Pts',(-104.958734125,12.3750000013656,-43.4753311640868));
#4403=CARTESIAN_POINT('Ctrl Pts',(-74.2170326445434,12.3125000013656,-74.2170326445434));
#4404=CARTESIAN_POINT('Ctrl Pts',(-43.4753311640868,12.2500000013656,-104.958734125));
#4405=CARTESIAN_POINT('Ctrl Pts',(-6.42686888943697E-15,12.1875000013656,
-104.958734125));
#4406=CARTESIAN_POINT('Ctrl Pts',(43.4753311640868,12.1250000013656,-104.958734125));
#4407=CARTESIAN_POINT('Ctrl Pts',(74.2170326445434,12.0625000013656,-74.2170326445434));
#4408=CARTESIAN_POINT('Ctrl Pts',(104.958734125,12.0000000013656,-43.4753311640868));
#4409=CARTESIAN_POINT('Ctrl Pts',(104.958734125,11.9375000013656,-1.28537377788739E-14));
#4410=CARTESIAN_POINT('Ctrl Pts',(104.958734125,13.1875000013656,-1.28537377788739E-14));
#4411=CARTESIAN_POINT('Ctrl Pts',(104.958734125,13.1250000013656,43.4753311640868));
#4412=CARTESIAN_POINT('Ctrl Pts',(74.2170326445434,13.0625000013656,74.2170326445434));
#4413=CARTESIAN_POINT('Ctrl Pts',(43.4753311640869,13.0000000013656,104.958734125));
#4414=CARTESIAN_POINT('Ctrl Pts',(1.92806066683109E-14,12.9375000013656,
104.958734125));
#4415=CARTESIAN_POINT('Ctrl Pts',(-43.4753311640868,12.8750000013656,104.958734125));
#4416=CARTESIAN_POINT('Ctrl Pts',(-74.2170326445434,12.8125000013656,74.2170326445434));
#4417=CARTESIAN_POINT('Ctrl Pts',(-104.958734125,12.7500000013656,43.4753311640869));
#4418=CARTESIAN_POINT('Ctrl Pts',(-104.958734125,12.6875000013656,0.));
#4419=CARTESIAN_POINT('Ctrl Pts',(-104.958734125,12.6250000013656,-43.4753311640868));
#4420=CARTESIAN_POINT('Ctrl Pts',(-74.2170326445434,12.5625000013656,-74.2170326445434));
#4421=CARTESIAN_POINT('Ctrl Pts',(-43.4753311640868,12.5000000013656,-104.958734125));
#4422=CARTESIAN_POINT('Ctrl Pts',(-6.42686888943697E-15,12.4375000013656,
-104.958734125));
#4423=CARTESIAN_POINT('Ctrl Pts',(43.4753311640868,12.3750000013656,-104.958734125));
#4424=CARTESIAN_POINT('Ctrl Pts',(74.2170326445434,12.3125000013656,-74.2170326445434));
#4425=CARTESIAN_POINT('Ctrl Pts',(104.958734125,12.2500000013656,-43.4753311640868));
#4426=CARTESIAN_POINT('Ctrl Pts',(104.958734125,12.1875000013656,-1.28537377788739E-14));
#4427=CARTESIAN_POINT('Origin',(-7.105427357601E-14,49.5625000013656,-6.0924204042587E-14));
#4428=CARTESIAN_POINT('',(104.958734125,14.1875000013656,-6.0924204042587E-14));
#4429=CARTESIAN_POINT('',(104.958734125,13.9375000013656,-6.0924204042587E-14));
#4430=CARTESIAN_POINT('',(104.958734125,49.5625000013656,-1.089946703063E-13));
#4431=CARTESIAN_POINT('Ctrl Pts',(104.958734125,13.9375000013656,-1.28537377788739E-14));
#4432=CARTESIAN_POINT('Ctrl Pts',(104.958734125,13.8750000013656,43.4753311640868));
#4433=CARTESIAN_POINT('Ctrl Pts',(74.2170326445434,13.8125000013656,74.2170326445434));
#4434=CARTESIAN_POINT('Ctrl Pts',(43.4753311640869,13.7500000013656,104.958734125));
#4435=CARTESIAN_POINT('Ctrl Pts',(1.92806066683109E-14,13.6875000013656,
104.958734125));
#4436=CARTESIAN_POINT('Ctrl Pts',(-43.4753311640868,13.6250000013656,104.958734125));
#4437=CARTESIAN_POINT('Ctrl Pts',(-74.2170326445434,13.5625000013656,74.2170326445434));
#4438=CARTESIAN_POINT('Ctrl Pts',(-104.958734125,13.5000000013656,43.4753311640869));
#4439=CARTESIAN_POINT('Ctrl Pts',(-104.958734125,13.4375000013656,0.));
#4440=CARTESIAN_POINT('Ctrl Pts',(-104.958734125,13.3750000013656,-43.4753311640868));
#4441=CARTESIAN_POINT('Ctrl Pts',(-74.2170326445434,13.3125000013656,-74.2170326445434));
#4442=CARTESIAN_POINT('Ctrl Pts',(-43.4753311640868,13.2500000013656,-104.958734125));
#4443=CARTESIAN_POINT('Ctrl Pts',(-6.42686888943697E-15,13.1875000013656,
-104.958734125));
#4444=CARTESIAN_POINT('Ctrl Pts',(43.4753311640868,13.1250000013656,-104.958734125));
#4445=CARTESIAN_POINT('Ctrl Pts',(74.2170326445434,13.0625000013656,-74.2170326445434));
#4446=CARTESIAN_POINT('Ctrl Pts',(104.958734125,13.0000000013656,-43.4753311640868));
#4447=CARTESIAN_POINT('Ctrl Pts',(104.958734125,12.9375000013656,-1.28537377788739E-14));
#4448=CARTESIAN_POINT('Ctrl Pts',(104.958734125,14.1875000013656,-1.28537377788739E-14));
#4449=CARTESIAN_POINT('Ctrl Pts',(104.958734125,14.1250000013656,43.4753311640868));
#4450=CARTESIAN_POINT('Ctrl Pts',(74.2170326445434,14.0625000013656,74.2170326445434));
#4451=CARTESIAN_POINT('Ctrl Pts',(43.4753311640869,14.0000000013656,104.958734125));
#4452=CARTESIAN_POINT('Ctrl Pts',(1.92806066683109E-14,13.9375000013656,
104.958734125));
#4453=CARTESIAN_POINT('Ctrl Pts',(-43.4753311640868,13.8750000013656,104.958734125));
#4454=CARTESIAN_POINT('Ctrl Pts',(-74.2170326445434,13.8125000013656,74.2170326445434));
#4455=CARTESIAN_POINT('Ctrl Pts',(-104.958734125,13.7500000013656,43.4753311640869));
#4456=CARTESIAN_POINT('Ctrl Pts',(-104.958734125,13.6875000013656,0.));
#4457=CARTESIAN_POINT('Ctrl Pts',(-104.958734125,13.6250000013656,-43.4753311640868));
#4458=CARTESIAN_POINT('Ctrl Pts',(-74.2170326445434,13.5625000013656,-74.2170326445434));
#4459=CARTESIAN_POINT('Ctrl Pts',(-43.4753311640868,13.5000000013656,-104.958734125));
#4460=CARTESIAN_POINT('Ctrl Pts',(-6.42686888943697E-15,13.4375000013656,
-104.958734125));
#4461=CARTESIAN_POINT('Ctrl Pts',(43.4753311640868,13.3750000013656,-104.958734125));
#4462=CARTESIAN_POINT('Ctrl Pts',(74.2170326445434,13.3125000013656,-74.2170326445434));
#4463=CARTESIAN_POINT('Ctrl Pts',(104.958734125,13.2500000013656,-43.4753311640868));
#4464=CARTESIAN_POINT('Ctrl Pts',(104.958734125,13.1875000013656,-1.28537377788739E-14));
#4465=CARTESIAN_POINT('Origin',(-7.105427357601E-14,49.5625000013656,-6.0924204042587E-14));
#4466=CARTESIAN_POINT('',(104.958734125,15.1875000013656,-6.0924204042587E-14));
#4467=CARTESIAN_POINT('',(104.958734125,14.9375000013656,-6.0924204042587E-14));
#4468=CARTESIAN_POINT('',(104.958734125,49.5625000013656,-1.089946703063E-13));
#4469=CARTESIAN_POINT('Ctrl Pts',(104.958734125,14.9375000013656,-1.28537377788739E-14));
#4470=CARTESIAN_POINT('Ctrl Pts',(104.958734125,14.8750000013656,43.4753311640868));
#4471=CARTESIAN_POINT('Ctrl Pts',(74.2170326445434,14.8125000013656,74.2170326445434));
#4472=CARTESIAN_POINT('Ctrl Pts',(43.4753311640869,14.7500000013656,104.958734125));
#4473=CARTESIAN_POINT('Ctrl Pts',(1.92806066683109E-14,14.6875000013656,
104.958734125));
#4474=CARTESIAN_POINT('Ctrl Pts',(-43.4753311640868,14.6250000013656,104.958734125));
#4475=CARTESIAN_POINT('Ctrl Pts',(-74.2170326445434,14.5625000013656,74.2170326445434));
#4476=CARTESIAN_POINT('Ctrl Pts',(-104.958734125,14.5000000013656,43.4753311640869));
#4477=CARTESIAN_POINT('Ctrl Pts',(-104.958734125,14.4375000013656,0.));
#4478=CARTESIAN_POINT('Ctrl Pts',(-104.958734125,14.3750000013656,-43.4753311640868));
#4479=CARTESIAN_POINT('Ctrl Pts',(-74.2170326445434,14.3125000013656,-74.2170326445434));
#4480=CARTESIAN_POINT('Ctrl Pts',(-43.4753311640868,14.2500000013656,-104.958734125));
#4481=CARTESIAN_POINT('Ctrl Pts',(-6.42686888943697E-15,14.1875000013656,
-104.958734125));
#4482=CARTESIAN_POINT('Ctrl Pts',(43.4753311640868,14.1250000013656,-104.958734125));
#4483=CARTESIAN_POINT('Ctrl Pts',(74.2170326445434,14.0625000013656,-74.2170326445434));
#4484=CARTESIAN_POINT('Ctrl Pts',(104.958734125,14.0000000013656,-43.4753311640868));
#4485=CARTESIAN_POINT('Ctrl Pts',(104.958734125,13.9375000013656,-1.28537377788739E-14));
#4486=CARTESIAN_POINT('Ctrl Pts',(104.958734125,15.1875000013656,-1.28537377788739E-14));
#4487=CARTESIAN_POINT('Ctrl Pts',(104.958734125,15.1250000013656,43.4753311640868));
#4488=CARTESIAN_POINT('Ctrl Pts',(74.2170326445434,15.0625000013656,74.2170326445434));
#4489=CARTESIAN_POINT('Ctrl Pts',(43.4753311640869,15.0000000013656,104.958734125));
#4490=CARTESIAN_POINT('Ctrl Pts',(1.92806066683109E-14,14.9375000013656,
104.958734125));
#4491=CARTESIAN_POINT('Ctrl Pts',(-43.4753311640868,14.8750000013656,104.958734125));
#4492=CARTESIAN_POINT('Ctrl Pts',(-74.2170326445434,14.8125000013656,74.2170326445434));
#4493=CARTESIAN_POINT('Ctrl Pts',(-104.958734125,14.7500000013656,43.4753311640869));
#4494=CARTESIAN_POINT('Ctrl Pts',(-104.958734125,14.6875000013656,0.));
#4495=CARTESIAN_POINT('Ctrl Pts',(-104.958734125,14.6250000013656,-43.4753311640868));
#4496=CARTESIAN_POINT('Ctrl Pts',(-74.2170326445434,14.5625000013656,-74.2170326445434));
#4497=CARTESIAN_POINT('Ctrl Pts',(-43.4753311640868,14.5000000013656,-104.958734125));
#4498=CARTESIAN_POINT('Ctrl Pts',(-6.42686888943697E-15,14.4375000013656,
-104.958734125));
#4499=CARTESIAN_POINT('Ctrl Pts',(43.4753311640868,14.3750000013656,-104.958734125));
#4500=CARTESIAN_POINT('Ctrl Pts',(74.2170326445434,14.3125000013656,-74.2170326445434));
#4501=CARTESIAN_POINT('Ctrl Pts',(104.958734125,14.2500000013656,-43.4753311640868));
#4502=CARTESIAN_POINT('Ctrl Pts',(104.958734125,14.1875000013656,-1.28537377788739E-14));
#4503=CARTESIAN_POINT('Origin',(-7.105427357601E-14,49.5625000013656,-6.0924204042587E-14));
#4504=CARTESIAN_POINT('',(104.958734125,16.1875000013656,-6.0924204042587E-14));
#4505=CARTESIAN_POINT('',(104.958734125,15.9375000013656,-6.0924204042587E-14));
#4506=CARTESIAN_POINT('',(104.958734125,49.5625000013656,-1.089946703063E-13));
#4507=CARTESIAN_POINT('Ctrl Pts',(104.958734125,15.9375000013656,-1.28537377788739E-14));
#4508=CARTESIAN_POINT('Ctrl Pts',(104.958734125,15.8750000013656,43.4753311640868));
#4509=CARTESIAN_POINT('Ctrl Pts',(74.2170326445434,15.8125000013656,74.2170326445434));
#4510=CARTESIAN_POINT('Ctrl Pts',(43.4753311640869,15.7500000013656,104.958734125));
#4511=CARTESIAN_POINT('Ctrl Pts',(1.92806066683109E-14,15.6875000013656,
104.958734125));
#4512=CARTESIAN_POINT('Ctrl Pts',(-43.4753311640868,15.6250000013656,104.958734125));
#4513=CARTESIAN_POINT('Ctrl Pts',(-74.2170326445434,15.5625000013656,74.2170326445434));
#4514=CARTESIAN_POINT('Ctrl Pts',(-104.958734125,15.5000000013656,43.4753311640869));
#4515=CARTESIAN_POINT('Ctrl Pts',(-104.958734125,15.4375000013656,0.));
#4516=CARTESIAN_POINT('Ctrl Pts',(-104.958734125,15.3750000013656,-43.4753311640868));
#4517=CARTESIAN_POINT('Ctrl Pts',(-74.2170326445434,15.3125000013656,-74.2170326445434));
#4518=CARTESIAN_POINT('Ctrl Pts',(-43.4753311640868,15.2500000013656,-104.958734125));
#4519=CARTESIAN_POINT('Ctrl Pts',(-6.42686888943697E-15,15.1875000013656,
-104.958734125));
#4520=CARTESIAN_POINT('Ctrl Pts',(43.4753311640868,15.1250000013656,-104.958734125));
#4521=CARTESIAN_POINT('Ctrl Pts',(74.2170326445434,15.0625000013656,-74.2170326445434));
#4522=CARTESIAN_POINT('Ctrl Pts',(104.958734125,15.0000000013656,-43.4753311640868));
#4523=CARTESIAN_POINT('Ctrl Pts',(104.958734125,14.9375000013656,-1.28537377788739E-14));
#4524=CARTESIAN_POINT('Ctrl Pts',(104.958734125,16.1875000013656,-1.28537377788739E-14));
#4525=CARTESIAN_POINT('Ctrl Pts',(104.958734125,16.1250000013656,43.4753311640868));
#4526=CARTESIAN_POINT('Ctrl Pts',(74.2170326445434,16.0625000013656,74.2170326445434));
#4527=CARTESIAN_POINT('Ctrl Pts',(43.4753311640869,16.0000000013656,104.958734125));
#4528=CARTESIAN_POINT('Ctrl Pts',(1.92806066683109E-14,15.9375000013656,
104.958734125));
#4529=CARTESIAN_POINT('Ctrl Pts',(-43.4753311640868,15.8750000013656,104.958734125));
#4530=CARTESIAN_POINT('Ctrl Pts',(-74.2170326445434,15.8125000013656,74.2170326445434));
#4531=CARTESIAN_POINT('Ctrl Pts',(-104.958734125,15.7500000013656,43.4753311640869));
#4532=CARTESIAN_POINT('Ctrl Pts',(-104.958734125,15.6875000013656,0.));
#4533=CARTESIAN_POINT('Ctrl Pts',(-104.958734125,15.6250000013656,-43.4753311640868));
#4534=CARTESIAN_POINT('Ctrl Pts',(-74.2170326445434,15.5625000013656,-74.2170326445434));
#4535=CARTESIAN_POINT('Ctrl Pts',(-43.4753311640868,15.5000000013656,-104.958734125));
#4536=CARTESIAN_POINT('Ctrl Pts',(-6.42686888943697E-15,15.4375000013656,
-104.958734125));
#4537=CARTESIAN_POINT('Ctrl Pts',(43.4753311640868,15.3750000013656,-104.958734125));
#4538=CARTESIAN_POINT('Ctrl Pts',(74.2170326445434,15.3125000013656,-74.2170326445434));
#4539=CARTESIAN_POINT('Ctrl Pts',(104.958734125,15.2500000013656,-43.4753311640868));
#4540=CARTESIAN_POINT('Ctrl Pts',(104.958734125,15.1875000013656,-1.28537377788739E-14));
#4541=CARTESIAN_POINT('Origin',(-7.105427357601E-14,49.5625000013656,-6.0924204042587E-14));
#4542=CARTESIAN_POINT('',(104.958734125,17.1875000013656,-6.0924204042587E-14));
#4543=CARTESIAN_POINT('',(104.958734125,16.9375000013656,-6.0924204042587E-14));
#4544=CARTESIAN_POINT('',(104.958734125,49.5625000013656,-1.089946703063E-13));
#4545=CARTESIAN_POINT('Ctrl Pts',(104.958734125,16.9375000013656,-1.28537377788739E-14));
#4546=CARTESIAN_POINT('Ctrl Pts',(104.958734125,16.8750000013656,43.4753311640868));
#4547=CARTESIAN_POINT('Ctrl Pts',(74.2170326445434,16.8125000013656,74.2170326445434));
#4548=CARTESIAN_POINT('Ctrl Pts',(43.4753311640869,16.7500000013656,104.958734125));
#4549=CARTESIAN_POINT('Ctrl Pts',(1.92806066683109E-14,16.6875000013656,
104.958734125));
#4550=CARTESIAN_POINT('Ctrl Pts',(-43.4753311640868,16.6250000013656,104.958734125));
#4551=CARTESIAN_POINT('Ctrl Pts',(-74.2170326445434,16.5625000013656,74.2170326445434));
#4552=CARTESIAN_POINT('Ctrl Pts',(-104.958734125,16.5000000013656,43.4753311640869));
#4553=CARTESIAN_POINT('Ctrl Pts',(-104.958734125,16.4375000013656,0.));
#4554=CARTESIAN_POINT('Ctrl Pts',(-104.958734125,16.3750000013656,-43.4753311640868));
#4555=CARTESIAN_POINT('Ctrl Pts',(-74.2170326445434,16.3125000013656,-74.2170326445434));
#4556=CARTESIAN_POINT('Ctrl Pts',(-43.4753311640868,16.2500000013656,-104.958734125));
#4557=CARTESIAN_POINT('Ctrl Pts',(-6.42686888943697E-15,16.1875000013656,
-104.958734125));
#4558=CARTESIAN_POINT('Ctrl Pts',(43.4753311640868,16.1250000013656,-104.958734125));
#4559=CARTESIAN_POINT('Ctrl Pts',(74.2170326445434,16.0625000013656,-74.2170326445434));
#4560=CARTESIAN_POINT('Ctrl Pts',(104.958734125,16.0000000013656,-43.4753311640868));
#4561=CARTESIAN_POINT('Ctrl Pts',(104.958734125,15.9375000013656,-1.28537377788739E-14));
#4562=CARTESIAN_POINT('Ctrl Pts',(104.958734125,17.1875000013656,-1.28537377788739E-14));
#4563=CARTESIAN_POINT('Ctrl Pts',(104.958734125,17.1250000013656,43.4753311640868));
#4564=CARTESIAN_POINT('Ctrl Pts',(74.2170326445434,17.0625000013656,74.2170326445434));
#4565=CARTESIAN_POINT('Ctrl Pts',(43.4753311640869,17.0000000013656,104.958734125));
#4566=CARTESIAN_POINT('Ctrl Pts',(1.92806066683109E-14,16.9375000013656,
104.958734125));
#4567=CARTESIAN_POINT('Ctrl Pts',(-43.4753311640868,16.8750000013656,104.958734125));
#4568=CARTESIAN_POINT('Ctrl Pts',(-74.2170326445434,16.8125000013656,74.2170326445434));
#4569=CARTESIAN_POINT('Ctrl Pts',(-104.958734125,16.7500000013656,43.4753311640869));
#4570=CARTESIAN_POINT('Ctrl Pts',(-104.958734125,16.6875000013656,0.));
#4571=CARTESIAN_POINT('Ctrl Pts',(-104.958734125,16.6250000013656,-43.4753311640868));
#4572=CARTESIAN_POINT('Ctrl Pts',(-74.2170326445434,16.5625000013656,-74.2170326445434));
#4573=CARTESIAN_POINT('Ctrl Pts',(-43.4753311640868,16.5000000013656,-104.958734125));
#4574=CARTESIAN_POINT('Ctrl Pts',(-6.42686888943697E-15,16.4375000013656,
-104.958734125));
#4575=CARTESIAN_POINT('Ctrl Pts',(43.4753311640868,16.3750000013656,-104.958734125));
#4576=CARTESIAN_POINT('Ctrl Pts',(74.2170326445434,16.3125000013656,-74.2170326445434));
#4577=CARTESIAN_POINT('Ctrl Pts',(104.958734125,16.2500000013656,-43.4753311640868));
#4578=CARTESIAN_POINT('Ctrl Pts',(104.958734125,16.1875000013656,-1.28537377788739E-14));
#4579=CARTESIAN_POINT('Origin',(-7.105427357601E-14,49.5625000013656,-6.0924204042587E-14));
#4580=CARTESIAN_POINT('',(104.958734125,18.1875000013656,-6.0924204042587E-14));
#4581=CARTESIAN_POINT('',(104.958734125,17.9375000013656,-6.0924204042587E-14));
#4582=CARTESIAN_POINT('',(104.958734125,49.5625000013656,-1.089946703063E-13));
#4583=CARTESIAN_POINT('Ctrl Pts',(104.958734125,17.9375000013656,-1.28537377788739E-14));
#4584=CARTESIAN_POINT('Ctrl Pts',(104.958734125,17.8750000013656,43.4753311640868));
#4585=CARTESIAN_POINT('Ctrl Pts',(74.2170326445434,17.8125000013656,74.2170326445434));
#4586=CARTESIAN_POINT('Ctrl Pts',(43.4753311640869,17.7500000013656,104.958734125));
#4587=CARTESIAN_POINT('Ctrl Pts',(1.92806066683109E-14,17.6875000013656,
104.958734125));
#4588=CARTESIAN_POINT('Ctrl Pts',(-43.4753311640868,17.6250000013656,104.958734125));
#4589=CARTESIAN_POINT('Ctrl Pts',(-74.2170326445434,17.5625000013656,74.2170326445434));
#4590=CARTESIAN_POINT('Ctrl Pts',(-104.958734125,17.5000000013656,43.4753311640869));
#4591=CARTESIAN_POINT('Ctrl Pts',(-104.958734125,17.4375000013656,0.));
#4592=CARTESIAN_POINT('Ctrl Pts',(-104.958734125,17.3750000013656,-43.4753311640868));
#4593=CARTESIAN_POINT('Ctrl Pts',(-74.2170326445434,17.3125000013656,-74.2170326445434));
#4594=CARTESIAN_POINT('Ctrl Pts',(-43.4753311640868,17.2500000013656,-104.958734125));
#4595=CARTESIAN_POINT('Ctrl Pts',(-6.42686888943697E-15,17.1875000013656,
-104.958734125));
#4596=CARTESIAN_POINT('Ctrl Pts',(43.4753311640868,17.1250000013656,-104.958734125));
#4597=CARTESIAN_POINT('Ctrl Pts',(74.2170326445434,17.0625000013656,-74.2170326445434));
#4598=CARTESIAN_POINT('Ctrl Pts',(104.958734125,17.0000000013656,-43.4753311640868));
#4599=CARTESIAN_POINT('Ctrl Pts',(104.958734125,16.9375000013656,-1.28537377788739E-14));
#4600=CARTESIAN_POINT('Ctrl Pts',(104.958734125,18.1875000013656,-1.28537377788739E-14));
#4601=CARTESIAN_POINT('Ctrl Pts',(104.958734125,18.1250000013656,43.4753311640868));
#4602=CARTESIAN_POINT('Ctrl Pts',(74.2170326445434,18.0625000013656,74.2170326445434));
#4603=CARTESIAN_POINT('Ctrl Pts',(43.4753311640869,18.0000000013656,104.958734125));
#4604=CARTESIAN_POINT('Ctrl Pts',(1.92806066683109E-14,17.9375000013656,
104.958734125));
#4605=CARTESIAN_POINT('Ctrl Pts',(-43.4753311640868,17.8750000013656,104.958734125));
#4606=CARTESIAN_POINT('Ctrl Pts',(-74.2170326445434,17.8125000013656,74.2170326445434));
#4607=CARTESIAN_POINT('Ctrl Pts',(-104.958734125,17.7500000013656,43.4753311640869));
#4608=CARTESIAN_POINT('Ctrl Pts',(-104.958734125,17.6875000013656,0.));
#4609=CARTESIAN_POINT('Ctrl Pts',(-104.958734125,17.6250000013656,-43.4753311640868));
#4610=CARTESIAN_POINT('Ctrl Pts',(-74.2170326445434,17.5625000013656,-74.2170326445434));
#4611=CARTESIAN_POINT('Ctrl Pts',(-43.4753311640868,17.5000000013656,-104.958734125));
#4612=CARTESIAN_POINT('Ctrl Pts',(-6.42686888943697E-15,17.4375000013656,
-104.958734125));
#4613=CARTESIAN_POINT('Ctrl Pts',(43.4753311640868,17.3750000013656,-104.958734125));
#4614=CARTESIAN_POINT('Ctrl Pts',(74.2170326445434,17.3125000013656,-74.2170326445434));
#4615=CARTESIAN_POINT('Ctrl Pts',(104.958734125,17.2500000013656,-43.4753311640868));
#4616=CARTESIAN_POINT('Ctrl Pts',(104.958734125,17.1875000013656,-1.28537377788739E-14));
#4617=CARTESIAN_POINT('Origin',(-7.105427357601E-14,49.5625000013656,-6.0924204042587E-14));
#4618=CARTESIAN_POINT('',(104.958734125,19.1875000013656,-6.0924204042587E-14));
#4619=CARTESIAN_POINT('',(104.958734125,18.9375000013656,-6.0924204042587E-14));
#4620=CARTESIAN_POINT('',(104.958734125,49.5625000013656,-1.089946703063E-13));
#4621=CARTESIAN_POINT('Ctrl Pts',(104.958734125,18.9375000013656,-1.28537377788739E-14));
#4622=CARTESIAN_POINT('Ctrl Pts',(104.958734125,18.8750000013656,43.4753311640868));
#4623=CARTESIAN_POINT('Ctrl Pts',(74.2170326445434,18.8125000013656,74.2170326445434));
#4624=CARTESIAN_POINT('Ctrl Pts',(43.4753311640869,18.7500000013656,104.958734125));
#4625=CARTESIAN_POINT('Ctrl Pts',(1.92806066683109E-14,18.6875000013656,
104.958734125));
#4626=CARTESIAN_POINT('Ctrl Pts',(-43.4753311640868,18.6250000013656,104.958734125));
#4627=CARTESIAN_POINT('Ctrl Pts',(-74.2170326445434,18.5625000013656,74.2170326445434));
#4628=CARTESIAN_POINT('Ctrl Pts',(-104.958734125,18.5000000013656,43.4753311640869));
#4629=CARTESIAN_POINT('Ctrl Pts',(-104.958734125,18.4375000013656,0.));
#4630=CARTESIAN_POINT('Ctrl Pts',(-104.958734125,18.3750000013656,-43.4753311640868));
#4631=CARTESIAN_POINT('Ctrl Pts',(-74.2170326445434,18.3125000013656,-74.2170326445434));
#4632=CARTESIAN_POINT('Ctrl Pts',(-43.4753311640868,18.2500000013656,-104.958734125));
#4633=CARTESIAN_POINT('Ctrl Pts',(-6.42686888943697E-15,18.1875000013656,
-104.958734125));
#4634=CARTESIAN_POINT('Ctrl Pts',(43.4753311640868,18.1250000013656,-104.958734125));
#4635=CARTESIAN_POINT('Ctrl Pts',(74.2170326445434,18.0625000013656,-74.2170326445434));
#4636=CARTESIAN_POINT('Ctrl Pts',(104.958734125,18.0000000013656,-43.4753311640868));
#4637=CARTESIAN_POINT('Ctrl Pts',(104.958734125,17.9375000013656,-1.28537377788739E-14));
#4638=CARTESIAN_POINT('Ctrl Pts',(104.958734125,19.1875000013656,-1.28537377788739E-14));
#4639=CARTESIAN_POINT('Ctrl Pts',(104.958734125,19.1250000013656,43.4753311640868));
#4640=CARTESIAN_POINT('Ctrl Pts',(74.2170326445434,19.0625000013656,74.2170326445434));
#4641=CARTESIAN_POINT('Ctrl Pts',(43.4753311640869,19.0000000013656,104.958734125));
#4642=CARTESIAN_POINT('Ctrl Pts',(1.92806066683109E-14,18.9375000013656,
104.958734125));
#4643=CARTESIAN_POINT('Ctrl Pts',(-43.4753311640868,18.8750000013656,104.958734125));
#4644=CARTESIAN_POINT('Ctrl Pts',(-74.2170326445434,18.8125000013656,74.2170326445434));
#4645=CARTESIAN_POINT('Ctrl Pts',(-104.958734125,18.7500000013656,43.4753311640869));
#4646=CARTESIAN_POINT('Ctrl Pts',(-104.958734125,18.6875000013656,0.));
#4647=CARTESIAN_POINT('Ctrl Pts',(-104.958734125,18.6250000013656,-43.4753311640868));
#4648=CARTESIAN_POINT('Ctrl Pts',(-74.2170326445434,18.5625000013656,-74.2170326445434));
#4649=CARTESIAN_POINT('Ctrl Pts',(-43.4753311640868,18.5000000013656,-104.958734125));
#4650=CARTESIAN_POINT('Ctrl Pts',(-6.42686888943697E-15,18.4375000013656,
-104.958734125));
#4651=CARTESIAN_POINT('Ctrl Pts',(43.4753311640868,18.3750000013656,-104.958734125));
#4652=CARTESIAN_POINT('Ctrl Pts',(74.2170326445434,18.3125000013656,-74.2170326445434));
#4653=CARTESIAN_POINT('Ctrl Pts',(104.958734125,18.2500000013656,-43.4753311640868));
#4654=CARTESIAN_POINT('Ctrl Pts',(104.958734125,18.1875000013656,-1.28537377788739E-14));
#4655=CARTESIAN_POINT('Origin',(-7.105427357601E-14,49.5625000013656,-6.0924204042587E-14));
#4656=CARTESIAN_POINT('',(104.958734125,20.1875000013656,-6.0924204042587E-14));
#4657=CARTESIAN_POINT('',(104.958734125,19.9375000013656,-6.0924204042587E-14));
#4658=CARTESIAN_POINT('',(104.958734125,49.5625000013656,-1.089946703063E-13));
#4659=CARTESIAN_POINT('Ctrl Pts',(104.958734125,19.9375000013656,-1.28537377788739E-14));
#4660=CARTESIAN_POINT('Ctrl Pts',(104.958734125,19.8750000013656,43.4753311640868));
#4661=CARTESIAN_POINT('Ctrl Pts',(74.2170326445434,19.8125000013656,74.2170326445434));
#4662=CARTESIAN_POINT('Ctrl Pts',(43.4753311640869,19.7500000013656,104.958734125));
#4663=CARTESIAN_POINT('Ctrl Pts',(1.92806066683109E-14,19.6875000013656,
104.958734125));
#4664=CARTESIAN_POINT('Ctrl Pts',(-43.4753311640868,19.6250000013656,104.958734125));
#4665=CARTESIAN_POINT('Ctrl Pts',(-74.2170326445434,19.5625000013656,74.2170326445434));
#4666=CARTESIAN_POINT('Ctrl Pts',(-104.958734125,19.5000000013656,43.4753311640869));
#4667=CARTESIAN_POINT('Ctrl Pts',(-104.958734125,19.4375000013656,0.));
#4668=CARTESIAN_POINT('Ctrl Pts',(-104.958734125,19.3750000013656,-43.4753311640868));
#4669=CARTESIAN_POINT('Ctrl Pts',(-74.2170326445434,19.3125000013656,-74.2170326445434));
#4670=CARTESIAN_POINT('Ctrl Pts',(-43.4753311640868,19.2500000013656,-104.958734125));
#4671=CARTESIAN_POINT('Ctrl Pts',(-6.42686888943697E-15,19.1875000013656,
-104.958734125));
#4672=CARTESIAN_POINT('Ctrl Pts',(43.4753311640868,19.1250000013656,-104.958734125));
#4673=CARTESIAN_POINT('Ctrl Pts',(74.2170326445434,19.0625000013656,-74.2170326445434));
#4674=CARTESIAN_POINT('Ctrl Pts',(104.958734125,19.0000000013656,-43.4753311640868));
#4675=CARTESIAN_POINT('Ctrl Pts',(104.958734125,18.9375000013656,-1.28537377788739E-14));
#4676=CARTESIAN_POINT('Ctrl Pts',(104.958734125,20.1875000013656,-1.28537377788739E-14));
#4677=CARTESIAN_POINT('Ctrl Pts',(104.958734125,20.1250000013656,43.4753311640868));
#4678=CARTESIAN_POINT('Ctrl Pts',(74.2170326445434,20.0625000013656,74.2170326445434));
#4679=CARTESIAN_POINT('Ctrl Pts',(43.4753311640869,20.0000000013656,104.958734125));
#4680=CARTESIAN_POINT('Ctrl Pts',(1.92806066683109E-14,19.9375000013656,
104.958734125));
#4681=CARTESIAN_POINT('Ctrl Pts',(-43.4753311640868,19.8750000013656,104.958734125));
#4682=CARTESIAN_POINT('Ctrl Pts',(-74.2170326445434,19.8125000013656,74.2170326445434));
#4683=CARTESIAN_POINT('Ctrl Pts',(-104.958734125,19.7500000013656,43.4753311640869));
#4684=CARTESIAN_POINT('Ctrl Pts',(-104.958734125,19.6875000013656,0.));
#4685=CARTESIAN_POINT('Ctrl Pts',(-104.958734125,19.6250000013656,-43.4753311640868));
#4686=CARTESIAN_POINT('Ctrl Pts',(-74.2170326445434,19.5625000013656,-74.2170326445434));
#4687=CARTESIAN_POINT('Ctrl Pts',(-43.4753311640868,19.5000000013656,-104.958734125));
#4688=CARTESIAN_POINT('Ctrl Pts',(-6.42686888943697E-15,19.4375000013656,
-104.958734125));
#4689=CARTESIAN_POINT('Ctrl Pts',(43.4753311640868,19.3750000013656,-104.958734125));
#4690=CARTESIAN_POINT('Ctrl Pts',(74.2170326445434,19.3125000013656,-74.2170326445434));
#4691=CARTESIAN_POINT('Ctrl Pts',(104.958734125,19.2500000013656,-43.4753311640868));
#4692=CARTESIAN_POINT('Ctrl Pts',(104.958734125,19.1875000013656,-1.28537377788739E-14));
#4693=CARTESIAN_POINT('Origin',(-7.105427357601E-14,49.5625000013656,-6.0924204042587E-14));
#4694=CARTESIAN_POINT('',(104.958734125,21.1875000013656,-6.0924204042587E-14));
#4695=CARTESIAN_POINT('',(104.958734125,20.9375000013656,-6.0924204042587E-14));
#4696=CARTESIAN_POINT('',(104.958734125,49.5625000013656,-1.089946703063E-13));
#4697=CARTESIAN_POINT('Ctrl Pts',(104.958734125,20.9375000013656,-1.28537377788739E-14));
#4698=CARTESIAN_POINT('Ctrl Pts',(104.958734125,20.8750000013656,43.4753311640868));
#4699=CARTESIAN_POINT('Ctrl Pts',(74.2170326445434,20.8125000013656,74.2170326445434));
#4700=CARTESIAN_POINT('Ctrl Pts',(43.4753311640869,20.7500000013656,104.958734125));
#4701=CARTESIAN_POINT('Ctrl Pts',(1.92806066683109E-14,20.6875000013656,
104.958734125));
#4702=CARTESIAN_POINT('Ctrl Pts',(-43.4753311640868,20.6250000013656,104.958734125));
#4703=CARTESIAN_POINT('Ctrl Pts',(-74.2170326445434,20.5625000013656,74.2170326445434));
#4704=CARTESIAN_POINT('Ctrl Pts',(-104.958734125,20.5000000013656,43.4753311640869));
#4705=CARTESIAN_POINT('Ctrl Pts',(-104.958734125,20.4375000013656,0.));
#4706=CARTESIAN_POINT('Ctrl Pts',(-104.958734125,20.3750000013656,-43.4753311640868));
#4707=CARTESIAN_POINT('Ctrl Pts',(-74.2170326445434,20.3125000013656,-74.2170326445434));
#4708=CARTESIAN_POINT('Ctrl Pts',(-43.4753311640868,20.2500000013656,-104.958734125));
#4709=CARTESIAN_POINT('Ctrl Pts',(-6.42686888943697E-15,20.1875000013656,
-104.958734125));
#4710=CARTESIAN_POINT('Ctrl Pts',(43.4753311640868,20.1250000013656,-104.958734125));
#4711=CARTESIAN_POINT('Ctrl Pts',(74.2170326445434,20.0625000013656,-74.2170326445434));
#4712=CARTESIAN_POINT('Ctrl Pts',(104.958734125,20.0000000013656,-43.4753311640868));
#4713=CARTESIAN_POINT('Ctrl Pts',(104.958734125,19.9375000013656,-1.28537377788739E-14));
#4714=CARTESIAN_POINT('Ctrl Pts',(104.958734125,21.1875000013656,-1.28537377788739E-14));
#4715=CARTESIAN_POINT('Ctrl Pts',(104.958734125,21.1250000013656,43.4753311640868));
#4716=CARTESIAN_POINT('Ctrl Pts',(74.2170326445434,21.0625000013656,74.2170326445434));
#4717=CARTESIAN_POINT('Ctrl Pts',(43.4753311640869,21.0000000013656,104.958734125));
#4718=CARTESIAN_POINT('Ctrl Pts',(1.92806066683109E-14,20.9375000013656,
104.958734125));
#4719=CARTESIAN_POINT('Ctrl Pts',(-43.4753311640868,20.8750000013656,104.958734125));
#4720=CARTESIAN_POINT('Ctrl Pts',(-74.2170326445434,20.8125000013656,74.2170326445434));
#4721=CARTESIAN_POINT('Ctrl Pts',(-104.958734125,20.7500000013656,43.4753311640869));
#4722=CARTESIAN_POINT('Ctrl Pts',(-104.958734125,20.6875000013656,0.));
#4723=CARTESIAN_POINT('Ctrl Pts',(-104.958734125,20.6250000013656,-43.4753311640868));
#4724=CARTESIAN_POINT('Ctrl Pts',(-74.2170326445434,20.5625000013656,-74.2170326445434));
#4725=CARTESIAN_POINT('Ctrl Pts',(-43.4753311640868,20.5000000013656,-104.958734125));
#4726=CARTESIAN_POINT('Ctrl Pts',(-6.42686888943697E-15,20.4375000013656,
-104.958734125));
#4727=CARTESIAN_POINT('Ctrl Pts',(43.4753311640868,20.3750000013656,-104.958734125));
#4728=CARTESIAN_POINT('Ctrl Pts',(74.2170326445434,20.3125000013656,-74.2170326445434));
#4729=CARTESIAN_POINT('Ctrl Pts',(104.958734125,20.2500000013656,-43.4753311640868));
#4730=CARTESIAN_POINT('Ctrl Pts',(104.958734125,20.1875000013656,-1.28537377788739E-14));
#4731=CARTESIAN_POINT('Origin',(-7.105427357601E-14,49.5625000013656,-6.0924204042587E-14));
#4732=CARTESIAN_POINT('',(104.958734125,22.1875000013656,-6.0924204042587E-14));
#4733=CARTESIAN_POINT('',(104.958734125,21.9375000013656,-6.0924204042587E-14));
#4734=CARTESIAN_POINT('',(104.958734125,49.5625000013656,-1.089946703063E-13));
#4735=CARTESIAN_POINT('Ctrl Pts',(104.958734125,21.9375000013656,-1.28537377788739E-14));
#4736=CARTESIAN_POINT('Ctrl Pts',(104.958734125,21.8750000013656,43.4753311640868));
#4737=CARTESIAN_POINT('Ctrl Pts',(74.2170326445434,21.8125000013656,74.2170326445434));
#4738=CARTESIAN_POINT('Ctrl Pts',(43.4753311640869,21.7500000013656,104.958734125));
#4739=CARTESIAN_POINT('Ctrl Pts',(1.92806066683109E-14,21.6875000013656,
104.958734125));
#4740=CARTESIAN_POINT('Ctrl Pts',(-43.4753311640868,21.6250000013656,104.958734125));
#4741=CARTESIAN_POINT('Ctrl Pts',(-74.2170326445434,21.5625000013656,74.2170326445434));
#4742=CARTESIAN_POINT('Ctrl Pts',(-104.958734125,21.5000000013656,43.4753311640869));
#4743=CARTESIAN_POINT('Ctrl Pts',(-104.958734125,21.4375000013656,0.));
#4744=CARTESIAN_POINT('Ctrl Pts',(-104.958734125,21.3750000013656,-43.4753311640868));
#4745=CARTESIAN_POINT('Ctrl Pts',(-74.2170326445434,21.3125000013656,-74.2170326445434));
#4746=CARTESIAN_POINT('Ctrl Pts',(-43.4753311640868,21.2500000013656,-104.958734125));
#4747=CARTESIAN_POINT('Ctrl Pts',(-6.42686888943697E-15,21.1875000013656,
-104.958734125));
#4748=CARTESIAN_POINT('Ctrl Pts',(43.4753311640868,21.1250000013656,-104.958734125));
#4749=CARTESIAN_POINT('Ctrl Pts',(74.2170326445434,21.0625000013656,-74.2170326445434));
#4750=CARTESIAN_POINT('Ctrl Pts',(104.958734125,21.0000000013656,-43.4753311640868));
#4751=CARTESIAN_POINT('Ctrl Pts',(104.958734125,20.9375000013656,-1.28537377788739E-14));
#4752=CARTESIAN_POINT('Ctrl Pts',(104.958734125,22.1875000013656,-1.28537377788739E-14));
#4753=CARTESIAN_POINT('Ctrl Pts',(104.958734125,22.1250000013656,43.4753311640868));
#4754=CARTESIAN_POINT('Ctrl Pts',(74.2170326445434,22.0625000013656,74.2170326445434));
#4755=CARTESIAN_POINT('Ctrl Pts',(43.4753311640869,22.0000000013656,104.958734125));
#4756=CARTESIAN_POINT('Ctrl Pts',(1.92806066683109E-14,21.9375000013656,
104.958734125));
#4757=CARTESIAN_POINT('Ctrl Pts',(-43.4753311640868,21.8750000013656,104.958734125));
#4758=CARTESIAN_POINT('Ctrl Pts',(-74.2170326445434,21.8125000013656,74.2170326445434));
#4759=CARTESIAN_POINT('Ctrl Pts',(-104.958734125,21.7500000013656,43.4753311640869));
#4760=CARTESIAN_POINT('Ctrl Pts',(-104.958734125,21.6875000013656,0.));
#4761=CARTESIAN_POINT('Ctrl Pts',(-104.958734125,21.6250000013656,-43.4753311640868));
#4762=CARTESIAN_POINT('Ctrl Pts',(-74.2170326445434,21.5625000013656,-74.2170326445434));
#4763=CARTESIAN_POINT('Ctrl Pts',(-43.4753311640868,21.5000000013656,-104.958734125));
#4764=CARTESIAN_POINT('Ctrl Pts',(-6.42686888943697E-15,21.4375000013656,
-104.958734125));
#4765=CARTESIAN_POINT('Ctrl Pts',(43.4753311640868,21.3750000013656,-104.958734125));
#4766=CARTESIAN_POINT('Ctrl Pts',(74.2170326445434,21.3125000013656,-74.2170326445434));
#4767=CARTESIAN_POINT('Ctrl Pts',(104.958734125,21.2500000013656,-43.4753311640868));
#4768=CARTESIAN_POINT('Ctrl Pts',(104.958734125,21.1875000013656,-1.28537377788739E-14));
#4769=CARTESIAN_POINT('Origin',(-7.105427357601E-14,49.5625000013656,-6.0924204042587E-14));
#4770=CARTESIAN_POINT('',(104.958734125,23.1875000013656,-6.0924204042587E-14));
#4771=CARTESIAN_POINT('',(104.958734125,22.9375000013656,-6.0924204042587E-14));
#4772=CARTESIAN_POINT('',(104.958734125,49.5625000013656,-1.089946703063E-13));
#4773=CARTESIAN_POINT('Ctrl Pts',(104.958734125,22.9375000013656,-1.28537377788739E-14));
#4774=CARTESIAN_POINT('Ctrl Pts',(104.958734125,22.8750000013656,43.4753311640868));
#4775=CARTESIAN_POINT('Ctrl Pts',(74.2170326445434,22.8125000013656,74.2170326445434));
#4776=CARTESIAN_POINT('Ctrl Pts',(43.4753311640869,22.7500000013656,104.958734125));
#4777=CARTESIAN_POINT('Ctrl Pts',(1.92806066683109E-14,22.6875000013656,
104.958734125));
#4778=CARTESIAN_POINT('Ctrl Pts',(-43.4753311640868,22.6250000013656,104.958734125));
#4779=CARTESIAN_POINT('Ctrl Pts',(-74.2170326445434,22.5625000013656,74.2170326445434));
#4780=CARTESIAN_POINT('Ctrl Pts',(-104.958734125,22.5000000013656,43.4753311640869));
#4781=CARTESIAN_POINT('Ctrl Pts',(-104.958734125,22.4375000013656,0.));
#4782=CARTESIAN_POINT('Ctrl Pts',(-104.958734125,22.3750000013656,-43.4753311640868));
#4783=CARTESIAN_POINT('Ctrl Pts',(-74.2170326445434,22.3125000013656,-74.2170326445434));
#4784=CARTESIAN_POINT('Ctrl Pts',(-43.4753311640868,22.2500000013656,-104.958734125));
#4785=CARTESIAN_POINT('Ctrl Pts',(-6.42686888943697E-15,22.1875000013656,
-104.958734125));
#4786=CARTESIAN_POINT('Ctrl Pts',(43.4753311640868,22.1250000013656,-104.958734125));
#4787=CARTESIAN_POINT('Ctrl Pts',(74.2170326445434,22.0625000013656,-74.2170326445434));
#4788=CARTESIAN_POINT('Ctrl Pts',(104.958734125,22.0000000013656,-43.4753311640868));
#4789=CARTESIAN_POINT('Ctrl Pts',(104.958734125,21.9375000013656,-1.28537377788739E-14));
#4790=CARTESIAN_POINT('Ctrl Pts',(104.958734125,23.1875000013656,-1.28537377788739E-14));
#4791=CARTESIAN_POINT('Ctrl Pts',(104.958734125,23.1250000013656,43.4753311640868));
#4792=CARTESIAN_POINT('Ctrl Pts',(74.2170326445434,23.0625000013656,74.2170326445434));
#4793=CARTESIAN_POINT('Ctrl Pts',(43.4753311640869,23.0000000013656,104.958734125));
#4794=CARTESIAN_POINT('Ctrl Pts',(1.92806066683109E-14,22.9375000013656,
104.958734125));
#4795=CARTESIAN_POINT('Ctrl Pts',(-43.4753311640868,22.8750000013656,104.958734125));
#4796=CARTESIAN_POINT('Ctrl Pts',(-74.2170326445434,22.8125000013656,74.2170326445434));
#4797=CARTESIAN_POINT('Ctrl Pts',(-104.958734125,22.7500000013656,43.4753311640869));
#4798=CARTESIAN_POINT('Ctrl Pts',(-104.958734125,22.6875000013656,0.));
#4799=CARTESIAN_POINT('Ctrl Pts',(-104.958734125,22.6250000013656,-43.4753311640868));
#4800=CARTESIAN_POINT('Ctrl Pts',(-74.2170326445434,22.5625000013656,-74.2170326445434));
#4801=CARTESIAN_POINT('Ctrl Pts',(-43.4753311640868,22.5000000013656,-104.958734125));
#4802=CARTESIAN_POINT('Ctrl Pts',(-6.42686888943697E-15,22.4375000013656,
-104.958734125));
#4803=CARTESIAN_POINT('Ctrl Pts',(43.4753311640868,22.3750000013656,-104.958734125));
#4804=CARTESIAN_POINT('Ctrl Pts',(74.2170326445434,22.3125000013656,-74.2170326445434));
#4805=CARTESIAN_POINT('Ctrl Pts',(104.958734125,22.2500000013656,-43.4753311640868));
#4806=CARTESIAN_POINT('Ctrl Pts',(104.958734125,22.1875000013656,-1.28537377788739E-14));
#4807=CARTESIAN_POINT('Origin',(-7.105427357601E-14,49.5625000013656,-6.0924204042587E-14));
#4808=CARTESIAN_POINT('',(104.958734125,24.1875000013656,-6.0924204042587E-14));
#4809=CARTESIAN_POINT('',(104.958734125,23.9375000013656,-6.0924204042587E-14));
#4810=CARTESIAN_POINT('',(104.958734125,49.5625000013656,-1.089946703063E-13));
#4811=CARTESIAN_POINT('Ctrl Pts',(104.958734125,23.9375000013656,-1.28537377788739E-14));
#4812=CARTESIAN_POINT('Ctrl Pts',(104.958734125,23.8750000013656,43.4753311640868));
#4813=CARTESIAN_POINT('Ctrl Pts',(74.2170326445434,23.8125000013656,74.2170326445434));
#4814=CARTESIAN_POINT('Ctrl Pts',(43.4753311640869,23.7500000013656,104.958734125));
#4815=CARTESIAN_POINT('Ctrl Pts',(1.92806066683109E-14,23.6875000013656,
104.958734125));
#4816=CARTESIAN_POINT('Ctrl Pts',(-43.4753311640868,23.6250000013656,104.958734125));
#4817=CARTESIAN_POINT('Ctrl Pts',(-74.2170326445434,23.5625000013656,74.2170326445434));
#4818=CARTESIAN_POINT('Ctrl Pts',(-104.958734125,23.5000000013656,43.4753311640869));
#4819=CARTESIAN_POINT('Ctrl Pts',(-104.958734125,23.4375000013656,0.));
#4820=CARTESIAN_POINT('Ctrl Pts',(-104.958734125,23.3750000013656,-43.4753311640868));
#4821=CARTESIAN_POINT('Ctrl Pts',(-74.2170326445434,23.3125000013656,-74.2170326445434));
#4822=CARTESIAN_POINT('Ctrl Pts',(-43.4753311640868,23.2500000013656,-104.958734125));
#4823=CARTESIAN_POINT('Ctrl Pts',(-6.42686888943697E-15,23.1875000013656,
-104.958734125));
#4824=CARTESIAN_POINT('Ctrl Pts',(43.4753311640868,23.1250000013656,-104.958734125));
#4825=CARTESIAN_POINT('Ctrl Pts',(74.2170326445434,23.0625000013656,-74.2170326445434));
#4826=CARTESIAN_POINT('Ctrl Pts',(104.958734125,23.0000000013656,-43.4753311640868));
#4827=CARTESIAN_POINT('Ctrl Pts',(104.958734125,22.9375000013656,-1.28537377788739E-14));
#4828=CARTESIAN_POINT('Ctrl Pts',(104.958734125,24.1875000013656,-1.28537377788739E-14));
#4829=CARTESIAN_POINT('Ctrl Pts',(104.958734125,24.1250000013656,43.4753311640868));
#4830=CARTESIAN_POINT('Ctrl Pts',(74.2170326445434,24.0625000013656,74.2170326445434));
#4831=CARTESIAN_POINT('Ctrl Pts',(43.4753311640869,24.0000000013656,104.958734125));
#4832=CARTESIAN_POINT('Ctrl Pts',(1.92806066683109E-14,23.9375000013656,
104.958734125));
#4833=CARTESIAN_POINT('Ctrl Pts',(-43.4753311640868,23.8750000013656,104.958734125));
#4834=CARTESIAN_POINT('Ctrl Pts',(-74.2170326445434,23.8125000013656,74.2170326445434));
#4835=CARTESIAN_POINT('Ctrl Pts',(-104.958734125,23.7500000013656,43.4753311640869));
#4836=CARTESIAN_POINT('Ctrl Pts',(-104.958734125,23.6875000013656,0.));
#4837=CARTESIAN_POINT('Ctrl Pts',(-104.958734125,23.6250000013656,-43.4753311640868));
#4838=CARTESIAN_POINT('Ctrl Pts',(-74.2170326445434,23.5625000013656,-74.2170326445434));
#4839=CARTESIAN_POINT('Ctrl Pts',(-43.4753311640868,23.5000000013656,-104.958734125));
#4840=CARTESIAN_POINT('Ctrl Pts',(-6.42686888943697E-15,23.4375000013656,
-104.958734125));
#4841=CARTESIAN_POINT('Ctrl Pts',(43.4753311640868,23.3750000013656,-104.958734125));
#4842=CARTESIAN_POINT('Ctrl Pts',(74.2170326445434,23.3125000013656,-74.2170326445434));
#4843=CARTESIAN_POINT('Ctrl Pts',(104.958734125,23.2500000013656,-43.4753311640868));
#4844=CARTESIAN_POINT('Ctrl Pts',(104.958734125,23.1875000013656,-1.28537377788739E-14));
#4845=CARTESIAN_POINT('Origin',(-7.105427357601E-14,49.5625000013656,-6.0924204042587E-14));
#4846=CARTESIAN_POINT('',(104.958734125,25.1875000013656,-6.0924204042587E-14));
#4847=CARTESIAN_POINT('',(104.958734125,24.9375000013656,-6.0924204042587E-14));
#4848=CARTESIAN_POINT('',(104.958734125,49.5625000013656,-1.089946703063E-13));
#4849=CARTESIAN_POINT('Ctrl Pts',(104.958734125,24.9375000013656,-1.28537377788739E-14));
#4850=CARTESIAN_POINT('Ctrl Pts',(104.958734125,24.8750000013656,43.4753311640868));
#4851=CARTESIAN_POINT('Ctrl Pts',(74.2170326445434,24.8125000013656,74.2170326445434));
#4852=CARTESIAN_POINT('Ctrl Pts',(43.4753311640869,24.7500000013656,104.958734125));
#4853=CARTESIAN_POINT('Ctrl Pts',(1.92806066683109E-14,24.6875000013656,
104.958734125));
#4854=CARTESIAN_POINT('Ctrl Pts',(-43.4753311640868,24.6250000013656,104.958734125));
#4855=CARTESIAN_POINT('Ctrl Pts',(-74.2170326445434,24.5625000013656,74.2170326445434));
#4856=CARTESIAN_POINT('Ctrl Pts',(-104.958734125,24.5000000013656,43.4753311640869));
#4857=CARTESIAN_POINT('Ctrl Pts',(-104.958734125,24.4375000013656,0.));
#4858=CARTESIAN_POINT('Ctrl Pts',(-104.958734125,24.3750000013656,-43.4753311640868));
#4859=CARTESIAN_POINT('Ctrl Pts',(-74.2170326445434,24.3125000013656,-74.2170326445434));
#4860=CARTESIAN_POINT('Ctrl Pts',(-43.4753311640868,24.2500000013656,-104.958734125));
#4861=CARTESIAN_POINT('Ctrl Pts',(-6.42686888943697E-15,24.1875000013656,
-104.958734125));
#4862=CARTESIAN_POINT('Ctrl Pts',(43.4753311640868,24.1250000013656,-104.958734125));
#4863=CARTESIAN_POINT('Ctrl Pts',(74.2170326445434,24.0625000013656,-74.2170326445434));
#4864=CARTESIAN_POINT('Ctrl Pts',(104.958734125,24.0000000013656,-43.4753311640868));
#4865=CARTESIAN_POINT('Ctrl Pts',(104.958734125,23.9375000013656,-1.28537377788739E-14));
#4866=CARTESIAN_POINT('Ctrl Pts',(104.958734125,25.1875000013656,-1.28537377788739E-14));
#4867=CARTESIAN_POINT('Ctrl Pts',(104.958734125,25.1250000013656,43.4753311640868));
#4868=CARTESIAN_POINT('Ctrl Pts',(74.2170326445434,25.0625000013656,74.2170326445434));
#4869=CARTESIAN_POINT('Ctrl Pts',(43.4753311640869,25.0000000013656,104.958734125));
#4870=CARTESIAN_POINT('Ctrl Pts',(1.92806066683109E-14,24.9375000013656,
104.958734125));
#4871=CARTESIAN_POINT('Ctrl Pts',(-43.4753311640868,24.8750000013656,104.958734125));
#4872=CARTESIAN_POINT('Ctrl Pts',(-74.2170326445434,24.8125000013656,74.2170326445434));
#4873=CARTESIAN_POINT('Ctrl Pts',(-104.958734125,24.7500000013656,43.4753311640869));
#4874=CARTESIAN_POINT('Ctrl Pts',(-104.958734125,24.6875000013656,0.));
#4875=CARTESIAN_POINT('Ctrl Pts',(-104.958734125,24.6250000013656,-43.4753311640868));
#4876=CARTESIAN_POINT('Ctrl Pts',(-74.2170326445434,24.5625000013656,-74.2170326445434));
#4877=CARTESIAN_POINT('Ctrl Pts',(-43.4753311640868,24.5000000013656,-104.958734125));
#4878=CARTESIAN_POINT('Ctrl Pts',(-6.42686888943697E-15,24.4375000013656,
-104.958734125));
#4879=CARTESIAN_POINT('Ctrl Pts',(43.4753311640868,24.3750000013656,-104.958734125));
#4880=CARTESIAN_POINT('Ctrl Pts',(74.2170326445434,24.3125000013656,-74.2170326445434));
#4881=CARTESIAN_POINT('Ctrl Pts',(104.958734125,24.2500000013656,-43.4753311640868));
#4882=CARTESIAN_POINT('Ctrl Pts',(104.958734125,24.1875000013656,-1.28537377788739E-14));
#4883=CARTESIAN_POINT('Origin',(-7.105427357601E-14,49.5625000013656,-6.0924204042587E-14));
#4884=CARTESIAN_POINT('',(104.958734125,26.1875000013656,-6.0924204042587E-14));
#4885=CARTESIAN_POINT('',(104.958734125,25.9375000013656,-6.0924204042587E-14));
#4886=CARTESIAN_POINT('',(104.958734125,49.5625000013656,-1.089946703063E-13));
#4887=CARTESIAN_POINT('Ctrl Pts',(104.958734125,25.9375000013656,-1.28537377788739E-14));
#4888=CARTESIAN_POINT('Ctrl Pts',(104.958734125,25.8750000013656,43.4753311640868));
#4889=CARTESIAN_POINT('Ctrl Pts',(74.2170326445434,25.8125000013656,74.2170326445434));
#4890=CARTESIAN_POINT('Ctrl Pts',(43.4753311640869,25.7500000013656,104.958734125));
#4891=CARTESIAN_POINT('Ctrl Pts',(1.92806066683109E-14,25.6875000013656,
104.958734125));
#4892=CARTESIAN_POINT('Ctrl Pts',(-43.4753311640868,25.6250000013656,104.958734125));
#4893=CARTESIAN_POINT('Ctrl Pts',(-74.2170326445434,25.5625000013656,74.2170326445434));
#4894=CARTESIAN_POINT('Ctrl Pts',(-104.958734125,25.5000000013656,43.4753311640869));
#4895=CARTESIAN_POINT('Ctrl Pts',(-104.958734125,25.4375000013656,0.));
#4896=CARTESIAN_POINT('Ctrl Pts',(-104.958734125,25.3750000013656,-43.4753311640868));
#4897=CARTESIAN_POINT('Ctrl Pts',(-74.2170326445434,25.3125000013656,-74.2170326445434));
#4898=CARTESIAN_POINT('Ctrl Pts',(-43.4753311640868,25.2500000013656,-104.958734125));
#4899=CARTESIAN_POINT('Ctrl Pts',(-6.42686888943697E-15,25.1875000013656,
-104.958734125));
#4900=CARTESIAN_POINT('Ctrl Pts',(43.4753311640868,25.1250000013656,-104.958734125));
#4901=CARTESIAN_POINT('Ctrl Pts',(74.2170326445434,25.0625000013656,-74.2170326445434));
#4902=CARTESIAN_POINT('Ctrl Pts',(104.958734125,25.0000000013656,-43.4753311640868));
#4903=CARTESIAN_POINT('Ctrl Pts',(104.958734125,24.9375000013656,-1.28537377788739E-14));
#4904=CARTESIAN_POINT('Ctrl Pts',(104.958734125,26.1875000013656,-1.28537377788739E-14));
#4905=CARTESIAN_POINT('Ctrl Pts',(104.958734125,26.1250000013656,43.4753311640868));
#4906=CARTESIAN_POINT('Ctrl Pts',(74.2170326445434,26.0625000013656,74.2170326445434));
#4907=CARTESIAN_POINT('Ctrl Pts',(43.4753311640869,26.0000000013656,104.958734125));
#4908=CARTESIAN_POINT('Ctrl Pts',(1.92806066683109E-14,25.9375000013656,
104.958734125));
#4909=CARTESIAN_POINT('Ctrl Pts',(-43.4753311640868,25.8750000013656,104.958734125));
#4910=CARTESIAN_POINT('Ctrl Pts',(-74.2170326445434,25.8125000013656,74.2170326445434));
#4911=CARTESIAN_POINT('Ctrl Pts',(-104.958734125,25.7500000013656,43.4753311640869));
#4912=CARTESIAN_POINT('Ctrl Pts',(-104.958734125,25.6875000013656,0.));
#4913=CARTESIAN_POINT('Ctrl Pts',(-104.958734125,25.6250000013656,-43.4753311640868));
#4914=CARTESIAN_POINT('Ctrl Pts',(-74.2170326445434,25.5625000013656,-74.2170326445434));
#4915=CARTESIAN_POINT('Ctrl Pts',(-43.4753311640868,25.5000000013656,-104.958734125));
#4916=CARTESIAN_POINT('Ctrl Pts',(-6.42686888943697E-15,25.4375000013656,
-104.958734125));
#4917=CARTESIAN_POINT('Ctrl Pts',(43.4753311640868,25.3750000013656,-104.958734125));
#4918=CARTESIAN_POINT('Ctrl Pts',(74.2170326445434,25.3125000013656,-74.2170326445434));
#4919=CARTESIAN_POINT('Ctrl Pts',(104.958734125,25.2500000013656,-43.4753311640868));
#4920=CARTESIAN_POINT('Ctrl Pts',(104.958734125,25.1875000013656,-1.28537377788739E-14));
#4921=CARTESIAN_POINT('Origin',(-7.105427357601E-14,49.5625000013656,-6.0924204042587E-14));
#4922=CARTESIAN_POINT('',(104.958734125,27.1875000013656,-6.0924204042587E-14));
#4923=CARTESIAN_POINT('',(104.958734125,26.9375000013656,-6.0924204042587E-14));
#4924=CARTESIAN_POINT('',(104.958734125,49.5625000013656,-1.089946703063E-13));
#4925=CARTESIAN_POINT('Ctrl Pts',(104.958734125,26.9375000013656,-1.28537377788739E-14));
#4926=CARTESIAN_POINT('Ctrl Pts',(104.958734125,26.8750000013656,43.4753311640868));
#4927=CARTESIAN_POINT('Ctrl Pts',(74.2170326445434,26.8125000013656,74.2170326445434));
#4928=CARTESIAN_POINT('Ctrl Pts',(43.4753311640869,26.7500000013656,104.958734125));
#4929=CARTESIAN_POINT('Ctrl Pts',(1.92806066683109E-14,26.6875000013656,
104.958734125));
#4930=CARTESIAN_POINT('Ctrl Pts',(-43.4753311640868,26.6250000013656,104.958734125));
#4931=CARTESIAN_POINT('Ctrl Pts',(-74.2170326445434,26.5625000013656,74.2170326445434));
#4932=CARTESIAN_POINT('Ctrl Pts',(-104.958734125,26.5000000013656,43.4753311640869));
#4933=CARTESIAN_POINT('Ctrl Pts',(-104.958734125,26.4375000013656,0.));
#4934=CARTESIAN_POINT('Ctrl Pts',(-104.958734125,26.3750000013656,-43.4753311640868));
#4935=CARTESIAN_POINT('Ctrl Pts',(-74.2170326445434,26.3125000013656,-74.2170326445434));
#4936=CARTESIAN_POINT('Ctrl Pts',(-43.4753311640868,26.2500000013656,-104.958734125));
#4937=CARTESIAN_POINT('Ctrl Pts',(-6.42686888943697E-15,26.1875000013656,
-104.958734125));
#4938=CARTESIAN_POINT('Ctrl Pts',(43.4753311640868,26.1250000013656,-104.958734125));
#4939=CARTESIAN_POINT('Ctrl Pts',(74.2170326445434,26.0625000013656,-74.2170326445434));
#4940=CARTESIAN_POINT('Ctrl Pts',(104.958734125,26.0000000013656,-43.4753311640868));
#4941=CARTESIAN_POINT('Ctrl Pts',(104.958734125,25.9375000013656,-1.28537377788739E-14));
#4942=CARTESIAN_POINT('Ctrl Pts',(104.958734125,27.1875000013656,-1.28537377788739E-14));
#4943=CARTESIAN_POINT('Ctrl Pts',(104.958734125,27.1250000013656,43.4753311640868));
#4944=CARTESIAN_POINT('Ctrl Pts',(74.2170326445434,27.0625000013656,74.2170326445434));
#4945=CARTESIAN_POINT('Ctrl Pts',(43.4753311640869,27.0000000013656,104.958734125));
#4946=CARTESIAN_POINT('Ctrl Pts',(1.92806066683109E-14,26.9375000013656,
104.958734125));
#4947=CARTESIAN_POINT('Ctrl Pts',(-43.4753311640868,26.8750000013656,104.958734125));
#4948=CARTESIAN_POINT('Ctrl Pts',(-74.2170326445434,26.8125000013656,74.2170326445434));
#4949=CARTESIAN_POINT('Ctrl Pts',(-104.958734125,26.7500000013656,43.4753311640869));
#4950=CARTESIAN_POINT('Ctrl Pts',(-104.958734125,26.6875000013656,0.));
#4951=CARTESIAN_POINT('Ctrl Pts',(-104.958734125,26.6250000013656,-43.4753311640868));
#4952=CARTESIAN_POINT('Ctrl Pts',(-74.2170326445434,26.5625000013656,-74.2170326445434));
#4953=CARTESIAN_POINT('Ctrl Pts',(-43.4753311640868,26.5000000013656,-104.958734125));
#4954=CARTESIAN_POINT('Ctrl Pts',(-6.42686888943697E-15,26.4375000013656,
-104.958734125));
#4955=CARTESIAN_POINT('Ctrl Pts',(43.4753311640868,26.3750000013656,-104.958734125));
#4956=CARTESIAN_POINT('Ctrl Pts',(74.2170326445434,26.3125000013656,-74.2170326445434));
#4957=CARTESIAN_POINT('Ctrl Pts',(104.958734125,26.2500000013656,-43.4753311640868));
#4958=CARTESIAN_POINT('Ctrl Pts',(104.958734125,26.1875000013656,-1.28537377788739E-14));
#4959=CARTESIAN_POINT('Origin',(-7.105427357601E-14,49.5625000013656,-6.0924204042587E-14));
#4960=CARTESIAN_POINT('',(104.958734125,28.1875000013656,-6.0924204042587E-14));
#4961=CARTESIAN_POINT('',(104.958734125,27.9375000013656,-6.0924204042587E-14));
#4962=CARTESIAN_POINT('',(104.958734125,49.5625000013656,-1.089946703063E-13));
#4963=CARTESIAN_POINT('Ctrl Pts',(104.958734125,27.9375000013656,-1.28537377788739E-14));
#4964=CARTESIAN_POINT('Ctrl Pts',(104.958734125,27.8750000013656,43.4753311640868));
#4965=CARTESIAN_POINT('Ctrl Pts',(74.2170326445434,27.8125000013656,74.2170326445434));
#4966=CARTESIAN_POINT('Ctrl Pts',(43.4753311640869,27.7500000013656,104.958734125));
#4967=CARTESIAN_POINT('Ctrl Pts',(1.92806066683109E-14,27.6875000013656,
104.958734125));
#4968=CARTESIAN_POINT('Ctrl Pts',(-43.4753311640868,27.6250000013656,104.958734125));
#4969=CARTESIAN_POINT('Ctrl Pts',(-74.2170326445434,27.5625000013656,74.2170326445434));
#4970=CARTESIAN_POINT('Ctrl Pts',(-104.958734125,27.5000000013656,43.4753311640869));
#4971=CARTESIAN_POINT('Ctrl Pts',(-104.958734125,27.4375000013656,0.));
#4972=CARTESIAN_POINT('Ctrl Pts',(-104.958734125,27.3750000013656,-43.4753311640868));
#4973=CARTESIAN_POINT('Ctrl Pts',(-74.2170326445434,27.3125000013656,-74.2170326445434));
#4974=CARTESIAN_POINT('Ctrl Pts',(-43.4753311640868,27.2500000013656,-104.958734125));
#4975=CARTESIAN_POINT('Ctrl Pts',(-6.42686888943697E-15,27.1875000013656,
-104.958734125));
#4976=CARTESIAN_POINT('Ctrl Pts',(43.4753311640868,27.1250000013656,-104.958734125));
#4977=CARTESIAN_POINT('Ctrl Pts',(74.2170326445434,27.0625000013656,-74.2170326445434));
#4978=CARTESIAN_POINT('Ctrl Pts',(104.958734125,27.0000000013656,-43.4753311640868));
#4979=CARTESIAN_POINT('Ctrl Pts',(104.958734125,26.9375000013656,-1.28537377788739E-14));
#4980=CARTESIAN_POINT('Ctrl Pts',(104.958734125,28.1875000013656,-1.28537377788739E-14));
#4981=CARTESIAN_POINT('Ctrl Pts',(104.958734125,28.1250000013656,43.4753311640868));
#4982=CARTESIAN_POINT('Ctrl Pts',(74.2170326445434,28.0625000013656,74.2170326445434));
#4983=CARTESIAN_POINT('Ctrl Pts',(43.4753311640869,28.0000000013656,104.958734125));
#4984=CARTESIAN_POINT('Ctrl Pts',(1.92806066683109E-14,27.9375000013656,
104.958734125));
#4985=CARTESIAN_POINT('Ctrl Pts',(-43.4753311640868,27.8750000013656,104.958734125));
#4986=CARTESIAN_POINT('Ctrl Pts',(-74.2170326445434,27.8125000013656,74.2170326445434));
#4987=CARTESIAN_POINT('Ctrl Pts',(-104.958734125,27.7500000013656,43.4753311640869));
#4988=CARTESIAN_POINT('Ctrl Pts',(-104.958734125,27.6875000013656,0.));
#4989=CARTESIAN_POINT('Ctrl Pts',(-104.958734125,27.6250000013656,-43.4753311640868));
#4990=CARTESIAN_POINT('Ctrl Pts',(-74.2170326445434,27.5625000013656,-74.2170326445434));
#4991=CARTESIAN_POINT('Ctrl Pts',(-43.4753311640868,27.5000000013656,-104.958734125));
#4992=CARTESIAN_POINT('Ctrl Pts',(-6.42686888943697E-15,27.4375000013656,
-104.958734125));
#4993=CARTESIAN_POINT('Ctrl Pts',(43.4753311640868,27.3750000013656,-104.958734125));
#4994=CARTESIAN_POINT('Ctrl Pts',(74.2170326445434,27.3125000013656,-74.2170326445434));
#4995=CARTESIAN_POINT('Ctrl Pts',(104.958734125,27.2500000013656,-43.4753311640868));
#4996=CARTESIAN_POINT('Ctrl Pts',(104.958734125,27.1875000013656,-1.28537377788739E-14));
#4997=CARTESIAN_POINT('Origin',(-7.105427357601E-14,49.5625000013656,-6.0924204042587E-14));
#4998=CARTESIAN_POINT('',(104.958734125,29.1875000013656,-6.0924204042587E-14));
#4999=CARTESIAN_POINT('',(104.958734125,28.9375000013656,-6.0924204042587E-14));
#5000=CARTESIAN_POINT('',(104.958734125,49.5625000013656,-1.089946703063E-13));
#5001=CARTESIAN_POINT('Ctrl Pts',(104.958734125,28.9375000013656,-1.28537377788739E-14));
#5002=CARTESIAN_POINT('Ctrl Pts',(104.958734125,28.8750000013656,43.4753311640868));
#5003=CARTESIAN_POINT('Ctrl Pts',(74.2170326445434,28.8125000013656,74.2170326445434));
#5004=CARTESIAN_POINT('Ctrl Pts',(43.4753311640869,28.7500000013656,104.958734125));
#5005=CARTESIAN_POINT('Ctrl Pts',(1.92806066683109E-14,28.6875000013656,
104.958734125));
#5006=CARTESIAN_POINT('Ctrl Pts',(-43.4753311640868,28.6250000013656,104.958734125));
#5007=CARTESIAN_POINT('Ctrl Pts',(-74.2170326445434,28.5625000013656,74.2170326445434));
#5008=CARTESIAN_POINT('Ctrl Pts',(-104.958734125,28.5000000013656,43.4753311640869));
#5009=CARTESIAN_POINT('Ctrl Pts',(-104.958734125,28.4375000013656,0.));
#5010=CARTESIAN_POINT('Ctrl Pts',(-104.958734125,28.3750000013656,-43.4753311640868));
#5011=CARTESIAN_POINT('Ctrl Pts',(-74.2170326445434,28.3125000013656,-74.2170326445434));
#5012=CARTESIAN_POINT('Ctrl Pts',(-43.4753311640868,28.2500000013656,-104.958734125));
#5013=CARTESIAN_POINT('Ctrl Pts',(-6.42686888943697E-15,28.1875000013656,
-104.958734125));
#5014=CARTESIAN_POINT('Ctrl Pts',(43.4753311640868,28.1250000013656,-104.958734125));
#5015=CARTESIAN_POINT('Ctrl Pts',(74.2170326445434,28.0625000013656,-74.2170326445434));
#5016=CARTESIAN_POINT('Ctrl Pts',(104.958734125,28.0000000013656,-43.4753311640868));
#5017=CARTESIAN_POINT('Ctrl Pts',(104.958734125,27.9375000013656,-1.28537377788739E-14));
#5018=CARTESIAN_POINT('Ctrl Pts',(104.958734125,29.1875000013656,-1.28537377788739E-14));
#5019=CARTESIAN_POINT('Ctrl Pts',(104.958734125,29.1250000013656,43.4753311640868));
#5020=CARTESIAN_POINT('Ctrl Pts',(74.2170326445434,29.0625000013656,74.2170326445434));
#5021=CARTESIAN_POINT('Ctrl Pts',(43.4753311640869,29.0000000013656,104.958734125));
#5022=CARTESIAN_POINT('Ctrl Pts',(1.92806066683109E-14,28.9375000013656,
104.958734125));
#5023=CARTESIAN_POINT('Ctrl Pts',(-43.4753311640868,28.8750000013656,104.958734125));
#5024=CARTESIAN_POINT('Ctrl Pts',(-74.2170326445434,28.8125000013656,74.2170326445434));
#5025=CARTESIAN_POINT('Ctrl Pts',(-104.958734125,28.7500000013656,43.4753311640869));
#5026=CARTESIAN_POINT('Ctrl Pts',(-104.958734125,28.6875000013656,0.));
#5027=CARTESIAN_POINT('Ctrl Pts',(-104.958734125,28.6250000013656,-43.4753311640868));
#5028=CARTESIAN_POINT('Ctrl Pts',(-74.2170326445434,28.5625000013656,-74.2170326445434));
#5029=CARTESIAN_POINT('Ctrl Pts',(-43.4753311640868,28.5000000013656,-104.958734125));
#5030=CARTESIAN_POINT('Ctrl Pts',(-6.42686888943697E-15,28.4375000013656,
-104.958734125));
#5031=CARTESIAN_POINT('Ctrl Pts',(43.4753311640868,28.3750000013656,-104.958734125));
#5032=CARTESIAN_POINT('Ctrl Pts',(74.2170326445434,28.3125000013656,-74.2170326445434));
#5033=CARTESIAN_POINT('Ctrl Pts',(104.958734125,28.2500000013656,-43.4753311640868));
#5034=CARTESIAN_POINT('Ctrl Pts',(104.958734125,28.1875000013656,-1.28537377788739E-14));
#5035=CARTESIAN_POINT('Origin',(-7.105427357601E-14,49.5625000013656,-6.0924204042587E-14));
#5036=CARTESIAN_POINT('',(104.958734125,30.1875000013656,-6.0924204042587E-14));
#5037=CARTESIAN_POINT('',(104.958734125,29.9375000013656,-6.0924204042587E-14));
#5038=CARTESIAN_POINT('',(104.958734125,49.5625000013656,-1.089946703063E-13));
#5039=CARTESIAN_POINT('Ctrl Pts',(104.958734125,29.9375000013656,-1.28537377788739E-14));
#5040=CARTESIAN_POINT('Ctrl Pts',(104.958734125,29.8750000013656,43.4753311640868));
#5041=CARTESIAN_POINT('Ctrl Pts',(74.2170326445434,29.8125000013656,74.2170326445434));
#5042=CARTESIAN_POINT('Ctrl Pts',(43.4753311640869,29.7500000013656,104.958734125));
#5043=CARTESIAN_POINT('Ctrl Pts',(1.92806066683109E-14,29.6875000013656,
104.958734125));
#5044=CARTESIAN_POINT('Ctrl Pts',(-43.4753311640868,29.6250000013656,104.958734125));
#5045=CARTESIAN_POINT('Ctrl Pts',(-74.2170326445434,29.5625000013656,74.2170326445434));
#5046=CARTESIAN_POINT('Ctrl Pts',(-104.958734125,29.5000000013656,43.4753311640869));
#5047=CARTESIAN_POINT('Ctrl Pts',(-104.958734125,29.4375000013656,0.));
#5048=CARTESIAN_POINT('Ctrl Pts',(-104.958734125,29.3750000013656,-43.4753311640868));
#5049=CARTESIAN_POINT('Ctrl Pts',(-74.2170326445434,29.3125000013656,-74.2170326445434));
#5050=CARTESIAN_POINT('Ctrl Pts',(-43.4753311640868,29.2500000013656,-104.958734125));
#5051=CARTESIAN_POINT('Ctrl Pts',(-6.42686888943697E-15,29.1875000013656,
-104.958734125));
#5052=CARTESIAN_POINT('Ctrl Pts',(43.4753311640868,29.1250000013656,-104.958734125));
#5053=CARTESIAN_POINT('Ctrl Pts',(74.2170326445434,29.0625000013656,-74.2170326445434));
#5054=CARTESIAN_POINT('Ctrl Pts',(104.958734125,29.0000000013656,-43.4753311640868));
#5055=CARTESIAN_POINT('Ctrl Pts',(104.958734125,28.9375000013656,-1.28537377788739E-14));
#5056=CARTESIAN_POINT('Ctrl Pts',(104.958734125,30.1875000013656,-1.28537377788739E-14));
#5057=CARTESIAN_POINT('Ctrl Pts',(104.958734125,30.1250000013656,43.4753311640868));
#5058=CARTESIAN_POINT('Ctrl Pts',(74.2170326445434,30.0625000013656,74.2170326445434));
#5059=CARTESIAN_POINT('Ctrl Pts',(43.4753311640869,30.0000000013656,104.958734125));
#5060=CARTESIAN_POINT('Ctrl Pts',(1.92806066683109E-14,29.9375000013656,
104.958734125));
#5061=CARTESIAN_POINT('Ctrl Pts',(-43.4753311640868,29.8750000013656,104.958734125));
#5062=CARTESIAN_POINT('Ctrl Pts',(-74.2170326445434,29.8125000013656,74.2170326445434));
#5063=CARTESIAN_POINT('Ctrl Pts',(-104.958734125,29.7500000013656,43.4753311640869));
#5064=CARTESIAN_POINT('Ctrl Pts',(-104.958734125,29.6875000013656,0.));
#5065=CARTESIAN_POINT('Ctrl Pts',(-104.958734125,29.6250000013656,-43.4753311640868));
#5066=CARTESIAN_POINT('Ctrl Pts',(-74.2170326445434,29.5625000013656,-74.2170326445434));
#5067=CARTESIAN_POINT('Ctrl Pts',(-43.4753311640868,29.5000000013656,-104.958734125));
#5068=CARTESIAN_POINT('Ctrl Pts',(-6.42686888943697E-15,29.4375000013656,
-104.958734125));
#5069=CARTESIAN_POINT('Ctrl Pts',(43.4753311640868,29.3750000013656,-104.958734125));
#5070=CARTESIAN_POINT('Ctrl Pts',(74.2170326445434,29.3125000013656,-74.2170326445434));
#5071=CARTESIAN_POINT('Ctrl Pts',(104.958734125,29.2500000013656,-43.4753311640868));
#5072=CARTESIAN_POINT('Ctrl Pts',(104.958734125,29.1875000013656,-1.28537377788739E-14));
#5073=CARTESIAN_POINT('Origin',(-7.105427357601E-14,49.5625000013656,-6.0924204042587E-14));
#5074=CARTESIAN_POINT('',(104.958734125,31.1875000013656,-6.0924204042587E-14));
#5075=CARTESIAN_POINT('',(104.958734125,30.9375000013656,-6.0924204042587E-14));
#5076=CARTESIAN_POINT('',(104.958734125,49.5625000013656,-1.089946703063E-13));
#5077=CARTESIAN_POINT('Ctrl Pts',(104.958734125,30.9375000013656,-1.28537377788739E-14));
#5078=CARTESIAN_POINT('Ctrl Pts',(104.958734125,30.8750000013656,43.4753311640868));
#5079=CARTESIAN_POINT('Ctrl Pts',(74.2170326445434,30.8125000013656,74.2170326445434));
#5080=CARTESIAN_POINT('Ctrl Pts',(43.4753311640869,30.7500000013656,104.958734125));
#5081=CARTESIAN_POINT('Ctrl Pts',(1.92806066683109E-14,30.6875000013656,
104.958734125));
#5082=CARTESIAN_POINT('Ctrl Pts',(-43.4753311640868,30.6250000013656,104.958734125));
#5083=CARTESIAN_POINT('Ctrl Pts',(-74.2170326445434,30.5625000013656,74.2170326445434));
#5084=CARTESIAN_POINT('Ctrl Pts',(-104.958734125,30.5000000013656,43.4753311640869));
#5085=CARTESIAN_POINT('Ctrl Pts',(-104.958734125,30.4375000013656,0.));
#5086=CARTESIAN_POINT('Ctrl Pts',(-104.958734125,30.3750000013656,-43.4753311640868));
#5087=CARTESIAN_POINT('Ctrl Pts',(-74.2170326445434,30.3125000013656,-74.2170326445434));
#5088=CARTESIAN_POINT('Ctrl Pts',(-43.4753311640868,30.2500000013656,-104.958734125));
#5089=CARTESIAN_POINT('Ctrl Pts',(-6.42686888943697E-15,30.1875000013656,
-104.958734125));
#5090=CARTESIAN_POINT('Ctrl Pts',(43.4753311640868,30.1250000013656,-104.958734125));
#5091=CARTESIAN_POINT('Ctrl Pts',(74.2170326445434,30.0625000013656,-74.2170326445434));
#5092=CARTESIAN_POINT('Ctrl Pts',(104.958734125,30.0000000013656,-43.4753311640868));
#5093=CARTESIAN_POINT('Ctrl Pts',(104.958734125,29.9375000013656,-1.28537377788739E-14));
#5094=CARTESIAN_POINT('Ctrl Pts',(104.958734125,31.1875000013656,-1.28537377788739E-14));
#5095=CARTESIAN_POINT('Ctrl Pts',(104.958734125,31.1250000013656,43.4753311640868));
#5096=CARTESIAN_POINT('Ctrl Pts',(74.2170326445434,31.0625000013656,74.2170326445434));
#5097=CARTESIAN_POINT('Ctrl Pts',(43.4753311640869,31.0000000013656,104.958734125));
#5098=CARTESIAN_POINT('Ctrl Pts',(1.92806066683109E-14,30.9375000013656,
104.958734125));
#5099=CARTESIAN_POINT('Ctrl Pts',(-43.4753311640868,30.8750000013656,104.958734125));
#5100=CARTESIAN_POINT('Ctrl Pts',(-74.2170326445434,30.8125000013656,74.2170326445434));
#5101=CARTESIAN_POINT('Ctrl Pts',(-104.958734125,30.7500000013656,43.4753311640869));
#5102=CARTESIAN_POINT('Ctrl Pts',(-104.958734125,30.6875000013656,0.));
#5103=CARTESIAN_POINT('Ctrl Pts',(-104.958734125,30.6250000013656,-43.4753311640868));
#5104=CARTESIAN_POINT('Ctrl Pts',(-74.2170326445434,30.5625000013656,-74.2170326445434));
#5105=CARTESIAN_POINT('Ctrl Pts',(-43.4753311640868,30.5000000013656,-104.958734125));
#5106=CARTESIAN_POINT('Ctrl Pts',(-6.42686888943697E-15,30.4375000013656,
-104.958734125));
#5107=CARTESIAN_POINT('Ctrl Pts',(43.4753311640868,30.3750000013656,-104.958734125));
#5108=CARTESIAN_POINT('Ctrl Pts',(74.2170326445434,30.3125000013656,-74.2170326445434));
#5109=CARTESIAN_POINT('Ctrl Pts',(104.958734125,30.2500000013656,-43.4753311640868));
#5110=CARTESIAN_POINT('Ctrl Pts',(104.958734125,30.1875000013656,-1.28537377788739E-14));
#5111=CARTESIAN_POINT('Origin',(-7.105427357601E-14,49.5625000013656,-6.0924204042587E-14));
#5112=CARTESIAN_POINT('',(104.958734125,32.1875000013656,-6.0924204042587E-14));
#5113=CARTESIAN_POINT('',(104.958734125,31.9375000013656,-6.0924204042587E-14));
#5114=CARTESIAN_POINT('',(104.958734125,49.5625000013656,-1.089946703063E-13));
#5115=CARTESIAN_POINT('Ctrl Pts',(104.958734125,31.9375000013656,-1.28537377788739E-14));
#5116=CARTESIAN_POINT('Ctrl Pts',(104.958734125,31.8750000013656,43.4753311640868));
#5117=CARTESIAN_POINT('Ctrl Pts',(74.2170326445434,31.8125000013656,74.2170326445434));
#5118=CARTESIAN_POINT('Ctrl Pts',(43.4753311640869,31.7500000013656,104.958734125));
#5119=CARTESIAN_POINT('Ctrl Pts',(1.92806066683109E-14,31.6875000013656,
104.958734125));
#5120=CARTESIAN_POINT('Ctrl Pts',(-43.4753311640868,31.6250000013656,104.958734125));
#5121=CARTESIAN_POINT('Ctrl Pts',(-74.2170326445434,31.5625000013656,74.2170326445434));
#5122=CARTESIAN_POINT('Ctrl Pts',(-104.958734125,31.5000000013656,43.4753311640869));
#5123=CARTESIAN_POINT('Ctrl Pts',(-104.958734125,31.4375000013656,0.));
#5124=CARTESIAN_POINT('Ctrl Pts',(-104.958734125,31.3750000013656,-43.4753311640868));
#5125=CARTESIAN_POINT('Ctrl Pts',(-74.2170326445434,31.3125000013656,-74.2170326445434));
#5126=CARTESIAN_POINT('Ctrl Pts',(-43.4753311640868,31.2500000013656,-104.958734125));
#5127=CARTESIAN_POINT('Ctrl Pts',(-6.42686888943697E-15,31.1875000013656,
-104.958734125));
#5128=CARTESIAN_POINT('Ctrl Pts',(43.4753311640868,31.1250000013656,-104.958734125));
#5129=CARTESIAN_POINT('Ctrl Pts',(74.2170326445434,31.0625000013656,-74.2170326445434));
#5130=CARTESIAN_POINT('Ctrl Pts',(104.958734125,31.0000000013656,-43.4753311640868));
#5131=CARTESIAN_POINT('Ctrl Pts',(104.958734125,30.9375000013656,-1.28537377788739E-14));
#5132=CARTESIAN_POINT('Ctrl Pts',(104.958734125,32.1875000013656,-1.28537377788739E-14));
#5133=CARTESIAN_POINT('Ctrl Pts',(104.958734125,32.1250000013656,43.4753311640868));
#5134=CARTESIAN_POINT('Ctrl Pts',(74.2170326445434,32.0625000013656,74.2170326445434));
#5135=CARTESIAN_POINT('Ctrl Pts',(43.4753311640869,32.0000000013656,104.958734125));
#5136=CARTESIAN_POINT('Ctrl Pts',(1.92806066683109E-14,31.9375000013656,
104.958734125));
#5137=CARTESIAN_POINT('Ctrl Pts',(-43.4753311640868,31.8750000013656,104.958734125));
#5138=CARTESIAN_POINT('Ctrl Pts',(-74.2170326445434,31.8125000013656,74.2170326445434));
#5139=CARTESIAN_POINT('Ctrl Pts',(-104.958734125,31.7500000013656,43.4753311640869));
#5140=CARTESIAN_POINT('Ctrl Pts',(-104.958734125,31.6875000013656,0.));
#5141=CARTESIAN_POINT('Ctrl Pts',(-104.958734125,31.6250000013656,-43.4753311640868));
#5142=CARTESIAN_POINT('Ctrl Pts',(-74.2170326445434,31.5625000013656,-74.2170326445434));
#5143=CARTESIAN_POINT('Ctrl Pts',(-43.4753311640868,31.5000000013656,-104.958734125));
#5144=CARTESIAN_POINT('Ctrl Pts',(-6.42686888943697E-15,31.4375000013656,
-104.958734125));
#5145=CARTESIAN_POINT('Ctrl Pts',(43.4753311640868,31.3750000013656,-104.958734125));
#5146=CARTESIAN_POINT('Ctrl Pts',(74.2170326445434,31.3125000013656,-74.2170326445434));
#5147=CARTESIAN_POINT('Ctrl Pts',(104.958734125,31.2500000013656,-43.4753311640868));
#5148=CARTESIAN_POINT('Ctrl Pts',(104.958734125,31.1875000013656,-1.28537377788739E-14));
#5149=CARTESIAN_POINT('Origin',(-7.105427357601E-14,49.5625000013656,-6.0924204042587E-14));
#5150=CARTESIAN_POINT('',(104.958734125,33.1875000013656,-6.0924204042587E-14));
#5151=CARTESIAN_POINT('',(104.958734125,32.9375000013656,-6.0924204042587E-14));
#5152=CARTESIAN_POINT('',(104.958734125,49.5625000013656,-1.089946703063E-13));
#5153=CARTESIAN_POINT('Ctrl Pts',(104.958734125,32.9375000013656,-1.28537377788739E-14));
#5154=CARTESIAN_POINT('Ctrl Pts',(104.958734125,32.8750000013656,43.4753311640868));
#5155=CARTESIAN_POINT('Ctrl Pts',(74.2170326445434,32.8125000013656,74.2170326445434));
#5156=CARTESIAN_POINT('Ctrl Pts',(43.4753311640869,32.7500000013656,104.958734125));
#5157=CARTESIAN_POINT('Ctrl Pts',(1.92806066683109E-14,32.6875000013656,
104.958734125));
#5158=CARTESIAN_POINT('Ctrl Pts',(-43.4753311640868,32.6250000013656,104.958734125));
#5159=CARTESIAN_POINT('Ctrl Pts',(-74.2170326445434,32.5625000013656,74.2170326445434));
#5160=CARTESIAN_POINT('Ctrl Pts',(-104.958734125,32.5000000013656,43.4753311640869));
#5161=CARTESIAN_POINT('Ctrl Pts',(-104.958734125,32.4375000013656,0.));
#5162=CARTESIAN_POINT('Ctrl Pts',(-104.958734125,32.3750000013656,-43.4753311640868));
#5163=CARTESIAN_POINT('Ctrl Pts',(-74.2170326445434,32.3125000013656,-74.2170326445434));
#5164=CARTESIAN_POINT('Ctrl Pts',(-43.4753311640868,32.2500000013656,-104.958734125));
#5165=CARTESIAN_POINT('Ctrl Pts',(-6.42686888943697E-15,32.1875000013656,
-104.958734125));
#5166=CARTESIAN_POINT('Ctrl Pts',(43.4753311640868,32.1250000013656,-104.958734125));
#5167=CARTESIAN_POINT('Ctrl Pts',(74.2170326445434,32.0625000013656,-74.2170326445434));
#5168=CARTESIAN_POINT('Ctrl Pts',(104.958734125,32.0000000013656,-43.4753311640868));
#5169=CARTESIAN_POINT('Ctrl Pts',(104.958734125,31.9375000013656,-1.28537377788739E-14));
#5170=CARTESIAN_POINT('Ctrl Pts',(104.958734125,33.1875000013656,-1.28537377788739E-14));
#5171=CARTESIAN_POINT('Ctrl Pts',(104.958734125,33.1250000013656,43.4753311640868));
#5172=CARTESIAN_POINT('Ctrl Pts',(74.2170326445434,33.0625000013656,74.2170326445434));
#5173=CARTESIAN_POINT('Ctrl Pts',(43.4753311640869,33.0000000013656,104.958734125));
#5174=CARTESIAN_POINT('Ctrl Pts',(1.92806066683109E-14,32.9375000013656,
104.958734125));
#5175=CARTESIAN_POINT('Ctrl Pts',(-43.4753311640868,32.8750000013656,104.958734125));
#5176=CARTESIAN_POINT('Ctrl Pts',(-74.2170326445434,32.8125000013656,74.2170326445434));
#5177=CARTESIAN_POINT('Ctrl Pts',(-104.958734125,32.7500000013656,43.4753311640869));
#5178=CARTESIAN_POINT('Ctrl Pts',(-104.958734125,32.6875000013656,0.));
#5179=CARTESIAN_POINT('Ctrl Pts',(-104.958734125,32.6250000013656,-43.4753311640868));
#5180=CARTESIAN_POINT('Ctrl Pts',(-74.2170326445434,32.5625000013656,-74.2170326445434));
#5181=CARTESIAN_POINT('Ctrl Pts',(-43.4753311640868,32.5000000013656,-104.958734125));
#5182=CARTESIAN_POINT('Ctrl Pts',(-6.42686888943697E-15,32.4375000013656,
-104.958734125));
#5183=CARTESIAN_POINT('Ctrl Pts',(43.4753311640868,32.3750000013656,-104.958734125));
#5184=CARTESIAN_POINT('Ctrl Pts',(74.2170326445434,32.3125000013656,-74.2170326445434));
#5185=CARTESIAN_POINT('Ctrl Pts',(104.958734125,32.2500000013656,-43.4753311640868));
#5186=CARTESIAN_POINT('Ctrl Pts',(104.958734125,32.1875000013656,-1.28537377788739E-14));
#5187=CARTESIAN_POINT('Origin',(-7.105427357601E-14,49.5625000013656,-6.0924204042587E-14));
#5188=CARTESIAN_POINT('',(104.958734125,34.1875000013656,-6.0924204042587E-14));
#5189=CARTESIAN_POINT('',(104.958734125,33.9375000013656,-6.0924204042587E-14));
#5190=CARTESIAN_POINT('',(104.958734125,49.5625000013656,-1.089946703063E-13));
#5191=CARTESIAN_POINT('Ctrl Pts',(104.958734125,33.9375000013656,-1.28537377788739E-14));
#5192=CARTESIAN_POINT('Ctrl Pts',(104.958734125,33.8750000013656,43.4753311640868));
#5193=CARTESIAN_POINT('Ctrl Pts',(74.2170326445434,33.8125000013656,74.2170326445434));
#5194=CARTESIAN_POINT('Ctrl Pts',(43.4753311640869,33.7500000013656,104.958734125));
#5195=CARTESIAN_POINT('Ctrl Pts',(1.92806066683109E-14,33.6875000013656,
104.958734125));
#5196=CARTESIAN_POINT('Ctrl Pts',(-43.4753311640868,33.6250000013656,104.958734125));
#5197=CARTESIAN_POINT('Ctrl Pts',(-74.2170326445434,33.5625000013656,74.2170326445434));
#5198=CARTESIAN_POINT('Ctrl Pts',(-104.958734125,33.5000000013656,43.4753311640869));
#5199=CARTESIAN_POINT('Ctrl Pts',(-104.958734125,33.4375000013656,0.));
#5200=CARTESIAN_POINT('Ctrl Pts',(-104.958734125,33.3750000013656,-43.4753311640868));
#5201=CARTESIAN_POINT('Ctrl Pts',(-74.2170326445434,33.3125000013656,-74.2170326445434));
#5202=CARTESIAN_POINT('Ctrl Pts',(-43.4753311640868,33.2500000013656,-104.958734125));
#5203=CARTESIAN_POINT('Ctrl Pts',(-6.42686888943697E-15,33.1875000013656,
-104.958734125));
#5204=CARTESIAN_POINT('Ctrl Pts',(43.4753311640868,33.1250000013656,-104.958734125));
#5205=CARTESIAN_POINT('Ctrl Pts',(74.2170326445434,33.0625000013656,-74.2170326445434));
#5206=CARTESIAN_POINT('Ctrl Pts',(104.958734125,33.0000000013656,-43.4753311640868));
#5207=CARTESIAN_POINT('Ctrl Pts',(104.958734125,32.9375000013656,-1.28537377788739E-14));
#5208=CARTESIAN_POINT('Ctrl Pts',(104.958734125,34.1875000013656,-1.28537377788739E-14));
#5209=CARTESIAN_POINT('Ctrl Pts',(104.958734125,34.1250000013656,43.4753311640868));
#5210=CARTESIAN_POINT('Ctrl Pts',(74.2170326445434,34.0625000013656,74.2170326445434));
#5211=CARTESIAN_POINT('Ctrl Pts',(43.4753311640869,34.0000000013656,104.958734125));
#5212=CARTESIAN_POINT('Ctrl Pts',(1.92806066683109E-14,33.9375000013656,
104.958734125));
#5213=CARTESIAN_POINT('Ctrl Pts',(-43.4753311640868,33.8750000013656,104.958734125));
#5214=CARTESIAN_POINT('Ctrl Pts',(-74.2170326445434,33.8125000013656,74.2170326445434));
#5215=CARTESIAN_POINT('Ctrl Pts',(-104.958734125,33.7500000013656,43.4753311640869));
#5216=CARTESIAN_POINT('Ctrl Pts',(-104.958734125,33.6875000013656,0.));
#5217=CARTESIAN_POINT('Ctrl Pts',(-104.958734125,33.6250000013656,-43.4753311640868));
#5218=CARTESIAN_POINT('Ctrl Pts',(-74.2170326445434,33.5625000013656,-74.2170326445434));
#5219=CARTESIAN_POINT('Ctrl Pts',(-43.4753311640868,33.5000000013656,-104.958734125));
#5220=CARTESIAN_POINT('Ctrl Pts',(-6.42686888943697E-15,33.4375000013656,
-104.958734125));
#5221=CARTESIAN_POINT('Ctrl Pts',(43.4753311640868,33.3750000013656,-104.958734125));
#5222=CARTESIAN_POINT('Ctrl Pts',(74.2170326445434,33.3125000013656,-74.2170326445434));
#5223=CARTESIAN_POINT('Ctrl Pts',(104.958734125,33.2500000013656,-43.4753311640868));
#5224=CARTESIAN_POINT('Ctrl Pts',(104.958734125,33.1875000013656,-1.28537377788739E-14));
#5225=CARTESIAN_POINT('Origin',(-7.105427357601E-14,49.5625000013656,-6.0924204042587E-14));
#5226=CARTESIAN_POINT('',(104.958734125,35.1875000013656,-6.0924204042587E-14));
#5227=CARTESIAN_POINT('',(104.958734125,34.9375000013656,-6.0924204042587E-14));
#5228=CARTESIAN_POINT('',(104.958734125,49.5625000013656,-1.089946703063E-13));
#5229=CARTESIAN_POINT('Ctrl Pts',(104.958734125,34.9375000013656,-1.28537377788739E-14));
#5230=CARTESIAN_POINT('Ctrl Pts',(104.958734125,34.8750000013656,43.4753311640868));
#5231=CARTESIAN_POINT('Ctrl Pts',(74.2170326445434,34.8125000013656,74.2170326445434));
#5232=CARTESIAN_POINT('Ctrl Pts',(43.4753311640869,34.7500000013656,104.958734125));
#5233=CARTESIAN_POINT('Ctrl Pts',(1.92806066683109E-14,34.6875000013656,
104.958734125));
#5234=CARTESIAN_POINT('Ctrl Pts',(-43.4753311640868,34.6250000013656,104.958734125));
#5235=CARTESIAN_POINT('Ctrl Pts',(-74.2170326445434,34.5625000013656,74.2170326445434));
#5236=CARTESIAN_POINT('Ctrl Pts',(-104.958734125,34.5000000013656,43.4753311640869));
#5237=CARTESIAN_POINT('Ctrl Pts',(-104.958734125,34.4375000013656,0.));
#5238=CARTESIAN_POINT('Ctrl Pts',(-104.958734125,34.3750000013656,-43.4753311640868));
#5239=CARTESIAN_POINT('Ctrl Pts',(-74.2170326445434,34.3125000013656,-74.2170326445434));
#5240=CARTESIAN_POINT('Ctrl Pts',(-43.4753311640868,34.2500000013656,-104.958734125));
#5241=CARTESIAN_POINT('Ctrl Pts',(-6.42686888943697E-15,34.1875000013656,
-104.958734125));
#5242=CARTESIAN_POINT('Ctrl Pts',(43.4753311640868,34.1250000013656,-104.958734125));
#5243=CARTESIAN_POINT('Ctrl Pts',(74.2170326445434,34.0625000013656,-74.2170326445434));
#5244=CARTESIAN_POINT('Ctrl Pts',(104.958734125,34.0000000013656,-43.4753311640868));
#5245=CARTESIAN_POINT('Ctrl Pts',(104.958734125,33.9375000013656,-1.28537377788739E-14));
#5246=CARTESIAN_POINT('Ctrl Pts',(104.958734125,35.1875000013656,-1.28537377788739E-14));
#5247=CARTESIAN_POINT('Ctrl Pts',(104.958734125,35.1250000013656,43.4753311640868));
#5248=CARTESIAN_POINT('Ctrl Pts',(74.2170326445434,35.0625000013656,74.2170326445434));
#5249=CARTESIAN_POINT('Ctrl Pts',(43.4753311640869,35.0000000013656,104.958734125));
#5250=CARTESIAN_POINT('Ctrl Pts',(1.92806066683109E-14,34.9375000013656,
104.958734125));
#5251=CARTESIAN_POINT('Ctrl Pts',(-43.4753311640868,34.8750000013656,104.958734125));
#5252=CARTESIAN_POINT('Ctrl Pts',(-74.2170326445434,34.8125000013656,74.2170326445434));
#5253=CARTESIAN_POINT('Ctrl Pts',(-104.958734125,34.7500000013656,43.4753311640869));
#5254=CARTESIAN_POINT('Ctrl Pts',(-104.958734125,34.6875000013656,0.));
#5255=CARTESIAN_POINT('Ctrl Pts',(-104.958734125,34.6250000013656,-43.4753311640868));
#5256=CARTESIAN_POINT('Ctrl Pts',(-74.2170326445434,34.5625000013656,-74.2170326445434));
#5257=CARTESIAN_POINT('Ctrl Pts',(-43.4753311640868,34.5000000013656,-104.958734125));
#5258=CARTESIAN_POINT('Ctrl Pts',(-6.42686888943697E-15,34.4375000013656,
-104.958734125));
#5259=CARTESIAN_POINT('Ctrl Pts',(43.4753311640868,34.3750000013656,-104.958734125));
#5260=CARTESIAN_POINT('Ctrl Pts',(74.2170326445434,34.3125000013656,-74.2170326445434));
#5261=CARTESIAN_POINT('Ctrl Pts',(104.958734125,34.2500000013656,-43.4753311640868));
#5262=CARTESIAN_POINT('Ctrl Pts',(104.958734125,34.1875000013656,-1.28537377788739E-14));
#5263=CARTESIAN_POINT('Origin',(-7.105427357601E-14,49.5625000013656,-6.0924204042587E-14));
#5264=CARTESIAN_POINT('',(104.958734125,36.1875000013656,-6.0924204042587E-14));
#5265=CARTESIAN_POINT('',(104.958734125,35.9375000013656,-6.0924204042587E-14));
#5266=CARTESIAN_POINT('',(104.958734125,49.5625000013656,-1.089946703063E-13));
#5267=CARTESIAN_POINT('Ctrl Pts',(104.958734125,35.9375000013656,-1.28537377788739E-14));
#5268=CARTESIAN_POINT('Ctrl Pts',(104.958734125,35.8750000013656,43.4753311640868));
#5269=CARTESIAN_POINT('Ctrl Pts',(74.2170326445434,35.8125000013656,74.2170326445434));
#5270=CARTESIAN_POINT('Ctrl Pts',(43.4753311640869,35.7500000013656,104.958734125));
#5271=CARTESIAN_POINT('Ctrl Pts',(1.92806066683109E-14,35.6875000013656,
104.958734125));
#5272=CARTESIAN_POINT('Ctrl Pts',(-43.4753311640868,35.6250000013656,104.958734125));
#5273=CARTESIAN_POINT('Ctrl Pts',(-74.2170326445434,35.5625000013656,74.2170326445434));
#5274=CARTESIAN_POINT('Ctrl Pts',(-104.958734125,35.5000000013656,43.4753311640869));
#5275=CARTESIAN_POINT('Ctrl Pts',(-104.958734125,35.4375000013656,0.));
#5276=CARTESIAN_POINT('Ctrl Pts',(-104.958734125,35.3750000013656,-43.4753311640868));
#5277=CARTESIAN_POINT('Ctrl Pts',(-74.2170326445434,35.3125000013656,-74.2170326445434));
#5278=CARTESIAN_POINT('Ctrl Pts',(-43.4753311640868,35.2500000013656,-104.958734125));
#5279=CARTESIAN_POINT('Ctrl Pts',(-6.42686888943697E-15,35.1875000013656,
-104.958734125));
#5280=CARTESIAN_POINT('Ctrl Pts',(43.4753311640868,35.1250000013656,-104.958734125));
#5281=CARTESIAN_POINT('Ctrl Pts',(74.2170326445434,35.0625000013656,-74.2170326445434));
#5282=CARTESIAN_POINT('Ctrl Pts',(104.958734125,35.0000000013656,-43.4753311640868));
#5283=CARTESIAN_POINT('Ctrl Pts',(104.958734125,34.9375000013656,-1.28537377788739E-14));
#5284=CARTESIAN_POINT('Ctrl Pts',(104.958734125,36.1875000013656,-1.28537377788739E-14));
#5285=CARTESIAN_POINT('Ctrl Pts',(104.958734125,36.1250000013656,43.4753311640868));
#5286=CARTESIAN_POINT('Ctrl Pts',(74.2170326445434,36.0625000013656,74.2170326445434));
#5287=CARTESIAN_POINT('Ctrl Pts',(43.4753311640869,36.0000000013656,104.958734125));
#5288=CARTESIAN_POINT('Ctrl Pts',(1.92806066683109E-14,35.9375000013656,
104.958734125));
#5289=CARTESIAN_POINT('Ctrl Pts',(-43.4753311640868,35.8750000013656,104.958734125));
#5290=CARTESIAN_POINT('Ctrl Pts',(-74.2170326445434,35.8125000013656,74.2170326445434));
#5291=CARTESIAN_POINT('Ctrl Pts',(-104.958734125,35.7500000013656,43.4753311640869));
#5292=CARTESIAN_POINT('Ctrl Pts',(-104.958734125,35.6875000013656,0.));
#5293=CARTESIAN_POINT('Ctrl Pts',(-104.958734125,35.6250000013656,-43.4753311640868));
#5294=CARTESIAN_POINT('Ctrl Pts',(-74.2170326445434,35.5625000013656,-74.2170326445434));
#5295=CARTESIAN_POINT('Ctrl Pts',(-43.4753311640868,35.5000000013656,-104.958734125));
#5296=CARTESIAN_POINT('Ctrl Pts',(-6.42686888943697E-15,35.4375000013656,
-104.958734125));
#5297=CARTESIAN_POINT('Ctrl Pts',(43.4753311640868,35.3750000013656,-104.958734125));
#5298=CARTESIAN_POINT('Ctrl Pts',(74.2170326445434,35.3125000013656,-74.2170326445434));
#5299=CARTESIAN_POINT('Ctrl Pts',(104.958734125,35.2500000013656,-43.4753311640868));
#5300=CARTESIAN_POINT('Ctrl Pts',(104.958734125,35.1875000013656,-1.28537377788739E-14));
#5301=CARTESIAN_POINT('Origin',(-7.105427357601E-14,49.5625000013656,-6.0924204042587E-14));
#5302=CARTESIAN_POINT('',(104.958734125,37.1875000013656,-6.0924204042587E-14));
#5303=CARTESIAN_POINT('',(104.958734125,36.9375000013656,-6.0924204042587E-14));
#5304=CARTESIAN_POINT('',(104.958734125,49.5625000013656,-1.089946703063E-13));
#5305=CARTESIAN_POINT('Ctrl Pts',(104.958734125,36.9375000013656,-1.28537377788739E-14));
#5306=CARTESIAN_POINT('Ctrl Pts',(104.958734125,36.8750000013656,43.4753311640868));
#5307=CARTESIAN_POINT('Ctrl Pts',(74.2170326445434,36.8125000013656,74.2170326445434));
#5308=CARTESIAN_POINT('Ctrl Pts',(43.4753311640869,36.7500000013656,104.958734125));
#5309=CARTESIAN_POINT('Ctrl Pts',(1.92806066683109E-14,36.6875000013656,
104.958734125));
#5310=CARTESIAN_POINT('Ctrl Pts',(-43.4753311640868,36.6250000013656,104.958734125));
#5311=CARTESIAN_POINT('Ctrl Pts',(-74.2170326445434,36.5625000013656,74.2170326445434));
#5312=CARTESIAN_POINT('Ctrl Pts',(-104.958734125,36.5000000013656,43.4753311640869));
#5313=CARTESIAN_POINT('Ctrl Pts',(-104.958734125,36.4375000013656,0.));
#5314=CARTESIAN_POINT('Ctrl Pts',(-104.958734125,36.3750000013656,-43.4753311640868));
#5315=CARTESIAN_POINT('Ctrl Pts',(-74.2170326445434,36.3125000013656,-74.2170326445434));
#5316=CARTESIAN_POINT('Ctrl Pts',(-43.4753311640868,36.2500000013656,-104.958734125));
#5317=CARTESIAN_POINT('Ctrl Pts',(-6.42686888943697E-15,36.1875000013656,
-104.958734125));
#5318=CARTESIAN_POINT('Ctrl Pts',(43.4753311640868,36.1250000013656,-104.958734125));
#5319=CARTESIAN_POINT('Ctrl Pts',(74.2170326445434,36.0625000013656,-74.2170326445434));
#5320=CARTESIAN_POINT('Ctrl Pts',(104.958734125,36.0000000013656,-43.4753311640868));
#5321=CARTESIAN_POINT('Ctrl Pts',(104.958734125,35.9375000013656,-1.28537377788739E-14));
#5322=CARTESIAN_POINT('Ctrl Pts',(104.958734125,37.1875000013656,-1.28537377788739E-14));
#5323=CARTESIAN_POINT('Ctrl Pts',(104.958734125,37.1250000013656,43.4753311640868));
#5324=CARTESIAN_POINT('Ctrl Pts',(74.2170326445434,37.0625000013656,74.2170326445434));
#5325=CARTESIAN_POINT('Ctrl Pts',(43.4753311640869,37.0000000013656,104.958734125));
#5326=CARTESIAN_POINT('Ctrl Pts',(1.92806066683109E-14,36.9375000013656,
104.958734125));
#5327=CARTESIAN_POINT('Ctrl Pts',(-43.4753311640868,36.8750000013656,104.958734125));
#5328=CARTESIAN_POINT('Ctrl Pts',(-74.2170326445434,36.8125000013656,74.2170326445434));
#5329=CARTESIAN_POINT('Ctrl Pts',(-104.958734125,36.7500000013656,43.4753311640869));
#5330=CARTESIAN_POINT('Ctrl Pts',(-104.958734125,36.6875000013656,0.));
#5331=CARTESIAN_POINT('Ctrl Pts',(-104.958734125,36.6250000013656,-43.4753311640868));
#5332=CARTESIAN_POINT('Ctrl Pts',(-74.2170326445434,36.5625000013656,-74.2170326445434));
#5333=CARTESIAN_POINT('Ctrl Pts',(-43.4753311640868,36.5000000013656,-104.958734125));
#5334=CARTESIAN_POINT('Ctrl Pts',(-6.42686888943697E-15,36.4375000013656,
-104.958734125));
#5335=CARTESIAN_POINT('Ctrl Pts',(43.4753311640868,36.3750000013656,-104.958734125));
#5336=CARTESIAN_POINT('Ctrl Pts',(74.2170326445434,36.3125000013656,-74.2170326445434));
#5337=CARTESIAN_POINT('Ctrl Pts',(104.958734125,36.2500000013656,-43.4753311640868));
#5338=CARTESIAN_POINT('Ctrl Pts',(104.958734125,36.1875000013656,-1.28537377788739E-14));
#5339=CARTESIAN_POINT('Origin',(-7.105427357601E-14,49.5625000013656,-6.0924204042587E-14));
#5340=CARTESIAN_POINT('',(104.958734125,38.1875000013656,-6.0924204042587E-14));
#5341=CARTESIAN_POINT('',(104.958734125,37.9375000013656,-6.0924204042587E-14));
#5342=CARTESIAN_POINT('',(104.958734125,49.5625000013656,-1.089946703063E-13));
#5343=CARTESIAN_POINT('Ctrl Pts',(104.958734125,37.9375000013656,-1.28537377788739E-14));
#5344=CARTESIAN_POINT('Ctrl Pts',(104.958734125,37.8750000013656,43.4753311640868));
#5345=CARTESIAN_POINT('Ctrl Pts',(74.2170326445434,37.8125000013656,74.2170326445434));
#5346=CARTESIAN_POINT('Ctrl Pts',(43.4753311640869,37.7500000013656,104.958734125));
#5347=CARTESIAN_POINT('Ctrl Pts',(1.92806066683109E-14,37.6875000013656,
104.958734125));
#5348=CARTESIAN_POINT('Ctrl Pts',(-43.4753311640868,37.6250000013656,104.958734125));
#5349=CARTESIAN_POINT('Ctrl Pts',(-74.2170326445434,37.5625000013656,74.2170326445434));
#5350=CARTESIAN_POINT('Ctrl Pts',(-104.958734125,37.5000000013656,43.4753311640869));
#5351=CARTESIAN_POINT('Ctrl Pts',(-104.958734125,37.4375000013656,0.));
#5352=CARTESIAN_POINT('Ctrl Pts',(-104.958734125,37.3750000013656,-43.4753311640868));
#5353=CARTESIAN_POINT('Ctrl Pts',(-74.2170326445434,37.3125000013656,-74.2170326445434));
#5354=CARTESIAN_POINT('Ctrl Pts',(-43.4753311640868,37.2500000013656,-104.958734125));
#5355=CARTESIAN_POINT('Ctrl Pts',(-6.42686888943697E-15,37.1875000013656,
-104.958734125));
#5356=CARTESIAN_POINT('Ctrl Pts',(43.4753311640868,37.1250000013656,-104.958734125));
#5357=CARTESIAN_POINT('Ctrl Pts',(74.2170326445434,37.0625000013656,-74.2170326445434));
#5358=CARTESIAN_POINT('Ctrl Pts',(104.958734125,37.0000000013656,-43.4753311640868));
#5359=CARTESIAN_POINT('Ctrl Pts',(104.958734125,36.9375000013656,-1.28537377788739E-14));
#5360=CARTESIAN_POINT('Ctrl Pts',(104.958734125,38.1875000013656,-1.28537377788739E-14));
#5361=CARTESIAN_POINT('Ctrl Pts',(104.958734125,38.1250000013656,43.4753311640868));
#5362=CARTESIAN_POINT('Ctrl Pts',(74.2170326445434,38.0625000013656,74.2170326445434));
#5363=CARTESIAN_POINT('Ctrl Pts',(43.4753311640869,38.0000000013656,104.958734125));
#5364=CARTESIAN_POINT('Ctrl Pts',(1.92806066683109E-14,37.9375000013656,
104.958734125));
#5365=CARTESIAN_POINT('Ctrl Pts',(-43.4753311640868,37.8750000013656,104.958734125));
#5366=CARTESIAN_POINT('Ctrl Pts',(-74.2170326445434,37.8125000013656,74.2170326445434));
#5367=CARTESIAN_POINT('Ctrl Pts',(-104.958734125,37.7500000013656,43.4753311640869));
#5368=CARTESIAN_POINT('Ctrl Pts',(-104.958734125,37.6875000013656,0.));
#5369=CARTESIAN_POINT('Ctrl Pts',(-104.958734125,37.6250000013656,-43.4753311640868));
#5370=CARTESIAN_POINT('Ctrl Pts',(-74.2170326445434,37.5625000013656,-74.2170326445434));
#5371=CARTESIAN_POINT('Ctrl Pts',(-43.4753311640868,37.5000000013656,-104.958734125));
#5372=CARTESIAN_POINT('Ctrl Pts',(-6.42686888943697E-15,37.4375000013656,
-104.958734125));
#5373=CARTESIAN_POINT('Ctrl Pts',(43.4753311640868,37.3750000013656,-104.958734125));
#5374=CARTESIAN_POINT('Ctrl Pts',(74.2170326445434,37.3125000013656,-74.2170326445434));
#5375=CARTESIAN_POINT('Ctrl Pts',(104.958734125,37.2500000013656,-43.4753311640868));
#5376=CARTESIAN_POINT('Ctrl Pts',(104.958734125,37.1875000013656,-1.28537377788739E-14));
#5377=CARTESIAN_POINT('Origin',(-7.105427357601E-14,49.5625000013656,-6.0924204042587E-14));
#5378=CARTESIAN_POINT('',(104.958734125,39.1875000013656,-6.0924204042587E-14));
#5379=CARTESIAN_POINT('',(104.958734125,38.9375000013656,-6.0924204042587E-14));
#5380=CARTESIAN_POINT('',(104.958734125,49.5625000013656,-1.089946703063E-13));
#5381=CARTESIAN_POINT('Ctrl Pts',(104.958734125,38.9375000013656,-1.28537377788739E-14));
#5382=CARTESIAN_POINT('Ctrl Pts',(104.958734125,38.8750000013656,43.4753311640868));
#5383=CARTESIAN_POINT('Ctrl Pts',(74.2170326445434,38.8125000013656,74.2170326445434));
#5384=CARTESIAN_POINT('Ctrl Pts',(43.4753311640869,38.7500000013656,104.958734125));
#5385=CARTESIAN_POINT('Ctrl Pts',(1.92806066683109E-14,38.6875000013656,
104.958734125));
#5386=CARTESIAN_POINT('Ctrl Pts',(-43.4753311640868,38.6250000013656,104.958734125));
#5387=CARTESIAN_POINT('Ctrl Pts',(-74.2170326445434,38.5625000013656,74.2170326445434));
#5388=CARTESIAN_POINT('Ctrl Pts',(-104.958734125,38.5000000013656,43.4753311640869));
#5389=CARTESIAN_POINT('Ctrl Pts',(-104.958734125,38.4375000013656,0.));
#5390=CARTESIAN_POINT('Ctrl Pts',(-104.958734125,38.3750000013656,-43.4753311640868));
#5391=CARTESIAN_POINT('Ctrl Pts',(-74.2170326445434,38.3125000013656,-74.2170326445434));
#5392=CARTESIAN_POINT('Ctrl Pts',(-43.4753311640868,38.2500000013656,-104.958734125));
#5393=CARTESIAN_POINT('Ctrl Pts',(-6.42686888943697E-15,38.1875000013656,
-104.958734125));
#5394=CARTESIAN_POINT('Ctrl Pts',(43.4753311640868,38.1250000013656,-104.958734125));
#5395=CARTESIAN_POINT('Ctrl Pts',(74.2170326445434,38.0625000013656,-74.2170326445434));
#5396=CARTESIAN_POINT('Ctrl Pts',(104.958734125,38.0000000013656,-43.4753311640868));
#5397=CARTESIAN_POINT('Ctrl Pts',(104.958734125,37.9375000013656,-1.28537377788739E-14));
#5398=CARTESIAN_POINT('Ctrl Pts',(104.958734125,39.1875000013656,-1.28537377788739E-14));
#5399=CARTESIAN_POINT('Ctrl Pts',(104.958734125,39.1250000013656,43.4753311640868));
#5400=CARTESIAN_POINT('Ctrl Pts',(74.2170326445434,39.0625000013656,74.2170326445434));
#5401=CARTESIAN_POINT('Ctrl Pts',(43.4753311640869,39.0000000013656,104.958734125));
#5402=CARTESIAN_POINT('Ctrl Pts',(1.92806066683109E-14,38.9375000013656,
104.958734125));
#5403=CARTESIAN_POINT('Ctrl Pts',(-43.4753311640868,38.8750000013656,104.958734125));
#5404=CARTESIAN_POINT('Ctrl Pts',(-74.2170326445434,38.8125000013656,74.2170326445434));
#5405=CARTESIAN_POINT('Ctrl Pts',(-104.958734125,38.7500000013656,43.4753311640869));
#5406=CARTESIAN_POINT('Ctrl Pts',(-104.958734125,38.6875000013656,0.));
#5407=CARTESIAN_POINT('Ctrl Pts',(-104.958734125,38.6250000013656,-43.4753311640868));
#5408=CARTESIAN_POINT('Ctrl Pts',(-74.2170326445434,38.5625000013656,-74.2170326445434));
#5409=CARTESIAN_POINT('Ctrl Pts',(-43.4753311640868,38.5000000013656,-104.958734125));
#5410=CARTESIAN_POINT('Ctrl Pts',(-6.42686888943697E-15,38.4375000013656,
-104.958734125));
#5411=CARTESIAN_POINT('Ctrl Pts',(43.4753311640868,38.3750000013656,-104.958734125));
#5412=CARTESIAN_POINT('Ctrl Pts',(74.2170326445434,38.3125000013656,-74.2170326445434));
#5413=CARTESIAN_POINT('Ctrl Pts',(104.958734125,38.2500000013656,-43.4753311640868));
#5414=CARTESIAN_POINT('Ctrl Pts',(104.958734125,38.1875000013656,-1.28537377788739E-14));
#5415=CARTESIAN_POINT('Origin',(-7.105427357601E-14,49.5625000013656,-6.0924204042587E-14));
#5416=CARTESIAN_POINT('',(104.958734125,40.1875000013656,-6.0924204042587E-14));
#5417=CARTESIAN_POINT('',(104.958734125,39.9375000013656,-6.0924204042587E-14));
#5418=CARTESIAN_POINT('',(104.958734125,49.5625000013656,-1.089946703063E-13));
#5419=CARTESIAN_POINT('Ctrl Pts',(104.958734125,39.9375000013656,-1.28537377788739E-14));
#5420=CARTESIAN_POINT('Ctrl Pts',(104.958734125,39.8750000013656,43.4753311640868));
#5421=CARTESIAN_POINT('Ctrl Pts',(74.2170326445434,39.8125000013656,74.2170326445434));
#5422=CARTESIAN_POINT('Ctrl Pts',(43.4753311640869,39.7500000013656,104.958734125));
#5423=CARTESIAN_POINT('Ctrl Pts',(1.92806066683109E-14,39.6875000013656,
104.958734125));
#5424=CARTESIAN_POINT('Ctrl Pts',(-43.4753311640868,39.6250000013656,104.958734125));
#5425=CARTESIAN_POINT('Ctrl Pts',(-74.2170326445434,39.5625000013656,74.2170326445434));
#5426=CARTESIAN_POINT('Ctrl Pts',(-104.958734125,39.5000000013656,43.4753311640869));
#5427=CARTESIAN_POINT('Ctrl Pts',(-104.958734125,39.4375000013656,0.));
#5428=CARTESIAN_POINT('Ctrl Pts',(-104.958734125,39.3750000013656,-43.4753311640868));
#5429=CARTESIAN_POINT('Ctrl Pts',(-74.2170326445434,39.3125000013656,-74.2170326445434));
#5430=CARTESIAN_POINT('Ctrl Pts',(-43.4753311640868,39.2500000013656,-104.958734125));
#5431=CARTESIAN_POINT('Ctrl Pts',(-6.42686888943697E-15,39.1875000013656,
-104.958734125));
#5432=CARTESIAN_POINT('Ctrl Pts',(43.4753311640868,39.1250000013656,-104.958734125));
#5433=CARTESIAN_POINT('Ctrl Pts',(74.2170326445434,39.0625000013656,-74.2170326445434));
#5434=CARTESIAN_POINT('Ctrl Pts',(104.958734125,39.0000000013656,-43.4753311640868));
#5435=CARTESIAN_POINT('Ctrl Pts',(104.958734125,38.9375000013656,-1.28537377788739E-14));
#5436=CARTESIAN_POINT('Ctrl Pts',(104.958734125,40.1875000013656,-1.28537377788739E-14));
#5437=CARTESIAN_POINT('Ctrl Pts',(104.958734125,40.1250000013656,43.4753311640868));
#5438=CARTESIAN_POINT('Ctrl Pts',(74.2170326445434,40.0625000013656,74.2170326445434));
#5439=CARTESIAN_POINT('Ctrl Pts',(43.4753311640869,40.0000000013656,104.958734125));
#5440=CARTESIAN_POINT('Ctrl Pts',(1.92806066683109E-14,39.9375000013656,
104.958734125));
#5441=CARTESIAN_POINT('Ctrl Pts',(-43.4753311640868,39.8750000013656,104.958734125));
#5442=CARTESIAN_POINT('Ctrl Pts',(-74.2170326445434,39.8125000013656,74.2170326445434));
#5443=CARTESIAN_POINT('Ctrl Pts',(-104.958734125,39.7500000013656,43.4753311640869));
#5444=CARTESIAN_POINT('Ctrl Pts',(-104.958734125,39.6875000013656,0.));
#5445=CARTESIAN_POINT('Ctrl Pts',(-104.958734125,39.6250000013656,-43.4753311640868));
#5446=CARTESIAN_POINT('Ctrl Pts',(-74.2170326445434,39.5625000013656,-74.2170326445434));
#5447=CARTESIAN_POINT('Ctrl Pts',(-43.4753311640868,39.5000000013656,-104.958734125));
#5448=CARTESIAN_POINT('Ctrl Pts',(-6.42686888943697E-15,39.4375000013656,
-104.958734125));
#5449=CARTESIAN_POINT('Ctrl Pts',(43.4753311640868,39.3750000013656,-104.958734125));
#5450=CARTESIAN_POINT('Ctrl Pts',(74.2170326445434,39.3125000013656,-74.2170326445434));
#5451=CARTESIAN_POINT('Ctrl Pts',(104.958734125,39.2500000013656,-43.4753311640868));
#5452=CARTESIAN_POINT('Ctrl Pts',(104.958734125,39.1875000013656,-1.28537377788739E-14));
#5453=CARTESIAN_POINT('Origin',(-7.105427357601E-14,49.5625000013656,-6.0924204042587E-14));
#5454=CARTESIAN_POINT('',(104.958734125,41.1875000013656,-6.0924204042587E-14));
#5455=CARTESIAN_POINT('',(104.958734125,40.9375000013656,-6.0924204042587E-14));
#5456=CARTESIAN_POINT('',(104.958734125,49.5625000013656,-1.089946703063E-13));
#5457=CARTESIAN_POINT('Ctrl Pts',(104.958734125,40.9375000013656,-1.28537377788739E-14));
#5458=CARTESIAN_POINT('Ctrl Pts',(104.958734125,40.8750000013656,43.4753311640868));
#5459=CARTESIAN_POINT('Ctrl Pts',(74.2170326445434,40.8125000013656,74.2170326445434));
#5460=CARTESIAN_POINT('Ctrl Pts',(43.4753311640869,40.7500000013656,104.958734125));
#5461=CARTESIAN_POINT('Ctrl Pts',(1.92806066683109E-14,40.6875000013656,
104.958734125));
#5462=CARTESIAN_POINT('Ctrl Pts',(-43.4753311640868,40.6250000013656,104.958734125));
#5463=CARTESIAN_POINT('Ctrl Pts',(-74.2170326445434,40.5625000013656,74.2170326445434));
#5464=CARTESIAN_POINT('Ctrl Pts',(-104.958734125,40.5000000013656,43.4753311640869));
#5465=CARTESIAN_POINT('Ctrl Pts',(-104.958734125,40.4375000013656,0.));
#5466=CARTESIAN_POINT('Ctrl Pts',(-104.958734125,40.3750000013656,-43.4753311640868));
#5467=CARTESIAN_POINT('Ctrl Pts',(-74.2170326445434,40.3125000013656,-74.2170326445434));
#5468=CARTESIAN_POINT('Ctrl Pts',(-43.4753311640868,40.2500000013656,-104.958734125));
#5469=CARTESIAN_POINT('Ctrl Pts',(-6.42686888943697E-15,40.1875000013656,
-104.958734125));
#5470=CARTESIAN_POINT('Ctrl Pts',(43.4753311640868,40.1250000013656,-104.958734125));
#5471=CARTESIAN_POINT('Ctrl Pts',(74.2170326445434,40.0625000013656,-74.2170326445434));
#5472=CARTESIAN_POINT('Ctrl Pts',(104.958734125,40.0000000013656,-43.4753311640868));
#5473=CARTESIAN_POINT('Ctrl Pts',(104.958734125,39.9375000013656,-1.28537377788739E-14));
#5474=CARTESIAN_POINT('Ctrl Pts',(104.958734125,41.1875000013656,-1.28537377788739E-14));
#5475=CARTESIAN_POINT('Ctrl Pts',(104.958734125,41.1250000013656,43.4753311640868));
#5476=CARTESIAN_POINT('Ctrl Pts',(74.2170326445434,41.0625000013656,74.2170326445434));
#5477=CARTESIAN_POINT('Ctrl Pts',(43.4753311640869,41.0000000013656,104.958734125));
#5478=CARTESIAN_POINT('Ctrl Pts',(1.92806066683109E-14,40.9375000013656,
104.958734125));
#5479=CARTESIAN_POINT('Ctrl Pts',(-43.4753311640868,40.8750000013656,104.958734125));
#5480=CARTESIAN_POINT('Ctrl Pts',(-74.2170326445434,40.8125000013656,74.2170326445434));
#5481=CARTESIAN_POINT('Ctrl Pts',(-104.958734125,40.7500000013656,43.4753311640869));
#5482=CARTESIAN_POINT('Ctrl Pts',(-104.958734125,40.6875000013656,0.));
#5483=CARTESIAN_POINT('Ctrl Pts',(-104.958734125,40.6250000013656,-43.4753311640868));
#5484=CARTESIAN_POINT('Ctrl Pts',(-74.2170326445434,40.5625000013656,-74.2170326445434));
#5485=CARTESIAN_POINT('Ctrl Pts',(-43.4753311640868,40.5000000013656,-104.958734125));
#5486=CARTESIAN_POINT('Ctrl Pts',(-6.42686888943697E-15,40.4375000013656,
-104.958734125));
#5487=CARTESIAN_POINT('Ctrl Pts',(43.4753311640868,40.3750000013656,-104.958734125));
#5488=CARTESIAN_POINT('Ctrl Pts',(74.2170326445434,40.3125000013656,-74.2170326445434));
#5489=CARTESIAN_POINT('Ctrl Pts',(104.958734125,40.2500000013656,-43.4753311640868));
#5490=CARTESIAN_POINT('Ctrl Pts',(104.958734125,40.1875000013656,-1.28537377788739E-14));
#5491=CARTESIAN_POINT('Origin',(-7.105427357601E-14,49.5625000013656,-6.0924204042587E-14));
#5492=CARTESIAN_POINT('',(104.958734125,42.1875000013656,-6.0924204042587E-14));
#5493=CARTESIAN_POINT('',(104.958734125,41.9375000013656,-6.0924204042587E-14));
#5494=CARTESIAN_POINT('',(104.958734125,49.5625000013656,-1.089946703063E-13));
#5495=CARTESIAN_POINT('Ctrl Pts',(104.958734125,41.9375000013656,-1.28537377788739E-14));
#5496=CARTESIAN_POINT('Ctrl Pts',(104.958734125,41.8750000013656,43.4753311640868));
#5497=CARTESIAN_POINT('Ctrl Pts',(74.2170326445434,41.8125000013656,74.2170326445434));
#5498=CARTESIAN_POINT('Ctrl Pts',(43.4753311640869,41.7500000013656,104.958734125));
#5499=CARTESIAN_POINT('Ctrl Pts',(1.92806066683109E-14,41.6875000013656,
104.958734125));
#5500=CARTESIAN_POINT('Ctrl Pts',(-43.4753311640868,41.6250000013656,104.958734125));
#5501=CARTESIAN_POINT('Ctrl Pts',(-74.2170326445434,41.5625000013656,74.2170326445434));
#5502=CARTESIAN_POINT('Ctrl Pts',(-104.958734125,41.5000000013656,43.4753311640869));
#5503=CARTESIAN_POINT('Ctrl Pts',(-104.958734125,41.4375000013656,0.));
#5504=CARTESIAN_POINT('Ctrl Pts',(-104.958734125,41.3750000013656,-43.4753311640868));
#5505=CARTESIAN_POINT('Ctrl Pts',(-74.2170326445434,41.3125000013656,-74.2170326445434));
#5506=CARTESIAN_POINT('Ctrl Pts',(-43.4753311640868,41.2500000013656,-104.958734125));
#5507=CARTESIAN_POINT('Ctrl Pts',(-6.42686888943697E-15,41.1875000013656,
-104.958734125));
#5508=CARTESIAN_POINT('Ctrl Pts',(43.4753311640868,41.1250000013656,-104.958734125));
#5509=CARTESIAN_POINT('Ctrl Pts',(74.2170326445434,41.0625000013656,-74.2170326445434));
#5510=CARTESIAN_POINT('Ctrl Pts',(104.958734125,41.0000000013656,-43.4753311640868));
#5511=CARTESIAN_POINT('Ctrl Pts',(104.958734125,40.9375000013656,-1.28537377788739E-14));
#5512=CARTESIAN_POINT('Ctrl Pts',(104.958734125,42.1875000013656,-1.28537377788739E-14));
#5513=CARTESIAN_POINT('Ctrl Pts',(104.958734125,42.1250000013656,43.4753311640868));
#5514=CARTESIAN_POINT('Ctrl Pts',(74.2170326445434,42.0625000013656,74.2170326445434));
#5515=CARTESIAN_POINT('Ctrl Pts',(43.4753311640869,42.0000000013656,104.958734125));
#5516=CARTESIAN_POINT('Ctrl Pts',(1.92806066683109E-14,41.9375000013656,
104.958734125));
#5517=CARTESIAN_POINT('Ctrl Pts',(-43.4753311640868,41.8750000013656,104.958734125));
#5518=CARTESIAN_POINT('Ctrl Pts',(-74.2170326445434,41.8125000013656,74.2170326445434));
#5519=CARTESIAN_POINT('Ctrl Pts',(-104.958734125,41.7500000013656,43.4753311640869));
#5520=CARTESIAN_POINT('Ctrl Pts',(-104.958734125,41.6875000013656,0.));
#5521=CARTESIAN_POINT('Ctrl Pts',(-104.958734125,41.6250000013656,-43.4753311640868));
#5522=CARTESIAN_POINT('Ctrl Pts',(-74.2170326445434,41.5625000013656,-74.2170326445434));
#5523=CARTESIAN_POINT('Ctrl Pts',(-43.4753311640868,41.5000000013656,-104.958734125));
#5524=CARTESIAN_POINT('Ctrl Pts',(-6.42686888943697E-15,41.4375000013656,
-104.958734125));
#5525=CARTESIAN_POINT('Ctrl Pts',(43.4753311640868,41.3750000013656,-104.958734125));
#5526=CARTESIAN_POINT('Ctrl Pts',(74.2170326445434,41.3125000013656,-74.2170326445434));
#5527=CARTESIAN_POINT('Ctrl Pts',(104.958734125,41.2500000013656,-43.4753311640868));
#5528=CARTESIAN_POINT('Ctrl Pts',(104.958734125,41.1875000013656,-1.28537377788739E-14));
#5529=CARTESIAN_POINT('Origin',(-7.105427357601E-14,49.5625000013656,-6.0924204042587E-14));
#5530=CARTESIAN_POINT('',(104.958734125,43.1875000013656,-6.0924204042587E-14));
#5531=CARTESIAN_POINT('',(104.958734125,42.9375000013656,-6.0924204042587E-14));
#5532=CARTESIAN_POINT('',(104.958734125,49.5625000013656,-1.089946703063E-13));
#5533=CARTESIAN_POINT('Ctrl Pts',(104.958734125,42.9375000013656,-1.28537377788739E-14));
#5534=CARTESIAN_POINT('Ctrl Pts',(104.958734125,42.8750000013656,43.4753311640868));
#5535=CARTESIAN_POINT('Ctrl Pts',(74.2170326445434,42.8125000013656,74.2170326445434));
#5536=CARTESIAN_POINT('Ctrl Pts',(43.4753311640869,42.7500000013656,104.958734125));
#5537=CARTESIAN_POINT('Ctrl Pts',(1.92806066683109E-14,42.6875000013656,
104.958734125));
#5538=CARTESIAN_POINT('Ctrl Pts',(-43.4753311640868,42.6250000013656,104.958734125));
#5539=CARTESIAN_POINT('Ctrl Pts',(-74.2170326445434,42.5625000013656,74.2170326445434));
#5540=CARTESIAN_POINT('Ctrl Pts',(-104.958734125,42.5000000013656,43.4753311640869));
#5541=CARTESIAN_POINT('Ctrl Pts',(-104.958734125,42.4375000013656,0.));
#5542=CARTESIAN_POINT('Ctrl Pts',(-104.958734125,42.3750000013656,-43.4753311640868));
#5543=CARTESIAN_POINT('Ctrl Pts',(-74.2170326445434,42.3125000013656,-74.2170326445434));
#5544=CARTESIAN_POINT('Ctrl Pts',(-43.4753311640868,42.2500000013656,-104.958734125));
#5545=CARTESIAN_POINT('Ctrl Pts',(-6.42686888943697E-15,42.1875000013656,
-104.958734125));
#5546=CARTESIAN_POINT('Ctrl Pts',(43.4753311640868,42.1250000013656,-104.958734125));
#5547=CARTESIAN_POINT('Ctrl Pts',(74.2170326445434,42.0625000013656,-74.2170326445434));
#5548=CARTESIAN_POINT('Ctrl Pts',(104.958734125,42.0000000013656,-43.4753311640868));
#5549=CARTESIAN_POINT('Ctrl Pts',(104.958734125,41.9375000013656,-1.28537377788739E-14));
#5550=CARTESIAN_POINT('Ctrl Pts',(104.958734125,43.1875000013656,-1.28537377788739E-14));
#5551=CARTESIAN_POINT('Ctrl Pts',(104.958734125,43.1250000013656,43.4753311640868));
#5552=CARTESIAN_POINT('Ctrl Pts',(74.2170326445434,43.0625000013656,74.2170326445434));
#5553=CARTESIAN_POINT('Ctrl Pts',(43.4753311640869,43.0000000013656,104.958734125));
#5554=CARTESIAN_POINT('Ctrl Pts',(1.92806066683109E-14,42.9375000013656,
104.958734125));
#5555=CARTESIAN_POINT('Ctrl Pts',(-43.4753311640868,42.8750000013656,104.958734125));
#5556=CARTESIAN_POINT('Ctrl Pts',(-74.2170326445434,42.8125000013656,74.2170326445434));
#5557=CARTESIAN_POINT('Ctrl Pts',(-104.958734125,42.7500000013656,43.4753311640869));
#5558=CARTESIAN_POINT('Ctrl Pts',(-104.958734125,42.6875000013656,0.));
#5559=CARTESIAN_POINT('Ctrl Pts',(-104.958734125,42.6250000013656,-43.4753311640868));
#5560=CARTESIAN_POINT('Ctrl Pts',(-74.2170326445434,42.5625000013656,-74.2170326445434));
#5561=CARTESIAN_POINT('Ctrl Pts',(-43.4753311640868,42.5000000013656,-104.958734125));
#5562=CARTESIAN_POINT('Ctrl Pts',(-6.42686888943697E-15,42.4375000013656,
-104.958734125));
#5563=CARTESIAN_POINT('Ctrl Pts',(43.4753311640868,42.3750000013656,-104.958734125));
#5564=CARTESIAN_POINT('Ctrl Pts',(74.2170326445434,42.3125000013656,-74.2170326445434));
#5565=CARTESIAN_POINT('Ctrl Pts',(104.958734125,42.2500000013656,-43.4753311640868));
#5566=CARTESIAN_POINT('Ctrl Pts',(104.958734125,42.1875000013656,-1.28537377788739E-14));
#5567=CARTESIAN_POINT('Origin',(-7.105427357601E-14,49.5625000013656,-6.0924204042587E-14));
#5568=CARTESIAN_POINT('',(104.958734125,44.1875000013656,-6.0924204042587E-14));
#5569=CARTESIAN_POINT('',(104.958734125,43.9375000013656,-6.0924204042587E-14));
#5570=CARTESIAN_POINT('',(104.958734125,49.5625000013656,-1.089946703063E-13));
#5571=CARTESIAN_POINT('Ctrl Pts',(104.958734125,43.9375000013656,-1.28537377788739E-14));
#5572=CARTESIAN_POINT('Ctrl Pts',(104.958734125,43.8750000013656,43.4753311640868));
#5573=CARTESIAN_POINT('Ctrl Pts',(74.2170326445434,43.8125000013656,74.2170326445434));
#5574=CARTESIAN_POINT('Ctrl Pts',(43.4753311640869,43.7500000013656,104.958734125));
#5575=CARTESIAN_POINT('Ctrl Pts',(1.92806066683109E-14,43.6875000013656,
104.958734125));
#5576=CARTESIAN_POINT('Ctrl Pts',(-43.4753311640868,43.6250000013656,104.958734125));
#5577=CARTESIAN_POINT('Ctrl Pts',(-74.2170326445434,43.5625000013656,74.2170326445434));
#5578=CARTESIAN_POINT('Ctrl Pts',(-104.958734125,43.5000000013656,43.4753311640869));
#5579=CARTESIAN_POINT('Ctrl Pts',(-104.958734125,43.4375000013656,0.));
#5580=CARTESIAN_POINT('Ctrl Pts',(-104.958734125,43.3750000013656,-43.4753311640868));
#5581=CARTESIAN_POINT('Ctrl Pts',(-74.2170326445434,43.3125000013656,-74.2170326445434));
#5582=CARTESIAN_POINT('Ctrl Pts',(-43.4753311640868,43.2500000013656,-104.958734125));
#5583=CARTESIAN_POINT('Ctrl Pts',(-6.42686888943697E-15,43.1875000013656,
-104.958734125));
#5584=CARTESIAN_POINT('Ctrl Pts',(43.4753311640868,43.1250000013656,-104.958734125));
#5585=CARTESIAN_POINT('Ctrl Pts',(74.2170326445434,43.0625000013656,-74.2170326445434));
#5586=CARTESIAN_POINT('Ctrl Pts',(104.958734125,43.0000000013656,-43.4753311640868));
#5587=CARTESIAN_POINT('Ctrl Pts',(104.958734125,42.9375000013656,-1.28537377788739E-14));
#5588=CARTESIAN_POINT('Ctrl Pts',(104.958734125,44.1875000013656,-1.28537377788739E-14));
#5589=CARTESIAN_POINT('Ctrl Pts',(104.958734125,44.1250000013656,43.4753311640868));
#5590=CARTESIAN_POINT('Ctrl Pts',(74.2170326445434,44.0625000013656,74.2170326445434));
#5591=CARTESIAN_POINT('Ctrl Pts',(43.4753311640869,44.0000000013656,104.958734125));
#5592=CARTESIAN_POINT('Ctrl Pts',(1.92806066683109E-14,43.9375000013656,
104.958734125));
#5593=CARTESIAN_POINT('Ctrl Pts',(-43.4753311640868,43.8750000013656,104.958734125));
#5594=CARTESIAN_POINT('Ctrl Pts',(-74.2170326445434,43.8125000013656,74.2170326445434));
#5595=CARTESIAN_POINT('Ctrl Pts',(-104.958734125,43.7500000013656,43.4753311640869));
#5596=CARTESIAN_POINT('Ctrl Pts',(-104.958734125,43.6875000013656,0.));
#5597=CARTESIAN_POINT('Ctrl Pts',(-104.958734125,43.6250000013656,-43.4753311640868));
#5598=CARTESIAN_POINT('Ctrl Pts',(-74.2170326445434,43.5625000013656,-74.2170326445434));
#5599=CARTESIAN_POINT('Ctrl Pts',(-43.4753311640868,43.5000000013656,-104.958734125));
#5600=CARTESIAN_POINT('Ctrl Pts',(-6.42686888943697E-15,43.4375000013656,
-104.958734125));
#5601=CARTESIAN_POINT('Ctrl Pts',(43.4753311640868,43.3750000013656,-104.958734125));
#5602=CARTESIAN_POINT('Ctrl Pts',(74.2170326445434,43.3125000013656,-74.2170326445434));
#5603=CARTESIAN_POINT('Ctrl Pts',(104.958734125,43.2500000013656,-43.4753311640868));
#5604=CARTESIAN_POINT('Ctrl Pts',(104.958734125,43.1875000013656,-1.28537377788739E-14));
#5605=CARTESIAN_POINT('Origin',(-7.105427357601E-14,49.5625000013656,-6.0924204042587E-14));
#5606=CARTESIAN_POINT('',(104.958734125,45.1875000013656,-6.0924204042587E-14));
#5607=CARTESIAN_POINT('',(104.958734125,44.9375000013656,-6.0924204042587E-14));
#5608=CARTESIAN_POINT('',(104.958734125,49.5625000013656,-1.089946703063E-13));
#5609=CARTESIAN_POINT('Ctrl Pts',(104.958734125,44.9375000013656,-1.28537377788739E-14));
#5610=CARTESIAN_POINT('Ctrl Pts',(104.958734125,44.8750000013656,43.4753311640868));
#5611=CARTESIAN_POINT('Ctrl Pts',(74.2170326445434,44.8125000013656,74.2170326445434));
#5612=CARTESIAN_POINT('Ctrl Pts',(43.4753311640869,44.7500000013656,104.958734125));
#5613=CARTESIAN_POINT('Ctrl Pts',(1.92806066683109E-14,44.6875000013656,
104.958734125));
#5614=CARTESIAN_POINT('Ctrl Pts',(-43.4753311640868,44.6250000013656,104.958734125));
#5615=CARTESIAN_POINT('Ctrl Pts',(-74.2170326445434,44.5625000013656,74.2170326445434));
#5616=CARTESIAN_POINT('Ctrl Pts',(-104.958734125,44.5000000013656,43.4753311640869));
#5617=CARTESIAN_POINT('Ctrl Pts',(-104.958734125,44.4375000013656,0.));
#5618=CARTESIAN_POINT('Ctrl Pts',(-104.958734125,44.3750000013656,-43.4753311640868));
#5619=CARTESIAN_POINT('Ctrl Pts',(-74.2170326445434,44.3125000013656,-74.2170326445434));
#5620=CARTESIAN_POINT('Ctrl Pts',(-43.4753311640868,44.2500000013656,-104.958734125));
#5621=CARTESIAN_POINT('Ctrl Pts',(-6.42686888943697E-15,44.1875000013656,
-104.958734125));
#5622=CARTESIAN_POINT('Ctrl Pts',(43.4753311640868,44.1250000013656,-104.958734125));
#5623=CARTESIAN_POINT('Ctrl Pts',(74.2170326445434,44.0625000013656,-74.2170326445434));
#5624=CARTESIAN_POINT('Ctrl Pts',(104.958734125,44.0000000013656,-43.4753311640868));
#5625=CARTESIAN_POINT('Ctrl Pts',(104.958734125,43.9375000013656,-1.28537377788739E-14));
#5626=CARTESIAN_POINT('Ctrl Pts',(104.958734125,45.1875000013656,-1.28537377788739E-14));
#5627=CARTESIAN_POINT('Ctrl Pts',(104.958734125,45.1250000013656,43.4753311640868));
#5628=CARTESIAN_POINT('Ctrl Pts',(74.2170326445434,45.0625000013656,74.2170326445434));
#5629=CARTESIAN_POINT('Ctrl Pts',(43.4753311640869,45.0000000013656,104.958734125));
#5630=CARTESIAN_POINT('Ctrl Pts',(1.92806066683109E-14,44.9375000013656,
104.958734125));
#5631=CARTESIAN_POINT('Ctrl Pts',(-43.4753311640868,44.8750000013656,104.958734125));
#5632=CARTESIAN_POINT('Ctrl Pts',(-74.2170326445434,44.8125000013656,74.2170326445434));
#5633=CARTESIAN_POINT('Ctrl Pts',(-104.958734125,44.7500000013656,43.4753311640869));
#5634=CARTESIAN_POINT('Ctrl Pts',(-104.958734125,44.6875000013656,0.));
#5635=CARTESIAN_POINT('Ctrl Pts',(-104.958734125,44.6250000013656,-43.4753311640868));
#5636=CARTESIAN_POINT('Ctrl Pts',(-74.2170326445434,44.5625000013656,-74.2170326445434));
#5637=CARTESIAN_POINT('Ctrl Pts',(-43.4753311640868,44.5000000013656,-104.958734125));
#5638=CARTESIAN_POINT('Ctrl Pts',(-6.42686888943697E-15,44.4375000013656,
-104.958734125));
#5639=CARTESIAN_POINT('Ctrl Pts',(43.4753311640868,44.3750000013656,-104.958734125));
#5640=CARTESIAN_POINT('Ctrl Pts',(74.2170326445434,44.3125000013656,-74.2170326445434));
#5641=CARTESIAN_POINT('Ctrl Pts',(104.958734125,44.2500000013656,-43.4753311640868));
#5642=CARTESIAN_POINT('Ctrl Pts',(104.958734125,44.1875000013656,-1.28537377788739E-14));
#5643=CARTESIAN_POINT('Origin',(-7.105427357601E-14,49.5625000013656,-6.0924204042587E-14));
#5644=CARTESIAN_POINT('',(104.958734125,46.1875000013656,-6.0924204042587E-14));
#5645=CARTESIAN_POINT('',(104.958734125,45.9375000013656,-6.0924204042587E-14));
#5646=CARTESIAN_POINT('',(104.958734125,49.5625000013656,-1.089946703063E-13));
#5647=CARTESIAN_POINT('Ctrl Pts',(104.958734125,45.9375000013656,-1.28537377788739E-14));
#5648=CARTESIAN_POINT('Ctrl Pts',(104.958734125,45.8750000013656,43.4753311640868));
#5649=CARTESIAN_POINT('Ctrl Pts',(74.2170326445434,45.8125000013656,74.2170326445434));
#5650=CARTESIAN_POINT('Ctrl Pts',(43.4753311640869,45.7500000013656,104.958734125));
#5651=CARTESIAN_POINT('Ctrl Pts',(1.92806066683109E-14,45.6875000013656,
104.958734125));
#5652=CARTESIAN_POINT('Ctrl Pts',(-43.4753311640868,45.6250000013656,104.958734125));
#5653=CARTESIAN_POINT('Ctrl Pts',(-74.2170326445434,45.5625000013656,74.2170326445434));
#5654=CARTESIAN_POINT('Ctrl Pts',(-104.958734125,45.5000000013656,43.4753311640869));
#5655=CARTESIAN_POINT('Ctrl Pts',(-104.958734125,45.4375000013656,0.));
#5656=CARTESIAN_POINT('Ctrl Pts',(-104.958734125,45.3750000013656,-43.4753311640868));
#5657=CARTESIAN_POINT('Ctrl Pts',(-74.2170326445434,45.3125000013656,-74.2170326445434));
#5658=CARTESIAN_POINT('Ctrl Pts',(-43.4753311640868,45.2500000013656,-104.958734125));
#5659=CARTESIAN_POINT('Ctrl Pts',(-6.42686888943697E-15,45.1875000013656,
-104.958734125));
#5660=CARTESIAN_POINT('Ctrl Pts',(43.4753311640868,45.1250000013656,-104.958734125));
#5661=CARTESIAN_POINT('Ctrl Pts',(74.2170326445434,45.0625000013656,-74.2170326445434));
#5662=CARTESIAN_POINT('Ctrl Pts',(104.958734125,45.0000000013656,-43.4753311640868));
#5663=CARTESIAN_POINT('Ctrl Pts',(104.958734125,44.9375000013656,-1.28537377788739E-14));
#5664=CARTESIAN_POINT('Ctrl Pts',(104.958734125,46.1875000013656,-1.28537377788739E-14));
#5665=CARTESIAN_POINT('Ctrl Pts',(104.958734125,46.1250000013656,43.4753311640868));
#5666=CARTESIAN_POINT('Ctrl Pts',(74.2170326445434,46.0625000013656,74.2170326445434));
#5667=CARTESIAN_POINT('Ctrl Pts',(43.4753311640869,46.0000000013656,104.958734125));
#5668=CARTESIAN_POINT('Ctrl Pts',(1.92806066683109E-14,45.9375000013656,
104.958734125));
#5669=CARTESIAN_POINT('Ctrl Pts',(-43.4753311640868,45.8750000013656,104.958734125));
#5670=CARTESIAN_POINT('Ctrl Pts',(-74.2170326445434,45.8125000013656,74.2170326445434));
#5671=CARTESIAN_POINT('Ctrl Pts',(-104.958734125,45.7500000013656,43.4753311640869));
#5672=CARTESIAN_POINT('Ctrl Pts',(-104.958734125,45.6875000013656,0.));
#5673=CARTESIAN_POINT('Ctrl Pts',(-104.958734125,45.6250000013656,-43.4753311640868));
#5674=CARTESIAN_POINT('Ctrl Pts',(-74.2170326445434,45.5625000013656,-74.2170326445434));
#5675=CARTESIAN_POINT('Ctrl Pts',(-43.4753311640868,45.5000000013656,-104.958734125));
#5676=CARTESIAN_POINT('Ctrl Pts',(-6.42686888943697E-15,45.4375000013656,
-104.958734125));
#5677=CARTESIAN_POINT('Ctrl Pts',(43.4753311640868,45.3750000013656,-104.958734125));
#5678=CARTESIAN_POINT('Ctrl Pts',(74.2170326445434,45.3125000013656,-74.2170326445434));
#5679=CARTESIAN_POINT('Ctrl Pts',(104.958734125,45.2500000013656,-43.4753311640868));
#5680=CARTESIAN_POINT('Ctrl Pts',(104.958734125,45.1875000013656,-1.28537377788739E-14));
#5681=CARTESIAN_POINT('Origin',(-7.105427357601E-14,49.5625000013656,-6.0924204042587E-14));
#5682=CARTESIAN_POINT('',(104.958734125,47.1875000013656,-6.0924204042587E-14));
#5683=CARTESIAN_POINT('',(104.958734125,46.9375000013656,-6.0924204042587E-14));
#5684=CARTESIAN_POINT('',(104.958734125,49.5625000013656,-1.089946703063E-13));
#5685=CARTESIAN_POINT('Ctrl Pts',(104.958734125,46.9375000013656,-1.28537377788739E-14));
#5686=CARTESIAN_POINT('Ctrl Pts',(104.958734125,46.8750000013656,43.4753311640868));
#5687=CARTESIAN_POINT('Ctrl Pts',(74.2170326445434,46.8125000013656,74.2170326445434));
#5688=CARTESIAN_POINT('Ctrl Pts',(43.4753311640869,46.7500000013656,104.958734125));
#5689=CARTESIAN_POINT('Ctrl Pts',(1.92806066683109E-14,46.6875000013656,
104.958734125));
#5690=CARTESIAN_POINT('Ctrl Pts',(-43.4753311640868,46.6250000013656,104.958734125));
#5691=CARTESIAN_POINT('Ctrl Pts',(-74.2170326445434,46.5625000013656,74.2170326445434));
#5692=CARTESIAN_POINT('Ctrl Pts',(-104.958734125,46.5000000013656,43.4753311640869));
#5693=CARTESIAN_POINT('Ctrl Pts',(-104.958734125,46.4375000013656,0.));
#5694=CARTESIAN_POINT('Ctrl Pts',(-104.958734125,46.3750000013656,-43.4753311640868));
#5695=CARTESIAN_POINT('Ctrl Pts',(-74.2170326445434,46.3125000013656,-74.2170326445434));
#5696=CARTESIAN_POINT('Ctrl Pts',(-43.4753311640868,46.2500000013656,-104.958734125));
#5697=CARTESIAN_POINT('Ctrl Pts',(-6.42686888943697E-15,46.1875000013656,
-104.958734125));
#5698=CARTESIAN_POINT('Ctrl Pts',(43.4753311640868,46.1250000013656,-104.958734125));
#5699=CARTESIAN_POINT('Ctrl Pts',(74.2170326445434,46.0625000013656,-74.2170326445434));
#5700=CARTESIAN_POINT('Ctrl Pts',(104.958734125,46.0000000013656,-43.4753311640868));
#5701=CARTESIAN_POINT('Ctrl Pts',(104.958734125,45.9375000013656,-1.28537377788739E-14));
#5702=CARTESIAN_POINT('Ctrl Pts',(104.958734125,47.1875000013656,-1.28537377788739E-14));
#5703=CARTESIAN_POINT('Ctrl Pts',(104.958734125,47.1250000013656,43.4753311640868));
#5704=CARTESIAN_POINT('Ctrl Pts',(74.2170326445434,47.0625000013656,74.2170326445434));
#5705=CARTESIAN_POINT('Ctrl Pts',(43.4753311640869,47.0000000013656,104.958734125));
#5706=CARTESIAN_POINT('Ctrl Pts',(1.92806066683109E-14,46.9375000013656,
104.958734125));
#5707=CARTESIAN_POINT('Ctrl Pts',(-43.4753311640868,46.8750000013656,104.958734125));
#5708=CARTESIAN_POINT('Ctrl Pts',(-74.2170326445434,46.8125000013656,74.2170326445434));
#5709=CARTESIAN_POINT('Ctrl Pts',(-104.958734125,46.7500000013656,43.4753311640869));
#5710=CARTESIAN_POINT('Ctrl Pts',(-104.958734125,46.6875000013656,0.));
#5711=CARTESIAN_POINT('Ctrl Pts',(-104.958734125,46.6250000013656,-43.4753311640868));
#5712=CARTESIAN_POINT('Ctrl Pts',(-74.2170326445434,46.5625000013656,-74.2170326445434));
#5713=CARTESIAN_POINT('Ctrl Pts',(-43.4753311640868,46.5000000013656,-104.958734125));
#5714=CARTESIAN_POINT('Ctrl Pts',(-6.42686888943697E-15,46.4375000013656,
-104.958734125));
#5715=CARTESIAN_POINT('Ctrl Pts',(43.4753311640868,46.3750000013656,-104.958734125));
#5716=CARTESIAN_POINT('Ctrl Pts',(74.2170326445434,46.3125000013656,-74.2170326445434));
#5717=CARTESIAN_POINT('Ctrl Pts',(104.958734125,46.2500000013656,-43.4753311640868));
#5718=CARTESIAN_POINT('Ctrl Pts',(104.958734125,46.1875000013656,-1.28537377788739E-14));
#5719=CARTESIAN_POINT('Origin',(-7.105427357601E-14,49.5625000013656,-6.0924204042587E-14));
#5720=CARTESIAN_POINT('',(104.958734125,48.1875000013656,-6.0924204042587E-14));
#5721=CARTESIAN_POINT('',(104.958734125,47.9375000013656,-6.0924204042587E-14));
#5722=CARTESIAN_POINT('',(104.958734125,49.5625000013656,-1.089946703063E-13));
#5723=CARTESIAN_POINT('Ctrl Pts',(104.958734125,47.9375000013656,-1.28537377788739E-14));
#5724=CARTESIAN_POINT('Ctrl Pts',(104.958734125,47.8750000013656,43.4753311640868));
#5725=CARTESIAN_POINT('Ctrl Pts',(74.2170326445434,47.8125000013656,74.2170326445434));
#5726=CARTESIAN_POINT('Ctrl Pts',(43.4753311640869,47.7500000013656,104.958734125));
#5727=CARTESIAN_POINT('Ctrl Pts',(1.92806066683109E-14,47.6875000013656,
104.958734125));
#5728=CARTESIAN_POINT('Ctrl Pts',(-43.4753311640868,47.6250000013656,104.958734125));
#5729=CARTESIAN_POINT('Ctrl Pts',(-74.2170326445434,47.5625000013656,74.2170326445434));
#5730=CARTESIAN_POINT('Ctrl Pts',(-104.958734125,47.5000000013656,43.4753311640869));
#5731=CARTESIAN_POINT('Ctrl Pts',(-104.958734125,47.4375000013656,0.));
#5732=CARTESIAN_POINT('Ctrl Pts',(-104.958734125,47.3750000013656,-43.4753311640868));
#5733=CARTESIAN_POINT('Ctrl Pts',(-74.2170326445434,47.3125000013656,-74.2170326445434));
#5734=CARTESIAN_POINT('Ctrl Pts',(-43.4753311640868,47.2500000013656,-104.958734125));
#5735=CARTESIAN_POINT('Ctrl Pts',(-6.42686888943697E-15,47.1875000013656,
-104.958734125));
#5736=CARTESIAN_POINT('Ctrl Pts',(43.4753311640868,47.1250000013656,-104.958734125));
#5737=CARTESIAN_POINT('Ctrl Pts',(74.2170326445434,47.0625000013656,-74.2170326445434));
#5738=CARTESIAN_POINT('Ctrl Pts',(104.958734125,47.0000000013656,-43.4753311640868));
#5739=CARTESIAN_POINT('Ctrl Pts',(104.958734125,46.9375000013656,-1.28537377788739E-14));
#5740=CARTESIAN_POINT('Ctrl Pts',(104.958734125,48.1875000013656,-1.28537377788739E-14));
#5741=CARTESIAN_POINT('Ctrl Pts',(104.958734125,48.1250000013656,43.4753311640868));
#5742=CARTESIAN_POINT('Ctrl Pts',(74.2170326445434,48.0625000013656,74.2170326445434));
#5743=CARTESIAN_POINT('Ctrl Pts',(43.4753311640869,48.0000000013656,104.958734125));
#5744=CARTESIAN_POINT('Ctrl Pts',(1.92806066683109E-14,47.9375000013656,
104.958734125));
#5745=CARTESIAN_POINT('Ctrl Pts',(-43.4753311640868,47.8750000013656,104.958734125));
#5746=CARTESIAN_POINT('Ctrl Pts',(-74.2170326445434,47.8125000013656,74.2170326445434));
#5747=CARTESIAN_POINT('Ctrl Pts',(-104.958734125,47.7500000013656,43.4753311640869));
#5748=CARTESIAN_POINT('Ctrl Pts',(-104.958734125,47.6875000013656,0.));
#5749=CARTESIAN_POINT('Ctrl Pts',(-104.958734125,47.6250000013656,-43.4753311640868));
#5750=CARTESIAN_POINT('Ctrl Pts',(-74.2170326445434,47.5625000013656,-74.2170326445434));
#5751=CARTESIAN_POINT('Ctrl Pts',(-43.4753311640868,47.5000000013656,-104.958734125));
#5752=CARTESIAN_POINT('Ctrl Pts',(-6.42686888943697E-15,47.4375000013656,
-104.958734125));
#5753=CARTESIAN_POINT('Ctrl Pts',(43.4753311640868,47.3750000013656,-104.958734125));
#5754=CARTESIAN_POINT('Ctrl Pts',(74.2170326445434,47.3125000013656,-74.2170326445434));
#5755=CARTESIAN_POINT('Ctrl Pts',(104.958734125,47.2500000013656,-43.4753311640868));
#5756=CARTESIAN_POINT('Ctrl Pts',(104.958734125,47.1875000013656,-1.28537377788739E-14));
#5757=CARTESIAN_POINT('Origin',(-7.105427357601E-14,49.5625000013656,-6.0924204042587E-14));
#5758=CARTESIAN_POINT('',(104.958734125,49.1875000013656,-6.0924204042587E-14));
#5759=CARTESIAN_POINT('',(104.958734125,48.9375000013656,-6.0924204042587E-14));
#5760=CARTESIAN_POINT('',(104.958734125,49.5625000013656,-1.089946703063E-13));
#5761=CARTESIAN_POINT('',(-104.958734125,49.6875000013656,0.));
#5762=CARTESIAN_POINT('Ctrl Pts',(-104.958734125,49.6875000013656,0.));
#5763=CARTESIAN_POINT('Ctrl Pts',(-104.958734125,49.6250000013656,-43.4753311640868));
#5764=CARTESIAN_POINT('Ctrl Pts',(-74.2170326445434,49.5625000013656,-74.2170326445434));
#5765=CARTESIAN_POINT('Ctrl Pts',(-43.4753311640868,49.5000000013656,-104.958734125));
#5766=CARTESIAN_POINT('Ctrl Pts',(-6.42686888943697E-15,49.4375000013656,
-104.958734125));
#5767=CARTESIAN_POINT('Ctrl Pts',(43.4753311640868,49.3750000013656,-104.958734125));
#5768=CARTESIAN_POINT('Ctrl Pts',(74.2170326445434,49.3125000013656,-74.2170326445434));
#5769=CARTESIAN_POINT('Ctrl Pts',(104.958734125,49.2500000013656,-43.4753311640868));
#5770=CARTESIAN_POINT('Ctrl Pts',(104.958734125,49.1875000013656,-1.28537377788739E-14));
#5771=CARTESIAN_POINT('',(-104.958734125,49.4375000013656,0.));
#5772=CARTESIAN_POINT('',(-104.958734125,49.4375000013656,0.));
#5773=CARTESIAN_POINT('Ctrl Pts',(-104.958734125,49.4375000013656,0.));
#5774=CARTESIAN_POINT('Ctrl Pts',(-104.958734125,49.3750000013656,-43.4753311640868));
#5775=CARTESIAN_POINT('Ctrl Pts',(-74.2170326445434,49.3125000013656,-74.2170326445434));
#5776=CARTESIAN_POINT('Ctrl Pts',(-43.4753311640868,49.2500000013656,-104.958734125));
#5777=CARTESIAN_POINT('Ctrl Pts',(-6.42686888943697E-15,49.1875000013656,
-104.958734125));
#5778=CARTESIAN_POINT('Ctrl Pts',(43.4753311640868,49.1250000013656,-104.958734125));
#5779=CARTESIAN_POINT('Ctrl Pts',(74.2170326445434,49.0625000013656,-74.2170326445434));
#5780=CARTESIAN_POINT('Ctrl Pts',(104.958734125,49.0000000013656,-43.4753311640868));
#5781=CARTESIAN_POINT('Ctrl Pts',(104.958734125,48.9375000013656,-1.28537377788739E-14));
#5782=CARTESIAN_POINT('Origin',(0.,105.,0.));
#5783=CARTESIAN_POINT('',(3.23000593275114E-15,0.375000002731177,105.5));
#5784=CARTESIAN_POINT('',(3.23000593275114E-15,0.249999999999986,105.5));
#5785=CARTESIAN_POINT('',(-1.29200237310046E-14,105.,105.5));
#5786=CARTESIAN_POINT('',(-105.5,0.,0.));
#5787=CARTESIAN_POINT('Ctrl Pts',(1.93800355965069E-14,0.249999999999986,
105.5));
#5788=CARTESIAN_POINT('Ctrl Pts',(-43.6995308303616,0.187499999999986,105.5));
#5789=CARTESIAN_POINT('Ctrl Pts',(-74.5997654151808,0.124999999999986,74.5997654151808));
#5790=CARTESIAN_POINT('Ctrl Pts',(-105.5,0.0624999999999862,43.6995308303616));
#5791=CARTESIAN_POINT('Ctrl Pts',(-105.5,-1.38777878078145E-14,0.));
#5792=CARTESIAN_POINT('',(-74.5997640648779,1.90551595483966E-15,-74.5997667654837));
#5793=CARTESIAN_POINT('Origin',(0.,0.,0.));
#5794=CARTESIAN_POINT('Ctrl Pts',(1.93800355965069E-14,0.375000002731177,
105.5));
#5795=CARTESIAN_POINT('Ctrl Pts',(-43.6995308303616,0.312500002731177,105.5));
#5796=CARTESIAN_POINT('Ctrl Pts',(-74.5997654151808,0.250000002731177,74.5997654151808));
#5797=CARTESIAN_POINT('Ctrl Pts',(-105.5,0.187500002731177,43.6995308303616));
#5798=CARTESIAN_POINT('Ctrl Pts',(-105.5,0.125000002731177,0.));
#5799=CARTESIAN_POINT('Ctrl Pts',(-105.5,0.0625000027311765,-43.6995308303615));
#5800=CARTESIAN_POINT('Ctrl Pts',(-74.5997640648778,1.90551595467487E-15,
-74.5997667654837));
#5801=CARTESIAN_POINT('Origin',(0.,105.,0.));
#5802=CARTESIAN_POINT('',(3.23000593275114E-15,1.37500000273118,105.5));
#5803=CARTESIAN_POINT('',(3.23000593275114E-15,1.24999999999999,105.5));
#5804=CARTESIAN_POINT('',(-1.29200237310046E-14,105.,105.5));
#5805=CARTESIAN_POINT('Ctrl Pts',(1.93800355965069E-14,1.24999999999999,
105.5));
#5806=CARTESIAN_POINT('Ctrl Pts',(-43.6995308303616,1.18749999999999,105.5));
#5807=CARTESIAN_POINT('Ctrl Pts',(-74.5997654151808,1.12499999999999,74.5997654151808));
#5808=CARTESIAN_POINT('Ctrl Pts',(-105.5,1.06249999999999,43.6995308303616));
#5809=CARTESIAN_POINT('Ctrl Pts',(-105.5,0.999999999999987,0.));
#5810=CARTESIAN_POINT('Ctrl Pts',(-105.5,0.937499999999987,-43.6995308303615));
#5811=CARTESIAN_POINT('Ctrl Pts',(-74.5997654151808,0.874999999999987,-74.5997654151808));
#5812=CARTESIAN_POINT('Ctrl Pts',(-43.6995308303615,0.812499999999987,-105.5));
#5813=CARTESIAN_POINT('Ctrl Pts',(-6.46001186550229E-15,0.749999999999987,
-105.5));
#5814=CARTESIAN_POINT('Ctrl Pts',(43.6995308303615,0.687499999999987,-105.5));
#5815=CARTESIAN_POINT('Ctrl Pts',(74.5997654151808,0.624999999999987,-74.5997654151808));
#5816=CARTESIAN_POINT('Ctrl Pts',(105.5,0.562499999999987,-43.6995308303616));
#5817=CARTESIAN_POINT('Ctrl Pts',(105.5,0.499999999999987,-1.29200237310046E-14));
#5818=CARTESIAN_POINT('Ctrl Pts',(105.5,0.437499999999987,43.6995308303615));
#5819=CARTESIAN_POINT('Ctrl Pts',(74.5997654151808,0.374999999999986,74.5997654151808));
#5820=CARTESIAN_POINT('Ctrl Pts',(43.6995308303616,0.312499999999986,105.5));
#5821=CARTESIAN_POINT('Ctrl Pts',(1.93800355965069E-14,0.249999999999986,
105.5));
#5822=CARTESIAN_POINT('Ctrl Pts',(1.93800355965069E-14,1.37500000273118,
105.5));
#5823=CARTESIAN_POINT('Ctrl Pts',(-43.6995308303616,1.31250000273118,105.5));
#5824=CARTESIAN_POINT('Ctrl Pts',(-74.5997654151808,1.25000000273118,74.5997654151808));
#5825=CARTESIAN_POINT('Ctrl Pts',(-105.5,1.18750000273118,43.6995308303616));
#5826=CARTESIAN_POINT('Ctrl Pts',(-105.5,1.12500000273118,0.));
#5827=CARTESIAN_POINT('Ctrl Pts',(-105.5,1.06250000273118,-43.6995308303615));
#5828=CARTESIAN_POINT('Ctrl Pts',(-74.5997654151808,1.00000000273118,-74.5997654151808));
#5829=CARTESIAN_POINT('Ctrl Pts',(-43.6995308303615,0.937500002731177,-105.5));
#5830=CARTESIAN_POINT('Ctrl Pts',(-6.46001186550229E-15,0.875000002731177,
-105.5));
#5831=CARTESIAN_POINT('Ctrl Pts',(43.6995308303615,0.812500002731177,-105.5));
#5832=CARTESIAN_POINT('Ctrl Pts',(74.5997654151808,0.750000002731177,-74.5997654151808));
#5833=CARTESIAN_POINT('Ctrl Pts',(105.5,0.687500002731177,-43.6995308303616));
#5834=CARTESIAN_POINT('Ctrl Pts',(105.5,0.625000002731177,-1.29200237310046E-14));
#5835=CARTESIAN_POINT('Ctrl Pts',(105.5,0.562500002731177,43.6995308303615));
#5836=CARTESIAN_POINT('Ctrl Pts',(74.5997654151808,0.500000002731177,74.5997654151808));
#5837=CARTESIAN_POINT('Ctrl Pts',(43.6995308303616,0.437500002731177,105.5));
#5838=CARTESIAN_POINT('Ctrl Pts',(1.93800355965069E-14,0.375000002731177,
105.5));
#5839=CARTESIAN_POINT('Origin',(0.,105.,0.));
#5840=CARTESIAN_POINT('',(3.23000593275114E-15,2.37500000273118,105.5));
#5841=CARTESIAN_POINT('',(3.23000593275114E-15,2.24999999999999,105.5));
#5842=CARTESIAN_POINT('',(-1.29200237310046E-14,105.,105.5));
#5843=CARTESIAN_POINT('Ctrl Pts',(1.93800355965069E-14,2.24999999999999,
105.5));
#5844=CARTESIAN_POINT('Ctrl Pts',(-43.6995308303616,2.18749999999999,105.5));
#5845=CARTESIAN_POINT('Ctrl Pts',(-74.5997654151808,2.12499999999999,74.5997654151808));
#5846=CARTESIAN_POINT('Ctrl Pts',(-105.5,2.06249999999999,43.6995308303616));
#5847=CARTESIAN_POINT('Ctrl Pts',(-105.5,1.99999999999999,0.));
#5848=CARTESIAN_POINT('Ctrl Pts',(-105.5,1.93749999999999,-43.6995308303615));
#5849=CARTESIAN_POINT('Ctrl Pts',(-74.5997654151808,1.87499999999999,-74.5997654151808));
#5850=CARTESIAN_POINT('Ctrl Pts',(-43.6995308303615,1.81249999999999,-105.5));
#5851=CARTESIAN_POINT('Ctrl Pts',(-6.46001186550229E-15,1.74999999999999,
-105.5));
#5852=CARTESIAN_POINT('Ctrl Pts',(43.6995308303615,1.68749999999999,-105.5));
#5853=CARTESIAN_POINT('Ctrl Pts',(74.5997654151808,1.62499999999999,-74.5997654151808));
#5854=CARTESIAN_POINT('Ctrl Pts',(105.5,1.56249999999999,-43.6995308303616));
#5855=CARTESIAN_POINT('Ctrl Pts',(105.5,1.49999999999999,-1.29200237310046E-14));
#5856=CARTESIAN_POINT('Ctrl Pts',(105.5,1.43749999999999,43.6995308303615));
#5857=CARTESIAN_POINT('Ctrl Pts',(74.5997654151808,1.37499999999999,74.5997654151808));
#5858=CARTESIAN_POINT('Ctrl Pts',(43.6995308303616,1.31249999999999,105.5));
#5859=CARTESIAN_POINT('Ctrl Pts',(1.93800355965069E-14,1.24999999999999,
105.5));
#5860=CARTESIAN_POINT('Ctrl Pts',(1.93800355965069E-14,2.37500000273118,
105.5));
#5861=CARTESIAN_POINT('Ctrl Pts',(-43.6995308303616,2.31250000273118,105.5));
#5862=CARTESIAN_POINT('Ctrl Pts',(-74.5997654151808,2.25000000273118,74.5997654151808));
#5863=CARTESIAN_POINT('Ctrl Pts',(-105.5,2.18750000273118,43.6995308303616));
#5864=CARTESIAN_POINT('Ctrl Pts',(-105.5,2.12500000273118,0.));
#5865=CARTESIAN_POINT('Ctrl Pts',(-105.5,2.06250000273118,-43.6995308303615));
#5866=CARTESIAN_POINT('Ctrl Pts',(-74.5997654151808,2.00000000273118,-74.5997654151808));
#5867=CARTESIAN_POINT('Ctrl Pts',(-43.6995308303615,1.93750000273118,-105.5));
#5868=CARTESIAN_POINT('Ctrl Pts',(-6.46001186550229E-15,1.87500000273118,
-105.5));
#5869=CARTESIAN_POINT('Ctrl Pts',(43.6995308303615,1.81250000273118,-105.5));
#5870=CARTESIAN_POINT('Ctrl Pts',(74.5997654151808,1.75000000273118,-74.5997654151808));
#5871=CARTESIAN_POINT('Ctrl Pts',(105.5,1.68750000273118,-43.6995308303616));
#5872=CARTESIAN_POINT('Ctrl Pts',(105.5,1.62500000273118,-1.29200237310046E-14));
#5873=CARTESIAN_POINT('Ctrl Pts',(105.5,1.56250000273118,43.6995308303615));
#5874=CARTESIAN_POINT('Ctrl Pts',(74.5997654151808,1.50000000273118,74.5997654151808));
#5875=CARTESIAN_POINT('Ctrl Pts',(43.6995308303616,1.43750000273118,105.5));
#5876=CARTESIAN_POINT('Ctrl Pts',(1.93800355965069E-14,1.37500000273118,
105.5));
#5877=CARTESIAN_POINT('Origin',(0.,105.,0.));
#5878=CARTESIAN_POINT('',(3.23000593275114E-15,3.37500000273118,105.5));
#5879=CARTESIAN_POINT('',(3.23000593275114E-15,3.24999999999999,105.5));
#5880=CARTESIAN_POINT('',(-1.29200237310046E-14,105.,105.5));
#5881=CARTESIAN_POINT('Ctrl Pts',(1.93800355965069E-14,3.24999999999999,
105.5));
#5882=CARTESIAN_POINT('Ctrl Pts',(-43.6995308303616,3.18749999999999,105.5));
#5883=CARTESIAN_POINT('Ctrl Pts',(-74.5997654151808,3.12499999999999,74.5997654151808));
#5884=CARTESIAN_POINT('Ctrl Pts',(-105.5,3.06249999999999,43.6995308303616));
#5885=CARTESIAN_POINT('Ctrl Pts',(-105.5,2.99999999999999,0.));
#5886=CARTESIAN_POINT('Ctrl Pts',(-105.5,2.93749999999999,-43.6995308303615));
#5887=CARTESIAN_POINT('Ctrl Pts',(-74.5997654151808,2.87499999999999,-74.5997654151808));
#5888=CARTESIAN_POINT('Ctrl Pts',(-43.6995308303615,2.81249999999999,-105.5));
#5889=CARTESIAN_POINT('Ctrl Pts',(-6.46001186550229E-15,2.74999999999999,
-105.5));
#5890=CARTESIAN_POINT('Ctrl Pts',(43.6995308303615,2.68749999999999,-105.5));
#5891=CARTESIAN_POINT('Ctrl Pts',(74.5997654151808,2.62499999999999,-74.5997654151808));
#5892=CARTESIAN_POINT('Ctrl Pts',(105.5,2.56249999999999,-43.6995308303616));
#5893=CARTESIAN_POINT('Ctrl Pts',(105.5,2.49999999999999,-1.29200237310046E-14));
#5894=CARTESIAN_POINT('Ctrl Pts',(105.5,2.43749999999999,43.6995308303615));
#5895=CARTESIAN_POINT('Ctrl Pts',(74.5997654151808,2.37499999999999,74.5997654151808));
#5896=CARTESIAN_POINT('Ctrl Pts',(43.6995308303616,2.31249999999999,105.5));
#5897=CARTESIAN_POINT('Ctrl Pts',(1.93800355965069E-14,2.24999999999999,
105.5));
#5898=CARTESIAN_POINT('Ctrl Pts',(1.93800355965069E-14,3.37500000273118,
105.5));
#5899=CARTESIAN_POINT('Ctrl Pts',(-43.6995308303616,3.31250000273118,105.5));
#5900=CARTESIAN_POINT('Ctrl Pts',(-74.5997654151808,3.25000000273118,74.5997654151808));
#5901=CARTESIAN_POINT('Ctrl Pts',(-105.5,3.18750000273118,43.6995308303616));
#5902=CARTESIAN_POINT('Ctrl Pts',(-105.5,3.12500000273118,0.));
#5903=CARTESIAN_POINT('Ctrl Pts',(-105.5,3.06250000273118,-43.6995308303615));
#5904=CARTESIAN_POINT('Ctrl Pts',(-74.5997654151808,3.00000000273118,-74.5997654151808));
#5905=CARTESIAN_POINT('Ctrl Pts',(-43.6995308303615,2.93750000273118,-105.5));
#5906=CARTESIAN_POINT('Ctrl Pts',(-6.46001186550229E-15,2.87500000273118,
-105.5));
#5907=CARTESIAN_POINT('Ctrl Pts',(43.6995308303615,2.81250000273118,-105.5));
#5908=CARTESIAN_POINT('Ctrl Pts',(74.5997654151808,2.75000000273118,-74.5997654151808));
#5909=CARTESIAN_POINT('Ctrl Pts',(105.5,2.68750000273118,-43.6995308303616));
#5910=CARTESIAN_POINT('Ctrl Pts',(105.5,2.62500000273118,-1.29200237310046E-14));
#5911=CARTESIAN_POINT('Ctrl Pts',(105.5,2.56250000273118,43.6995308303615));
#5912=CARTESIAN_POINT('Ctrl Pts',(74.5997654151808,2.50000000273118,74.5997654151808));
#5913=CARTESIAN_POINT('Ctrl Pts',(43.6995308303616,2.43750000273118,105.5));
#5914=CARTESIAN_POINT('Ctrl Pts',(1.93800355965069E-14,2.37500000273118,
105.5));
#5915=CARTESIAN_POINT('Origin',(0.,105.,0.));
#5916=CARTESIAN_POINT('',(3.23000593275114E-15,4.37500000273118,105.5));
#5917=CARTESIAN_POINT('',(3.23000593275114E-15,4.24999999999999,105.5));
#5918=CARTESIAN_POINT('',(-1.29200237310046E-14,105.,105.5));
#5919=CARTESIAN_POINT('Ctrl Pts',(1.93800355965069E-14,4.24999999999999,
105.5));
#5920=CARTESIAN_POINT('Ctrl Pts',(-43.6995308303616,4.18749999999999,105.5));
#5921=CARTESIAN_POINT('Ctrl Pts',(-74.5997654151808,4.12499999999999,74.5997654151808));
#5922=CARTESIAN_POINT('Ctrl Pts',(-105.5,4.06249999999999,43.6995308303616));
#5923=CARTESIAN_POINT('Ctrl Pts',(-105.5,3.99999999999999,0.));
#5924=CARTESIAN_POINT('Ctrl Pts',(-105.5,3.93749999999999,-43.6995308303615));
#5925=CARTESIAN_POINT('Ctrl Pts',(-74.5997654151808,3.87499999999999,-74.5997654151808));
#5926=CARTESIAN_POINT('Ctrl Pts',(-43.6995308303615,3.81249999999999,-105.5));
#5927=CARTESIAN_POINT('Ctrl Pts',(-6.46001186550229E-15,3.74999999999999,
-105.5));
#5928=CARTESIAN_POINT('Ctrl Pts',(43.6995308303615,3.68749999999999,-105.5));
#5929=CARTESIAN_POINT('Ctrl Pts',(74.5997654151808,3.62499999999999,-74.5997654151808));
#5930=CARTESIAN_POINT('Ctrl Pts',(105.5,3.56249999999999,-43.6995308303616));
#5931=CARTESIAN_POINT('Ctrl Pts',(105.5,3.49999999999999,-1.29200237310046E-14));
#5932=CARTESIAN_POINT('Ctrl Pts',(105.5,3.43749999999999,43.6995308303615));
#5933=CARTESIAN_POINT('Ctrl Pts',(74.5997654151808,3.37499999999999,74.5997654151808));
#5934=CARTESIAN_POINT('Ctrl Pts',(43.6995308303616,3.31249999999999,105.5));
#5935=CARTESIAN_POINT('Ctrl Pts',(1.93800355965069E-14,3.24999999999999,
105.5));
#5936=CARTESIAN_POINT('Ctrl Pts',(1.93800355965069E-14,4.37500000273118,
105.5));
#5937=CARTESIAN_POINT('Ctrl Pts',(-43.6995308303616,4.31250000273118,105.5));
#5938=CARTESIAN_POINT('Ctrl Pts',(-74.5997654151808,4.25000000273118,74.5997654151808));
#5939=CARTESIAN_POINT('Ctrl Pts',(-105.5,4.18750000273118,43.6995308303616));
#5940=CARTESIAN_POINT('Ctrl Pts',(-105.5,4.12500000273118,0.));
#5941=CARTESIAN_POINT('Ctrl Pts',(-105.5,4.06250000273118,-43.6995308303615));
#5942=CARTESIAN_POINT('Ctrl Pts',(-74.5997654151808,4.00000000273118,-74.5997654151808));
#5943=CARTESIAN_POINT('Ctrl Pts',(-43.6995308303615,3.93750000273118,-105.5));
#5944=CARTESIAN_POINT('Ctrl Pts',(-6.46001186550229E-15,3.87500000273118,
-105.5));
#5945=CARTESIAN_POINT('Ctrl Pts',(43.6995308303615,3.81250000273118,-105.5));
#5946=CARTESIAN_POINT('Ctrl Pts',(74.5997654151808,3.75000000273118,-74.5997654151808));
#5947=CARTESIAN_POINT('Ctrl Pts',(105.5,3.68750000273118,-43.6995308303616));
#5948=CARTESIAN_POINT('Ctrl Pts',(105.5,3.62500000273118,-1.29200237310046E-14));
#5949=CARTESIAN_POINT('Ctrl Pts',(105.5,3.56250000273118,43.6995308303615));
#5950=CARTESIAN_POINT('Ctrl Pts',(74.5997654151808,3.50000000273118,74.5997654151808));
#5951=CARTESIAN_POINT('Ctrl Pts',(43.6995308303616,3.43750000273118,105.5));
#5952=CARTESIAN_POINT('Ctrl Pts',(1.93800355965069E-14,3.37500000273118,
105.5));
#5953=CARTESIAN_POINT('Origin',(0.,105.,0.));
#5954=CARTESIAN_POINT('',(3.23000593275114E-15,5.37500000273117,105.5));
#5955=CARTESIAN_POINT('',(3.23000593275114E-15,5.24999999999999,105.5));
#5956=CARTESIAN_POINT('',(-1.29200237310046E-14,105.,105.5));
#5957=CARTESIAN_POINT('Ctrl Pts',(1.93800355965069E-14,5.24999999999999,
105.5));
#5958=CARTESIAN_POINT('Ctrl Pts',(-43.6995308303616,5.18749999999999,105.5));
#5959=CARTESIAN_POINT('Ctrl Pts',(-74.5997654151808,5.12499999999999,74.5997654151808));
#5960=CARTESIAN_POINT('Ctrl Pts',(-105.5,5.06249999999999,43.6995308303616));
#5961=CARTESIAN_POINT('Ctrl Pts',(-105.5,4.99999999999999,0.));
#5962=CARTESIAN_POINT('Ctrl Pts',(-105.5,4.93749999999999,-43.6995308303615));
#5963=CARTESIAN_POINT('Ctrl Pts',(-74.5997654151808,4.87499999999999,-74.5997654151808));
#5964=CARTESIAN_POINT('Ctrl Pts',(-43.6995308303615,4.81249999999999,-105.5));
#5965=CARTESIAN_POINT('Ctrl Pts',(-6.46001186550229E-15,4.74999999999999,
-105.5));
#5966=CARTESIAN_POINT('Ctrl Pts',(43.6995308303615,4.68749999999999,-105.5));
#5967=CARTESIAN_POINT('Ctrl Pts',(74.5997654151808,4.62499999999999,-74.5997654151808));
#5968=CARTESIAN_POINT('Ctrl Pts',(105.5,4.56249999999999,-43.6995308303616));
#5969=CARTESIAN_POINT('Ctrl Pts',(105.5,4.49999999999999,-1.29200237310046E-14));
#5970=CARTESIAN_POINT('Ctrl Pts',(105.5,4.43749999999999,43.6995308303615));
#5971=CARTESIAN_POINT('Ctrl Pts',(74.5997654151808,4.37499999999999,74.5997654151808));
#5972=CARTESIAN_POINT('Ctrl Pts',(43.6995308303616,4.31249999999999,105.5));
#5973=CARTESIAN_POINT('Ctrl Pts',(1.93800355965069E-14,4.24999999999999,
105.5));
#5974=CARTESIAN_POINT('Ctrl Pts',(1.93800355965069E-14,5.37500000273117,
105.5));
#5975=CARTESIAN_POINT('Ctrl Pts',(-43.6995308303616,5.31250000273117,105.5));
#5976=CARTESIAN_POINT('Ctrl Pts',(-74.5997654151808,5.25000000273117,74.5997654151808));
#5977=CARTESIAN_POINT('Ctrl Pts',(-105.5,5.18750000273117,43.6995308303616));
#5978=CARTESIAN_POINT('Ctrl Pts',(-105.5,5.12500000273118,0.));
#5979=CARTESIAN_POINT('Ctrl Pts',(-105.5,5.06250000273118,-43.6995308303615));
#5980=CARTESIAN_POINT('Ctrl Pts',(-74.5997654151808,5.00000000273118,-74.5997654151808));
#5981=CARTESIAN_POINT('Ctrl Pts',(-43.6995308303615,4.93750000273118,-105.5));
#5982=CARTESIAN_POINT('Ctrl Pts',(-6.46001186550229E-15,4.87500000273118,
-105.5));
#5983=CARTESIAN_POINT('Ctrl Pts',(43.6995308303615,4.81250000273118,-105.5));
#5984=CARTESIAN_POINT('Ctrl Pts',(74.5997654151808,4.75000000273118,-74.5997654151808));
#5985=CARTESIAN_POINT('Ctrl Pts',(105.5,4.68750000273118,-43.6995308303616));
#5986=CARTESIAN_POINT('Ctrl Pts',(105.5,4.62500000273118,-1.29200237310046E-14));
#5987=CARTESIAN_POINT('Ctrl Pts',(105.5,4.56250000273118,43.6995308303615));
#5988=CARTESIAN_POINT('Ctrl Pts',(74.5997654151808,4.50000000273118,74.5997654151808));
#5989=CARTESIAN_POINT('Ctrl Pts',(43.6995308303616,4.43750000273118,105.5));
#5990=CARTESIAN_POINT('Ctrl Pts',(1.93800355965069E-14,4.37500000273118,
105.5));
#5991=CARTESIAN_POINT('Origin',(0.,105.,0.));
#5992=CARTESIAN_POINT('',(3.23000593275114E-15,6.37500000273118,105.5));
#5993=CARTESIAN_POINT('',(3.23000593275114E-15,6.24999999999998,105.5));
#5994=CARTESIAN_POINT('',(-1.29200237310046E-14,105.,105.5));
#5995=CARTESIAN_POINT('Ctrl Pts',(1.93800355965069E-14,6.24999999999998,
105.5));
#5996=CARTESIAN_POINT('Ctrl Pts',(-43.6995308303616,6.18749999999998,105.5));
#5997=CARTESIAN_POINT('Ctrl Pts',(-74.5997654151808,6.12499999999998,74.5997654151808));
#5998=CARTESIAN_POINT('Ctrl Pts',(-105.5,6.06249999999998,43.6995308303616));
#5999=CARTESIAN_POINT('Ctrl Pts',(-105.5,5.99999999999999,0.));
#6000=CARTESIAN_POINT('Ctrl Pts',(-105.5,5.93749999999999,-43.6995308303615));
#6001=CARTESIAN_POINT('Ctrl Pts',(-74.5997654151808,5.87499999999999,-74.5997654151808));
#6002=CARTESIAN_POINT('Ctrl Pts',(-43.6995308303615,5.81249999999999,-105.5));
#6003=CARTESIAN_POINT('Ctrl Pts',(-6.46001186550229E-15,5.74999999999999,
-105.5));
#6004=CARTESIAN_POINT('Ctrl Pts',(43.6995308303615,5.68749999999999,-105.5));
#6005=CARTESIAN_POINT('Ctrl Pts',(74.5997654151808,5.62499999999999,-74.5997654151808));
#6006=CARTESIAN_POINT('Ctrl Pts',(105.5,5.56249999999999,-43.6995308303616));
#6007=CARTESIAN_POINT('Ctrl Pts',(105.5,5.49999999999999,-1.29200237310046E-14));
#6008=CARTESIAN_POINT('Ctrl Pts',(105.5,5.43749999999999,43.6995308303615));
#6009=CARTESIAN_POINT('Ctrl Pts',(74.5997654151808,5.37499999999999,74.5997654151808));
#6010=CARTESIAN_POINT('Ctrl Pts',(43.6995308303616,5.31249999999999,105.5));
#6011=CARTESIAN_POINT('Ctrl Pts',(1.93800355965069E-14,5.24999999999999,
105.5));
#6012=CARTESIAN_POINT('Ctrl Pts',(1.93800355965069E-14,6.37500000273118,
105.5));
#6013=CARTESIAN_POINT('Ctrl Pts',(-43.6995308303616,6.31250000273118,105.5));
#6014=CARTESIAN_POINT('Ctrl Pts',(-74.5997654151808,6.25000000273118,74.5997654151808));
#6015=CARTESIAN_POINT('Ctrl Pts',(-105.5,6.18750000273117,43.6995308303616));
#6016=CARTESIAN_POINT('Ctrl Pts',(-105.5,6.12500000273117,0.));
#6017=CARTESIAN_POINT('Ctrl Pts',(-105.5,6.06250000273118,-43.6995308303615));
#6018=CARTESIAN_POINT('Ctrl Pts',(-74.5997654151808,6.00000000273118,-74.5997654151808));
#6019=CARTESIAN_POINT('Ctrl Pts',(-43.6995308303615,5.93750000273118,-105.5));
#6020=CARTESIAN_POINT('Ctrl Pts',(-6.46001186550229E-15,5.87500000273117,
-105.5));
#6021=CARTESIAN_POINT('Ctrl Pts',(43.6995308303615,5.81250000273117,-105.5));
#6022=CARTESIAN_POINT('Ctrl Pts',(74.5997654151808,5.75000000273118,-74.5997654151808));
#6023=CARTESIAN_POINT('Ctrl Pts',(105.5,5.68750000273117,-43.6995308303616));
#6024=CARTESIAN_POINT('Ctrl Pts',(105.5,5.62500000273117,-1.29200237310046E-14));
#6025=CARTESIAN_POINT('Ctrl Pts',(105.5,5.56250000273117,43.6995308303615));
#6026=CARTESIAN_POINT('Ctrl Pts',(74.5997654151808,5.50000000273117,74.5997654151808));
#6027=CARTESIAN_POINT('Ctrl Pts',(43.6995308303616,5.43750000273118,105.5));
#6028=CARTESIAN_POINT('Ctrl Pts',(1.93800355965069E-14,5.37500000273117,
105.5));
#6029=CARTESIAN_POINT('Origin',(0.,105.,0.));
#6030=CARTESIAN_POINT('',(3.23000593275114E-15,7.37500000273118,105.5));
#6031=CARTESIAN_POINT('',(3.23000593275114E-15,7.24999999999999,105.5));
#6032=CARTESIAN_POINT('',(-1.29200237310046E-14,105.,105.5));
#6033=CARTESIAN_POINT('Ctrl Pts',(1.93800355965069E-14,7.24999999999999,
105.5));
#6034=CARTESIAN_POINT('Ctrl Pts',(-43.6995308303616,7.18749999999999,105.5));
#6035=CARTESIAN_POINT('Ctrl Pts',(-74.5997654151808,7.12499999999999,74.5997654151808));
#6036=CARTESIAN_POINT('Ctrl Pts',(-105.5,7.06249999999998,43.6995308303616));
#6037=CARTESIAN_POINT('Ctrl Pts',(-105.5,6.99999999999998,0.));
#6038=CARTESIAN_POINT('Ctrl Pts',(-105.5,6.93749999999999,-43.6995308303615));
#6039=CARTESIAN_POINT('Ctrl Pts',(-74.5997654151808,6.87499999999999,-74.5997654151808));
#6040=CARTESIAN_POINT('Ctrl Pts',(-43.6995308303615,6.81249999999999,-105.5));
#6041=CARTESIAN_POINT('Ctrl Pts',(-6.46001186550229E-15,6.74999999999998,
-105.5));
#6042=CARTESIAN_POINT('Ctrl Pts',(43.6995308303615,6.68749999999998,-105.5));
#6043=CARTESIAN_POINT('Ctrl Pts',(74.5997654151808,6.62499999999999,-74.5997654151808));
#6044=CARTESIAN_POINT('Ctrl Pts',(105.5,6.56249999999998,-43.6995308303616));
#6045=CARTESIAN_POINT('Ctrl Pts',(105.5,6.49999999999998,-1.29200237310046E-14));
#6046=CARTESIAN_POINT('Ctrl Pts',(105.5,6.43749999999998,43.6995308303615));
#6047=CARTESIAN_POINT('Ctrl Pts',(74.5997654151808,6.37499999999998,74.5997654151808));
#6048=CARTESIAN_POINT('Ctrl Pts',(43.6995308303616,6.31249999999999,105.5));
#6049=CARTESIAN_POINT('Ctrl Pts',(1.93800355965069E-14,6.24999999999998,
105.5));
#6050=CARTESIAN_POINT('Ctrl Pts',(1.93800355965069E-14,7.37500000273118,
105.5));
#6051=CARTESIAN_POINT('Ctrl Pts',(-43.6995308303616,7.31250000273118,105.5));
#6052=CARTESIAN_POINT('Ctrl Pts',(-74.5997654151808,7.25000000273118,74.5997654151808));
#6053=CARTESIAN_POINT('Ctrl Pts',(-105.5,7.18750000273118,43.6995308303616));
#6054=CARTESIAN_POINT('Ctrl Pts',(-105.5,7.12500000273118,0.));
#6055=CARTESIAN_POINT('Ctrl Pts',(-105.5,7.06250000273118,-43.6995308303615));
#6056=CARTESIAN_POINT('Ctrl Pts',(-74.5997654151808,7.00000000273118,-74.5997654151808));
#6057=CARTESIAN_POINT('Ctrl Pts',(-43.6995308303615,6.93750000273118,-105.5));
#6058=CARTESIAN_POINT('Ctrl Pts',(-6.46001186550229E-15,6.87500000273118,
-105.5));
#6059=CARTESIAN_POINT('Ctrl Pts',(43.6995308303615,6.81250000273118,-105.5));
#6060=CARTESIAN_POINT('Ctrl Pts',(74.5997654151808,6.75000000273118,-74.5997654151808));
#6061=CARTESIAN_POINT('Ctrl Pts',(105.5,6.68750000273118,-43.6995308303616));
#6062=CARTESIAN_POINT('Ctrl Pts',(105.5,6.62500000273118,-1.29200237310046E-14));
#6063=CARTESIAN_POINT('Ctrl Pts',(105.5,6.56250000273118,43.6995308303615));
#6064=CARTESIAN_POINT('Ctrl Pts',(74.5997654151808,6.50000000273118,74.5997654151808));
#6065=CARTESIAN_POINT('Ctrl Pts',(43.6995308303616,6.43750000273118,105.5));
#6066=CARTESIAN_POINT('Ctrl Pts',(1.93800355965069E-14,6.37500000273118,
105.5));
#6067=CARTESIAN_POINT('Origin',(0.,105.,0.));
#6068=CARTESIAN_POINT('',(3.23000593275114E-15,8.37500000273118,105.5));
#6069=CARTESIAN_POINT('',(3.23000593275114E-15,8.24999999999999,105.5));
#6070=CARTESIAN_POINT('',(-1.29200237310046E-14,105.,105.5));
#6071=CARTESIAN_POINT('Ctrl Pts',(1.93800355965069E-14,8.24999999999999,
105.5));
#6072=CARTESIAN_POINT('Ctrl Pts',(-43.6995308303616,8.18749999999999,105.5));
#6073=CARTESIAN_POINT('Ctrl Pts',(-74.5997654151808,8.12499999999999,74.5997654151808));
#6074=CARTESIAN_POINT('Ctrl Pts',(-105.5,8.06249999999999,43.6995308303616));
#6075=CARTESIAN_POINT('Ctrl Pts',(-105.5,7.99999999999999,0.));
#6076=CARTESIAN_POINT('Ctrl Pts',(-105.5,7.93749999999999,-43.6995308303615));
#6077=CARTESIAN_POINT('Ctrl Pts',(-74.5997654151808,7.87499999999999,-74.5997654151808));
#6078=CARTESIAN_POINT('Ctrl Pts',(-43.6995308303615,7.81249999999999,-105.5));
#6079=CARTESIAN_POINT('Ctrl Pts',(-6.46001186550229E-15,7.74999999999999,
-105.5));
#6080=CARTESIAN_POINT('Ctrl Pts',(43.6995308303615,7.68749999999999,-105.5));
#6081=CARTESIAN_POINT('Ctrl Pts',(74.5997654151808,7.62499999999999,-74.5997654151808));
#6082=CARTESIAN_POINT('Ctrl Pts',(105.5,7.56249999999999,-43.6995308303616));
#6083=CARTESIAN_POINT('Ctrl Pts',(105.5,7.49999999999999,-1.29200237310046E-14));
#6084=CARTESIAN_POINT('Ctrl Pts',(105.5,7.43749999999999,43.6995308303615));
#6085=CARTESIAN_POINT('Ctrl Pts',(74.5997654151808,7.37499999999999,74.5997654151808));
#6086=CARTESIAN_POINT('Ctrl Pts',(43.6995308303616,7.31249999999999,105.5));
#6087=CARTESIAN_POINT('Ctrl Pts',(1.93800355965069E-14,7.24999999999999,
105.5));
#6088=CARTESIAN_POINT('Ctrl Pts',(1.93800355965069E-14,8.37500000273118,
105.5));
#6089=CARTESIAN_POINT('Ctrl Pts',(-43.6995308303616,8.31250000273118,105.5));
#6090=CARTESIAN_POINT('Ctrl Pts',(-74.5997654151808,8.25000000273118,74.5997654151808));
#6091=CARTESIAN_POINT('Ctrl Pts',(-105.5,8.18750000273118,43.6995308303616));
#6092=CARTESIAN_POINT('Ctrl Pts',(-105.5,8.12500000273118,0.));
#6093=CARTESIAN_POINT('Ctrl Pts',(-105.5,8.06250000273118,-43.6995308303615));
#6094=CARTESIAN_POINT('Ctrl Pts',(-74.5997654151808,8.00000000273118,-74.5997654151808));
#6095=CARTESIAN_POINT('Ctrl Pts',(-43.6995308303615,7.93750000273118,-105.5));
#6096=CARTESIAN_POINT('Ctrl Pts',(-6.46001186550229E-15,7.87500000273118,
-105.5));
#6097=CARTESIAN_POINT('Ctrl Pts',(43.6995308303615,7.81250000273118,-105.5));
#6098=CARTESIAN_POINT('Ctrl Pts',(74.5997654151808,7.75000000273118,-74.5997654151808));
#6099=CARTESIAN_POINT('Ctrl Pts',(105.5,7.68750000273118,-43.6995308303616));
#6100=CARTESIAN_POINT('Ctrl Pts',(105.5,7.62500000273118,-1.29200237310046E-14));
#6101=CARTESIAN_POINT('Ctrl Pts',(105.5,7.56250000273118,43.6995308303615));
#6102=CARTESIAN_POINT('Ctrl Pts',(74.5997654151808,7.50000000273118,74.5997654151808));
#6103=CARTESIAN_POINT('Ctrl Pts',(43.6995308303616,7.43750000273118,105.5));
#6104=CARTESIAN_POINT('Ctrl Pts',(1.93800355965069E-14,7.37500000273118,
105.5));
#6105=CARTESIAN_POINT('Origin',(0.,105.,0.));
#6106=CARTESIAN_POINT('',(3.23000593275114E-15,9.37500000273118,105.5));
#6107=CARTESIAN_POINT('',(3.23000593275114E-15,9.24999999999999,105.5));
#6108=CARTESIAN_POINT('',(-1.29200237310046E-14,105.,105.5));
#6109=CARTESIAN_POINT('Ctrl Pts',(1.93800355965069E-14,9.24999999999999,
105.5));
#6110=CARTESIAN_POINT('Ctrl Pts',(-43.6995308303616,9.18749999999999,105.5));
#6111=CARTESIAN_POINT('Ctrl Pts',(-74.5997654151808,9.12499999999999,74.5997654151808));
#6112=CARTESIAN_POINT('Ctrl Pts',(-105.5,9.06249999999999,43.6995308303616));
#6113=CARTESIAN_POINT('Ctrl Pts',(-105.5,8.99999999999999,0.));
#6114=CARTESIAN_POINT('Ctrl Pts',(-105.5,8.93749999999999,-43.6995308303615));
#6115=CARTESIAN_POINT('Ctrl Pts',(-74.5997654151808,8.87499999999999,-74.5997654151808));
#6116=CARTESIAN_POINT('Ctrl Pts',(-43.6995308303615,8.81249999999999,-105.5));
#6117=CARTESIAN_POINT('Ctrl Pts',(-6.46001186550229E-15,8.74999999999999,
-105.5));
#6118=CARTESIAN_POINT('Ctrl Pts',(43.6995308303615,8.68749999999999,-105.5));
#6119=CARTESIAN_POINT('Ctrl Pts',(74.5997654151808,8.62499999999999,-74.5997654151808));
#6120=CARTESIAN_POINT('Ctrl Pts',(105.5,8.56249999999999,-43.6995308303616));
#6121=CARTESIAN_POINT('Ctrl Pts',(105.5,8.49999999999999,-1.29200237310046E-14));
#6122=CARTESIAN_POINT('Ctrl Pts',(105.5,8.43749999999999,43.6995308303615));
#6123=CARTESIAN_POINT('Ctrl Pts',(74.5997654151808,8.37499999999999,74.5997654151808));
#6124=CARTESIAN_POINT('Ctrl Pts',(43.6995308303616,8.31249999999999,105.5));
#6125=CARTESIAN_POINT('Ctrl Pts',(1.93800355965069E-14,8.24999999999999,
105.5));
#6126=CARTESIAN_POINT('Ctrl Pts',(1.93800355965069E-14,9.37500000273118,
105.5));
#6127=CARTESIAN_POINT('Ctrl Pts',(-43.6995308303616,9.31250000273118,105.5));
#6128=CARTESIAN_POINT('Ctrl Pts',(-74.5997654151808,9.25000000273118,74.5997654151808));
#6129=CARTESIAN_POINT('Ctrl Pts',(-105.5,9.18750000273118,43.6995308303616));
#6130=CARTESIAN_POINT('Ctrl Pts',(-105.5,9.12500000273118,0.));
#6131=CARTESIAN_POINT('Ctrl Pts',(-105.5,9.06250000273118,-43.6995308303615));
#6132=CARTESIAN_POINT('Ctrl Pts',(-74.5997654151808,9.00000000273118,-74.5997654151808));
#6133=CARTESIAN_POINT('Ctrl Pts',(-43.6995308303615,8.93750000273118,-105.5));
#6134=CARTESIAN_POINT('Ctrl Pts',(-6.46001186550229E-15,8.87500000273118,
-105.5));
#6135=CARTESIAN_POINT('Ctrl Pts',(43.6995308303615,8.81250000273118,-105.5));
#6136=CARTESIAN_POINT('Ctrl Pts',(74.5997654151808,8.75000000273118,-74.5997654151808));
#6137=CARTESIAN_POINT('Ctrl Pts',(105.5,8.68750000273118,-43.6995308303616));
#6138=CARTESIAN_POINT('Ctrl Pts',(105.5,8.62500000273118,-1.29200237310046E-14));
#6139=CARTESIAN_POINT('Ctrl Pts',(105.5,8.56250000273118,43.6995308303615));
#6140=CARTESIAN_POINT('Ctrl Pts',(74.5997654151808,8.50000000273118,74.5997654151808));
#6141=CARTESIAN_POINT('Ctrl Pts',(43.6995308303616,8.43750000273118,105.5));
#6142=CARTESIAN_POINT('Ctrl Pts',(1.93800355965069E-14,8.37500000273118,
105.5));
#6143=CARTESIAN_POINT('Origin',(0.,105.,0.));
#6144=CARTESIAN_POINT('',(3.23000593275114E-15,10.3750000027312,105.5));
#6145=CARTESIAN_POINT('',(3.23000593275114E-15,10.25,105.5));
#6146=CARTESIAN_POINT('',(-1.29200237310046E-14,105.,105.5));
#6147=CARTESIAN_POINT('Ctrl Pts',(1.93800355965069E-14,10.25,105.5));
#6148=CARTESIAN_POINT('Ctrl Pts',(-43.6995308303616,10.1875,105.5));
#6149=CARTESIAN_POINT('Ctrl Pts',(-74.5997654151808,10.125,74.5997654151808));
#6150=CARTESIAN_POINT('Ctrl Pts',(-105.5,10.0625,43.6995308303616));
#6151=CARTESIAN_POINT('Ctrl Pts',(-105.5,9.99999999999999,0.));
#6152=CARTESIAN_POINT('Ctrl Pts',(-105.5,9.93749999999999,-43.6995308303615));
#6153=CARTESIAN_POINT('Ctrl Pts',(-74.5997654151808,9.87499999999999,-74.5997654151808));
#6154=CARTESIAN_POINT('Ctrl Pts',(-43.6995308303615,9.81249999999999,-105.5));
#6155=CARTESIAN_POINT('Ctrl Pts',(-6.46001186550229E-15,9.74999999999999,
-105.5));
#6156=CARTESIAN_POINT('Ctrl Pts',(43.6995308303615,9.68749999999999,-105.5));
#6157=CARTESIAN_POINT('Ctrl Pts',(74.5997654151808,9.62499999999999,-74.5997654151808));
#6158=CARTESIAN_POINT('Ctrl Pts',(105.5,9.56249999999999,-43.6995308303616));
#6159=CARTESIAN_POINT('Ctrl Pts',(105.5,9.49999999999999,-1.29200237310046E-14));
#6160=CARTESIAN_POINT('Ctrl Pts',(105.5,9.43749999999999,43.6995308303615));
#6161=CARTESIAN_POINT('Ctrl Pts',(74.5997654151808,9.37499999999999,74.5997654151808));
#6162=CARTESIAN_POINT('Ctrl Pts',(43.6995308303616,9.31249999999999,105.5));
#6163=CARTESIAN_POINT('Ctrl Pts',(1.93800355965069E-14,9.24999999999999,
105.5));
#6164=CARTESIAN_POINT('Ctrl Pts',(1.93800355965069E-14,10.3750000027312,
105.5));
#6165=CARTESIAN_POINT('Ctrl Pts',(-43.6995308303616,10.3125000027312,105.5));
#6166=CARTESIAN_POINT('Ctrl Pts',(-74.5997654151808,10.2500000027312,74.5997654151808));
#6167=CARTESIAN_POINT('Ctrl Pts',(-105.5,10.1875000027312,43.6995308303616));
#6168=CARTESIAN_POINT('Ctrl Pts',(-105.5,10.1250000027312,0.));
#6169=CARTESIAN_POINT('Ctrl Pts',(-105.5,10.0625000027312,-43.6995308303615));
#6170=CARTESIAN_POINT('Ctrl Pts',(-74.5997654151808,10.0000000027312,-74.5997654151808));
#6171=CARTESIAN_POINT('Ctrl Pts',(-43.6995308303615,9.93750000273118,-105.5));
#6172=CARTESIAN_POINT('Ctrl Pts',(-6.46001186550229E-15,9.87500000273118,
-105.5));
#6173=CARTESIAN_POINT('Ctrl Pts',(43.6995308303615,9.81250000273118,-105.5));
#6174=CARTESIAN_POINT('Ctrl Pts',(74.5997654151808,9.75000000273118,-74.5997654151808));
#6175=CARTESIAN_POINT('Ctrl Pts',(105.5,9.68750000273118,-43.6995308303616));
#6176=CARTESIAN_POINT('Ctrl Pts',(105.5,9.62500000273118,-1.29200237310046E-14));
#6177=CARTESIAN_POINT('Ctrl Pts',(105.5,9.56250000273118,43.6995308303615));
#6178=CARTESIAN_POINT('Ctrl Pts',(74.5997654151808,9.50000000273118,74.5997654151808));
#6179=CARTESIAN_POINT('Ctrl Pts',(43.6995308303616,9.43750000273118,105.5));
#6180=CARTESIAN_POINT('Ctrl Pts',(1.93800355965069E-14,9.37500000273118,
105.5));
#6181=CARTESIAN_POINT('Origin',(0.,105.,0.));
#6182=CARTESIAN_POINT('',(3.23000593275114E-15,11.3750000027312,105.5));
#6183=CARTESIAN_POINT('',(3.23000593275114E-15,11.25,105.5));
#6184=CARTESIAN_POINT('',(-1.29200237310046E-14,105.,105.5));
#6185=CARTESIAN_POINT('Ctrl Pts',(1.93800355965069E-14,11.25,105.5));
#6186=CARTESIAN_POINT('Ctrl Pts',(-43.6995308303616,11.1875,105.5));
#6187=CARTESIAN_POINT('Ctrl Pts',(-74.5997654151808,11.125,74.5997654151808));
#6188=CARTESIAN_POINT('Ctrl Pts',(-105.5,11.0625,43.6995308303616));
#6189=CARTESIAN_POINT('Ctrl Pts',(-105.5,11.,0.));
#6190=CARTESIAN_POINT('Ctrl Pts',(-105.5,10.9375,-43.6995308303615));
#6191=CARTESIAN_POINT('Ctrl Pts',(-74.5997654151808,10.875,-74.5997654151808));
#6192=CARTESIAN_POINT('Ctrl Pts',(-43.6995308303615,10.8125,-105.5));
#6193=CARTESIAN_POINT('Ctrl Pts',(-6.46001186550229E-15,10.75,-105.5));
#6194=CARTESIAN_POINT('Ctrl Pts',(43.6995308303615,10.6875,-105.5));
#6195=CARTESIAN_POINT('Ctrl Pts',(74.5997654151808,10.625,-74.5997654151808));
#6196=CARTESIAN_POINT('Ctrl Pts',(105.5,10.5625,-43.6995308303616));
#6197=CARTESIAN_POINT('Ctrl Pts',(105.5,10.5,-1.29200237310046E-14));
#6198=CARTESIAN_POINT('Ctrl Pts',(105.5,10.4375,43.6995308303615));
#6199=CARTESIAN_POINT('Ctrl Pts',(74.5997654151808,10.375,74.5997654151808));
#6200=CARTESIAN_POINT('Ctrl Pts',(43.6995308303616,10.3125,105.5));
#6201=CARTESIAN_POINT('Ctrl Pts',(1.93800355965069E-14,10.25,105.5));
#6202=CARTESIAN_POINT('Ctrl Pts',(1.93800355965069E-14,11.3750000027312,
105.5));
#6203=CARTESIAN_POINT('Ctrl Pts',(-43.6995308303616,11.3125000027312,105.5));
#6204=CARTESIAN_POINT('Ctrl Pts',(-74.5997654151808,11.2500000027312,74.5997654151808));
#6205=CARTESIAN_POINT('Ctrl Pts',(-105.5,11.1875000027312,43.6995308303616));
#6206=CARTESIAN_POINT('Ctrl Pts',(-105.5,11.1250000027312,0.));
#6207=CARTESIAN_POINT('Ctrl Pts',(-105.5,11.0625000027312,-43.6995308303615));
#6208=CARTESIAN_POINT('Ctrl Pts',(-74.5997654151808,11.0000000027312,-74.5997654151808));
#6209=CARTESIAN_POINT('Ctrl Pts',(-43.6995308303615,10.9375000027312,-105.5));
#6210=CARTESIAN_POINT('Ctrl Pts',(-6.46001186550229E-15,10.8750000027312,
-105.5));
#6211=CARTESIAN_POINT('Ctrl Pts',(43.6995308303615,10.8125000027312,-105.5));
#6212=CARTESIAN_POINT('Ctrl Pts',(74.5997654151808,10.7500000027312,-74.5997654151808));
#6213=CARTESIAN_POINT('Ctrl Pts',(105.5,10.6875000027312,-43.6995308303616));
#6214=CARTESIAN_POINT('Ctrl Pts',(105.5,10.6250000027312,-1.29200237310046E-14));
#6215=CARTESIAN_POINT('Ctrl Pts',(105.5,10.5625000027312,43.6995308303615));
#6216=CARTESIAN_POINT('Ctrl Pts',(74.5997654151808,10.5000000027312,74.5997654151808));
#6217=CARTESIAN_POINT('Ctrl Pts',(43.6995308303616,10.4375000027312,105.5));
#6218=CARTESIAN_POINT('Ctrl Pts',(1.93800355965069E-14,10.3750000027312,
105.5));
#6219=CARTESIAN_POINT('Origin',(0.,105.,0.));
#6220=CARTESIAN_POINT('',(3.23000593275114E-15,12.3750000027312,105.5));
#6221=CARTESIAN_POINT('',(3.23000593275114E-15,12.25,105.5));
#6222=CARTESIAN_POINT('',(-1.29200237310046E-14,105.,105.5));
#6223=CARTESIAN_POINT('Ctrl Pts',(1.93800355965069E-14,12.25,105.5));
#6224=CARTESIAN_POINT('Ctrl Pts',(-43.6995308303616,12.1875,105.5));
#6225=CARTESIAN_POINT('Ctrl Pts',(-74.5997654151808,12.125,74.5997654151808));
#6226=CARTESIAN_POINT('Ctrl Pts',(-105.5,12.0625,43.6995308303616));
#6227=CARTESIAN_POINT('Ctrl Pts',(-105.5,12.,0.));
#6228=CARTESIAN_POINT('Ctrl Pts',(-105.5,11.9375,-43.6995308303615));
#6229=CARTESIAN_POINT('Ctrl Pts',(-74.5997654151808,11.875,-74.5997654151808));
#6230=CARTESIAN_POINT('Ctrl Pts',(-43.6995308303615,11.8125,-105.5));
#6231=CARTESIAN_POINT('Ctrl Pts',(-6.46001186550229E-15,11.75,-105.5));
#6232=CARTESIAN_POINT('Ctrl Pts',(43.6995308303615,11.6875,-105.5));
#6233=CARTESIAN_POINT('Ctrl Pts',(74.5997654151808,11.625,-74.5997654151808));
#6234=CARTESIAN_POINT('Ctrl Pts',(105.5,11.5625,-43.6995308303616));
#6235=CARTESIAN_POINT('Ctrl Pts',(105.5,11.5,-1.29200237310046E-14));
#6236=CARTESIAN_POINT('Ctrl Pts',(105.5,11.4375,43.6995308303615));
#6237=CARTESIAN_POINT('Ctrl Pts',(74.5997654151808,11.375,74.5997654151808));
#6238=CARTESIAN_POINT('Ctrl Pts',(43.6995308303616,11.3125,105.5));
#6239=CARTESIAN_POINT('Ctrl Pts',(1.93800355965069E-14,11.25,105.5));
#6240=CARTESIAN_POINT('Ctrl Pts',(1.93800355965069E-14,12.3750000027312,
105.5));
#6241=CARTESIAN_POINT('Ctrl Pts',(-43.6995308303616,12.3125000027312,105.5));
#6242=CARTESIAN_POINT('Ctrl Pts',(-74.5997654151808,12.2500000027312,74.5997654151808));
#6243=CARTESIAN_POINT('Ctrl Pts',(-105.5,12.1875000027312,43.6995308303616));
#6244=CARTESIAN_POINT('Ctrl Pts',(-105.5,12.1250000027312,0.));
#6245=CARTESIAN_POINT('Ctrl Pts',(-105.5,12.0625000027312,-43.6995308303615));
#6246=CARTESIAN_POINT('Ctrl Pts',(-74.5997654151808,12.0000000027312,-74.5997654151808));
#6247=CARTESIAN_POINT('Ctrl Pts',(-43.6995308303615,11.9375000027312,-105.5));
#6248=CARTESIAN_POINT('Ctrl Pts',(-6.46001186550229E-15,11.8750000027312,
-105.5));
#6249=CARTESIAN_POINT('Ctrl Pts',(43.6995308303615,11.8125000027312,-105.5));
#6250=CARTESIAN_POINT('Ctrl Pts',(74.5997654151808,11.7500000027312,-74.5997654151808));
#6251=CARTESIAN_POINT('Ctrl Pts',(105.5,11.6875000027312,-43.6995308303616));
#6252=CARTESIAN_POINT('Ctrl Pts',(105.5,11.6250000027312,-1.29200237310046E-14));
#6253=CARTESIAN_POINT('Ctrl Pts',(105.5,11.5625000027312,43.6995308303615));
#6254=CARTESIAN_POINT('Ctrl Pts',(74.5997654151808,11.5000000027312,74.5997654151808));
#6255=CARTESIAN_POINT('Ctrl Pts',(43.6995308303616,11.4375000027312,105.5));
#6256=CARTESIAN_POINT('Ctrl Pts',(1.93800355965069E-14,11.3750000027312,
105.5));
#6257=CARTESIAN_POINT('Origin',(0.,105.,0.));
#6258=CARTESIAN_POINT('',(3.23000593275114E-15,13.3750000027312,105.5));
#6259=CARTESIAN_POINT('',(3.23000593275114E-15,13.25,105.5));
#6260=CARTESIAN_POINT('',(-1.29200237310046E-14,105.,105.5));
#6261=CARTESIAN_POINT('Ctrl Pts',(1.93800355965069E-14,13.25,105.5));
#6262=CARTESIAN_POINT('Ctrl Pts',(-43.6995308303616,13.1875,105.5));
#6263=CARTESIAN_POINT('Ctrl Pts',(-74.5997654151808,13.125,74.5997654151808));
#6264=CARTESIAN_POINT('Ctrl Pts',(-105.5,13.0625,43.6995308303616));
#6265=CARTESIAN_POINT('Ctrl Pts',(-105.5,13.,0.));
#6266=CARTESIAN_POINT('Ctrl Pts',(-105.5,12.9375,-43.6995308303615));
#6267=CARTESIAN_POINT('Ctrl Pts',(-74.5997654151808,12.875,-74.5997654151808));
#6268=CARTESIAN_POINT('Ctrl Pts',(-43.6995308303615,12.8125,-105.5));
#6269=CARTESIAN_POINT('Ctrl Pts',(-6.46001186550229E-15,12.75,-105.5));
#6270=CARTESIAN_POINT('Ctrl Pts',(43.6995308303615,12.6875,-105.5));
#6271=CARTESIAN_POINT('Ctrl Pts',(74.5997654151808,12.625,-74.5997654151808));
#6272=CARTESIAN_POINT('Ctrl Pts',(105.5,12.5625,-43.6995308303616));
#6273=CARTESIAN_POINT('Ctrl Pts',(105.5,12.5,-1.29200237310046E-14));
#6274=CARTESIAN_POINT('Ctrl Pts',(105.5,12.4375,43.6995308303615));
#6275=CARTESIAN_POINT('Ctrl Pts',(74.5997654151808,12.375,74.5997654151808));
#6276=CARTESIAN_POINT('Ctrl Pts',(43.6995308303616,12.3125,105.5));
#6277=CARTESIAN_POINT('Ctrl Pts',(1.93800355965069E-14,12.25,105.5));
#6278=CARTESIAN_POINT('Ctrl Pts',(1.93800355965069E-14,13.3750000027312,
105.5));
#6279=CARTESIAN_POINT('Ctrl Pts',(-43.6995308303616,13.3125000027312,105.5));
#6280=CARTESIAN_POINT('Ctrl Pts',(-74.5997654151808,13.2500000027312,74.5997654151808));
#6281=CARTESIAN_POINT('Ctrl Pts',(-105.5,13.1875000027312,43.6995308303616));
#6282=CARTESIAN_POINT('Ctrl Pts',(-105.5,13.1250000027312,0.));
#6283=CARTESIAN_POINT('Ctrl Pts',(-105.5,13.0625000027312,-43.6995308303615));
#6284=CARTESIAN_POINT('Ctrl Pts',(-74.5997654151808,13.0000000027312,-74.5997654151808));
#6285=CARTESIAN_POINT('Ctrl Pts',(-43.6995308303615,12.9375000027312,-105.5));
#6286=CARTESIAN_POINT('Ctrl Pts',(-6.46001186550229E-15,12.8750000027312,
-105.5));
#6287=CARTESIAN_POINT('Ctrl Pts',(43.6995308303615,12.8125000027312,-105.5));
#6288=CARTESIAN_POINT('Ctrl Pts',(74.5997654151808,12.7500000027312,-74.5997654151808));
#6289=CARTESIAN_POINT('Ctrl Pts',(105.5,12.6875000027312,-43.6995308303616));
#6290=CARTESIAN_POINT('Ctrl Pts',(105.5,12.6250000027312,-1.29200237310046E-14));
#6291=CARTESIAN_POINT('Ctrl Pts',(105.5,12.5625000027312,43.6995308303615));
#6292=CARTESIAN_POINT('Ctrl Pts',(74.5997654151808,12.5000000027312,74.5997654151808));
#6293=CARTESIAN_POINT('Ctrl Pts',(43.6995308303616,12.4375000027312,105.5));
#6294=CARTESIAN_POINT('Ctrl Pts',(1.93800355965069E-14,12.3750000027312,
105.5));
#6295=CARTESIAN_POINT('Origin',(0.,105.,0.));
#6296=CARTESIAN_POINT('',(3.23000593275114E-15,14.3750000027312,105.5));
#6297=CARTESIAN_POINT('',(3.23000593275114E-15,14.25,105.5));
#6298=CARTESIAN_POINT('',(-1.29200237310046E-14,105.,105.5));
#6299=CARTESIAN_POINT('Ctrl Pts',(1.93800355965069E-14,14.25,105.5));
#6300=CARTESIAN_POINT('Ctrl Pts',(-43.6995308303616,14.1875,105.5));
#6301=CARTESIAN_POINT('Ctrl Pts',(-74.5997654151808,14.125,74.5997654151808));
#6302=CARTESIAN_POINT('Ctrl Pts',(-105.5,14.0625,43.6995308303616));
#6303=CARTESIAN_POINT('Ctrl Pts',(-105.5,14.,0.));
#6304=CARTESIAN_POINT('Ctrl Pts',(-105.5,13.9375,-43.6995308303615));
#6305=CARTESIAN_POINT('Ctrl Pts',(-74.5997654151808,13.875,-74.5997654151808));
#6306=CARTESIAN_POINT('Ctrl Pts',(-43.6995308303615,13.8125,-105.5));
#6307=CARTESIAN_POINT('Ctrl Pts',(-6.46001186550229E-15,13.75,-105.5));
#6308=CARTESIAN_POINT('Ctrl Pts',(43.6995308303615,13.6875,-105.5));
#6309=CARTESIAN_POINT('Ctrl Pts',(74.5997654151808,13.625,-74.5997654151808));
#6310=CARTESIAN_POINT('Ctrl Pts',(105.5,13.5625,-43.6995308303616));
#6311=CARTESIAN_POINT('Ctrl Pts',(105.5,13.5,-1.29200237310046E-14));
#6312=CARTESIAN_POINT('Ctrl Pts',(105.5,13.4375,43.6995308303615));
#6313=CARTESIAN_POINT('Ctrl Pts',(74.5997654151808,13.375,74.5997654151808));
#6314=CARTESIAN_POINT('Ctrl Pts',(43.6995308303616,13.3125,105.5));
#6315=CARTESIAN_POINT('Ctrl Pts',(1.93800355965069E-14,13.25,105.5));
#6316=CARTESIAN_POINT('Ctrl Pts',(1.93800355965069E-14,14.3750000027312,
105.5));
#6317=CARTESIAN_POINT('Ctrl Pts',(-43.6995308303616,14.3125000027312,105.5));
#6318=CARTESIAN_POINT('Ctrl Pts',(-74.5997654151808,14.2500000027312,74.5997654151808));
#6319=CARTESIAN_POINT('Ctrl Pts',(-105.5,14.1875000027312,43.6995308303616));
#6320=CARTESIAN_POINT('Ctrl Pts',(-105.5,14.1250000027312,0.));
#6321=CARTESIAN_POINT('Ctrl Pts',(-105.5,14.0625000027312,-43.6995308303615));
#6322=CARTESIAN_POINT('Ctrl Pts',(-74.5997654151808,14.0000000027312,-74.5997654151808));
#6323=CARTESIAN_POINT('Ctrl Pts',(-43.6995308303615,13.9375000027312,-105.5));
#6324=CARTESIAN_POINT('Ctrl Pts',(-6.46001186550229E-15,13.8750000027312,
-105.5));
#6325=CARTESIAN_POINT('Ctrl Pts',(43.6995308303615,13.8125000027312,-105.5));
#6326=CARTESIAN_POINT('Ctrl Pts',(74.5997654151808,13.7500000027312,-74.5997654151808));
#6327=CARTESIAN_POINT('Ctrl Pts',(105.5,13.6875000027312,-43.6995308303616));
#6328=CARTESIAN_POINT('Ctrl Pts',(105.5,13.6250000027312,-1.29200237310046E-14));
#6329=CARTESIAN_POINT('Ctrl Pts',(105.5,13.5625000027312,43.6995308303615));
#6330=CARTESIAN_POINT('Ctrl Pts',(74.5997654151808,13.5000000027312,74.5997654151808));
#6331=CARTESIAN_POINT('Ctrl Pts',(43.6995308303616,13.4375000027312,105.5));
#6332=CARTESIAN_POINT('Ctrl Pts',(1.93800355965069E-14,13.3750000027312,
105.5));
#6333=CARTESIAN_POINT('Origin',(0.,105.,0.));
#6334=CARTESIAN_POINT('',(3.23000593275114E-15,15.3750000027312,105.5));
#6335=CARTESIAN_POINT('',(3.23000593275114E-15,15.25,105.5));
#6336=CARTESIAN_POINT('',(-1.29200237310046E-14,105.,105.5));
#6337=CARTESIAN_POINT('Ctrl Pts',(1.93800355965069E-14,15.25,105.5));
#6338=CARTESIAN_POINT('Ctrl Pts',(-43.6995308303616,15.1875,105.5));
#6339=CARTESIAN_POINT('Ctrl Pts',(-74.5997654151808,15.125,74.5997654151808));
#6340=CARTESIAN_POINT('Ctrl Pts',(-105.5,15.0625,43.6995308303616));
#6341=CARTESIAN_POINT('Ctrl Pts',(-105.5,15.,0.));
#6342=CARTESIAN_POINT('Ctrl Pts',(-105.5,14.9375,-43.6995308303615));
#6343=CARTESIAN_POINT('Ctrl Pts',(-74.5997654151808,14.875,-74.5997654151808));
#6344=CARTESIAN_POINT('Ctrl Pts',(-43.6995308303615,14.8125,-105.5));
#6345=CARTESIAN_POINT('Ctrl Pts',(-6.46001186550229E-15,14.75,-105.5));
#6346=CARTESIAN_POINT('Ctrl Pts',(43.6995308303615,14.6875,-105.5));
#6347=CARTESIAN_POINT('Ctrl Pts',(74.5997654151808,14.625,-74.5997654151808));
#6348=CARTESIAN_POINT('Ctrl Pts',(105.5,14.5625,-43.6995308303616));
#6349=CARTESIAN_POINT('Ctrl Pts',(105.5,14.5,-1.29200237310046E-14));
#6350=CARTESIAN_POINT('Ctrl Pts',(105.5,14.4375,43.6995308303615));
#6351=CARTESIAN_POINT('Ctrl Pts',(74.5997654151808,14.375,74.5997654151808));
#6352=CARTESIAN_POINT('Ctrl Pts',(43.6995308303616,14.3125,105.5));
#6353=CARTESIAN_POINT('Ctrl Pts',(1.93800355965069E-14,14.25,105.5));
#6354=CARTESIAN_POINT('Ctrl Pts',(1.93800355965069E-14,15.3750000027312,
105.5));
#6355=CARTESIAN_POINT('Ctrl Pts',(-43.6995308303616,15.3125000027312,105.5));
#6356=CARTESIAN_POINT('Ctrl Pts',(-74.5997654151808,15.2500000027312,74.5997654151808));
#6357=CARTESIAN_POINT('Ctrl Pts',(-105.5,15.1875000027312,43.6995308303616));
#6358=CARTESIAN_POINT('Ctrl Pts',(-105.5,15.1250000027312,0.));
#6359=CARTESIAN_POINT('Ctrl Pts',(-105.5,15.0625000027312,-43.6995308303615));
#6360=CARTESIAN_POINT('Ctrl Pts',(-74.5997654151808,15.0000000027312,-74.5997654151808));
#6361=CARTESIAN_POINT('Ctrl Pts',(-43.6995308303615,14.9375000027312,-105.5));
#6362=CARTESIAN_POINT('Ctrl Pts',(-6.46001186550229E-15,14.8750000027312,
-105.5));
#6363=CARTESIAN_POINT('Ctrl Pts',(43.6995308303615,14.8125000027312,-105.5));
#6364=CARTESIAN_POINT('Ctrl Pts',(74.5997654151808,14.7500000027312,-74.5997654151808));
#6365=CARTESIAN_POINT('Ctrl Pts',(105.5,14.6875000027312,-43.6995308303616));
#6366=CARTESIAN_POINT('Ctrl Pts',(105.5,14.6250000027312,-1.29200237310046E-14));
#6367=CARTESIAN_POINT('Ctrl Pts',(105.5,14.5625000027312,43.6995308303615));
#6368=CARTESIAN_POINT('Ctrl Pts',(74.5997654151808,14.5000000027312,74.5997654151808));
#6369=CARTESIAN_POINT('Ctrl Pts',(43.6995308303616,14.4375000027312,105.5));
#6370=CARTESIAN_POINT('Ctrl Pts',(1.93800355965069E-14,14.3750000027312,
105.5));
#6371=CARTESIAN_POINT('Origin',(0.,105.,0.));
#6372=CARTESIAN_POINT('',(3.23000593275114E-15,16.3750000027312,105.5));
#6373=CARTESIAN_POINT('',(3.23000593275114E-15,16.25,105.5));
#6374=CARTESIAN_POINT('',(-1.29200237310046E-14,105.,105.5));
#6375=CARTESIAN_POINT('Ctrl Pts',(1.93800355965069E-14,16.25,105.5));
#6376=CARTESIAN_POINT('Ctrl Pts',(-43.6995308303616,16.1875,105.5));
#6377=CARTESIAN_POINT('Ctrl Pts',(-74.5997654151808,16.125,74.5997654151808));
#6378=CARTESIAN_POINT('Ctrl Pts',(-105.5,16.0625,43.6995308303616));
#6379=CARTESIAN_POINT('Ctrl Pts',(-105.5,16.,0.));
#6380=CARTESIAN_POINT('Ctrl Pts',(-105.5,15.9375,-43.6995308303615));
#6381=CARTESIAN_POINT('Ctrl Pts',(-74.5997654151808,15.875,-74.5997654151808));
#6382=CARTESIAN_POINT('Ctrl Pts',(-43.6995308303615,15.8125,-105.5));
#6383=CARTESIAN_POINT('Ctrl Pts',(-6.46001186550229E-15,15.75,-105.5));
#6384=CARTESIAN_POINT('Ctrl Pts',(43.6995308303615,15.6875,-105.5));
#6385=CARTESIAN_POINT('Ctrl Pts',(74.5997654151808,15.625,-74.5997654151808));
#6386=CARTESIAN_POINT('Ctrl Pts',(105.5,15.5625,-43.6995308303616));
#6387=CARTESIAN_POINT('Ctrl Pts',(105.5,15.5,-1.29200237310046E-14));
#6388=CARTESIAN_POINT('Ctrl Pts',(105.5,15.4375,43.6995308303615));
#6389=CARTESIAN_POINT('Ctrl Pts',(74.5997654151808,15.375,74.5997654151808));
#6390=CARTESIAN_POINT('Ctrl Pts',(43.6995308303616,15.3125,105.5));
#6391=CARTESIAN_POINT('Ctrl Pts',(1.93800355965069E-14,15.25,105.5));
#6392=CARTESIAN_POINT('Ctrl Pts',(1.93800355965069E-14,16.3750000027312,
105.5));
#6393=CARTESIAN_POINT('Ctrl Pts',(-43.6995308303616,16.3125000027312,105.5));
#6394=CARTESIAN_POINT('Ctrl Pts',(-74.5997654151808,16.2500000027312,74.5997654151808));
#6395=CARTESIAN_POINT('Ctrl Pts',(-105.5,16.1875000027312,43.6995308303616));
#6396=CARTESIAN_POINT('Ctrl Pts',(-105.5,16.1250000027312,0.));
#6397=CARTESIAN_POINT('Ctrl Pts',(-105.5,16.0625000027312,-43.6995308303615));
#6398=CARTESIAN_POINT('Ctrl Pts',(-74.5997654151808,16.0000000027312,-74.5997654151808));
#6399=CARTESIAN_POINT('Ctrl Pts',(-43.6995308303615,15.9375000027312,-105.5));
#6400=CARTESIAN_POINT('Ctrl Pts',(-6.46001186550229E-15,15.8750000027312,
-105.5));
#6401=CARTESIAN_POINT('Ctrl Pts',(43.6995308303615,15.8125000027312,-105.5));
#6402=CARTESIAN_POINT('Ctrl Pts',(74.5997654151808,15.7500000027312,-74.5997654151808));
#6403=CARTESIAN_POINT('Ctrl Pts',(105.5,15.6875000027312,-43.6995308303616));
#6404=CARTESIAN_POINT('Ctrl Pts',(105.5,15.6250000027312,-1.29200237310046E-14));
#6405=CARTESIAN_POINT('Ctrl Pts',(105.5,15.5625000027312,43.6995308303615));
#6406=CARTESIAN_POINT('Ctrl Pts',(74.5997654151808,15.5000000027312,74.5997654151808));
#6407=CARTESIAN_POINT('Ctrl Pts',(43.6995308303616,15.4375000027312,105.5));
#6408=CARTESIAN_POINT('Ctrl Pts',(1.93800355965069E-14,15.3750000027312,
105.5));
#6409=CARTESIAN_POINT('Origin',(0.,105.,0.));
#6410=CARTESIAN_POINT('',(3.23000593275114E-15,17.3750000027312,105.5));
#6411=CARTESIAN_POINT('',(3.23000593275114E-15,17.25,105.5));
#6412=CARTESIAN_POINT('',(-1.29200237310046E-14,105.,105.5));
#6413=CARTESIAN_POINT('Ctrl Pts',(1.93800355965069E-14,17.25,105.5));
#6414=CARTESIAN_POINT('Ctrl Pts',(-43.6995308303616,17.1875,105.5));
#6415=CARTESIAN_POINT('Ctrl Pts',(-74.5997654151808,17.125,74.5997654151808));
#6416=CARTESIAN_POINT('Ctrl Pts',(-105.5,17.0625,43.6995308303616));
#6417=CARTESIAN_POINT('Ctrl Pts',(-105.5,17.,0.));
#6418=CARTESIAN_POINT('Ctrl Pts',(-105.5,16.9375,-43.6995308303615));
#6419=CARTESIAN_POINT('Ctrl Pts',(-74.5997654151808,16.875,-74.5997654151808));
#6420=CARTESIAN_POINT('Ctrl Pts',(-43.6995308303615,16.8125,-105.5));
#6421=CARTESIAN_POINT('Ctrl Pts',(-6.46001186550229E-15,16.75,-105.5));
#6422=CARTESIAN_POINT('Ctrl Pts',(43.6995308303615,16.6875,-105.5));
#6423=CARTESIAN_POINT('Ctrl Pts',(74.5997654151808,16.625,-74.5997654151808));
#6424=CARTESIAN_POINT('Ctrl Pts',(105.5,16.5625,-43.6995308303616));
#6425=CARTESIAN_POINT('Ctrl Pts',(105.5,16.5,-1.29200237310046E-14));
#6426=CARTESIAN_POINT('Ctrl Pts',(105.5,16.4375,43.6995308303615));
#6427=CARTESIAN_POINT('Ctrl Pts',(74.5997654151808,16.375,74.5997654151808));
#6428=CARTESIAN_POINT('Ctrl Pts',(43.6995308303616,16.3125,105.5));
#6429=CARTESIAN_POINT('Ctrl Pts',(1.93800355965069E-14,16.25,105.5));
#6430=CARTESIAN_POINT('Ctrl Pts',(1.93800355965069E-14,17.3750000027312,
105.5));
#6431=CARTESIAN_POINT('Ctrl Pts',(-43.6995308303616,17.3125000027312,105.5));
#6432=CARTESIAN_POINT('Ctrl Pts',(-74.5997654151808,17.2500000027312,74.5997654151808));
#6433=CARTESIAN_POINT('Ctrl Pts',(-105.5,17.1875000027312,43.6995308303616));
#6434=CARTESIAN_POINT('Ctrl Pts',(-105.5,17.1250000027312,0.));
#6435=CARTESIAN_POINT('Ctrl Pts',(-105.5,17.0625000027312,-43.6995308303615));
#6436=CARTESIAN_POINT('Ctrl Pts',(-74.5997654151808,17.0000000027312,-74.5997654151808));
#6437=CARTESIAN_POINT('Ctrl Pts',(-43.6995308303615,16.9375000027312,-105.5));
#6438=CARTESIAN_POINT('Ctrl Pts',(-6.46001186550229E-15,16.8750000027312,
-105.5));
#6439=CARTESIAN_POINT('Ctrl Pts',(43.6995308303615,16.8125000027312,-105.5));
#6440=CARTESIAN_POINT('Ctrl Pts',(74.5997654151808,16.7500000027312,-74.5997654151808));
#6441=CARTESIAN_POINT('Ctrl Pts',(105.5,16.6875000027312,-43.6995308303616));
#6442=CARTESIAN_POINT('Ctrl Pts',(105.5,16.6250000027312,-1.29200237310046E-14));
#6443=CARTESIAN_POINT('Ctrl Pts',(105.5,16.5625000027312,43.6995308303615));
#6444=CARTESIAN_POINT('Ctrl Pts',(74.5997654151808,16.5000000027312,74.5997654151808));
#6445=CARTESIAN_POINT('Ctrl Pts',(43.6995308303616,16.4375000027312,105.5));
#6446=CARTESIAN_POINT('Ctrl Pts',(1.93800355965069E-14,16.3750000027312,
105.5));
#6447=CARTESIAN_POINT('Origin',(0.,105.,0.));
#6448=CARTESIAN_POINT('',(3.23000593275114E-15,18.3750000027312,105.5));
#6449=CARTESIAN_POINT('',(3.23000593275114E-15,18.25,105.5));
#6450=CARTESIAN_POINT('',(-1.29200237310046E-14,105.,105.5));
#6451=CARTESIAN_POINT('Ctrl Pts',(1.93800355965069E-14,18.25,105.5));
#6452=CARTESIAN_POINT('Ctrl Pts',(-43.6995308303616,18.1875,105.5));
#6453=CARTESIAN_POINT('Ctrl Pts',(-74.5997654151808,18.125,74.5997654151808));
#6454=CARTESIAN_POINT('Ctrl Pts',(-105.5,18.0625,43.6995308303616));
#6455=CARTESIAN_POINT('Ctrl Pts',(-105.5,18.,0.));
#6456=CARTESIAN_POINT('Ctrl Pts',(-105.5,17.9375,-43.6995308303615));
#6457=CARTESIAN_POINT('Ctrl Pts',(-74.5997654151808,17.875,-74.5997654151808));
#6458=CARTESIAN_POINT('Ctrl Pts',(-43.6995308303615,17.8125,-105.5));
#6459=CARTESIAN_POINT('Ctrl Pts',(-6.46001186550229E-15,17.75,-105.5));
#6460=CARTESIAN_POINT('Ctrl Pts',(43.6995308303615,17.6875,-105.5));
#6461=CARTESIAN_POINT('Ctrl Pts',(74.5997654151808,17.625,-74.5997654151808));
#6462=CARTESIAN_POINT('Ctrl Pts',(105.5,17.5625,-43.6995308303616));
#6463=CARTESIAN_POINT('Ctrl Pts',(105.5,17.5,-1.29200237310046E-14));
#6464=CARTESIAN_POINT('Ctrl Pts',(105.5,17.4375,43.6995308303615));
#6465=CARTESIAN_POINT('Ctrl Pts',(74.5997654151808,17.375,74.5997654151808));
#6466=CARTESIAN_POINT('Ctrl Pts',(43.6995308303616,17.3125,105.5));
#6467=CARTESIAN_POINT('Ctrl Pts',(1.93800355965069E-14,17.25,105.5));
#6468=CARTESIAN_POINT('Ctrl Pts',(1.93800355965069E-14,18.3750000027312,
105.5));
#6469=CARTESIAN_POINT('Ctrl Pts',(-43.6995308303616,18.3125000027312,105.5));
#6470=CARTESIAN_POINT('Ctrl Pts',(-74.5997654151808,18.2500000027312,74.5997654151808));
#6471=CARTESIAN_POINT('Ctrl Pts',(-105.5,18.1875000027312,43.6995308303616));
#6472=CARTESIAN_POINT('Ctrl Pts',(-105.5,18.1250000027312,0.));
#6473=CARTESIAN_POINT('Ctrl Pts',(-105.5,18.0625000027312,-43.6995308303615));
#6474=CARTESIAN_POINT('Ctrl Pts',(-74.5997654151808,18.0000000027312,-74.5997654151808));
#6475=CARTESIAN_POINT('Ctrl Pts',(-43.6995308303615,17.9375000027312,-105.5));
#6476=CARTESIAN_POINT('Ctrl Pts',(-6.46001186550229E-15,17.8750000027312,
-105.5));
#6477=CARTESIAN_POINT('Ctrl Pts',(43.6995308303615,17.8125000027312,-105.5));
#6478=CARTESIAN_POINT('Ctrl Pts',(74.5997654151808,17.7500000027312,-74.5997654151808));
#6479=CARTESIAN_POINT('Ctrl Pts',(105.5,17.6875000027312,-43.6995308303616));
#6480=CARTESIAN_POINT('Ctrl Pts',(105.5,17.6250000027312,-1.29200237310046E-14));
#6481=CARTESIAN_POINT('Ctrl Pts',(105.5,17.5625000027312,43.6995308303615));
#6482=CARTESIAN_POINT('Ctrl Pts',(74.5997654151808,17.5000000027312,74.5997654151808));
#6483=CARTESIAN_POINT('Ctrl Pts',(43.6995308303616,17.4375000027312,105.5));
#6484=CARTESIAN_POINT('Ctrl Pts',(1.93800355965069E-14,17.3750000027312,
105.5));
#6485=CARTESIAN_POINT('Origin',(0.,105.,0.));
#6486=CARTESIAN_POINT('',(3.23000593275114E-15,19.3750000027312,105.5));
#6487=CARTESIAN_POINT('',(3.23000593275114E-15,19.25,105.5));
#6488=CARTESIAN_POINT('',(-1.29200237310046E-14,105.,105.5));
#6489=CARTESIAN_POINT('Ctrl Pts',(1.93800355965069E-14,19.25,105.5));
#6490=CARTESIAN_POINT('Ctrl Pts',(-43.6995308303616,19.1875,105.5));
#6491=CARTESIAN_POINT('Ctrl Pts',(-74.5997654151808,19.125,74.5997654151808));
#6492=CARTESIAN_POINT('Ctrl Pts',(-105.5,19.0625,43.6995308303616));
#6493=CARTESIAN_POINT('Ctrl Pts',(-105.5,19.,0.));
#6494=CARTESIAN_POINT('Ctrl Pts',(-105.5,18.9375,-43.6995308303615));
#6495=CARTESIAN_POINT('Ctrl Pts',(-74.5997654151808,18.875,-74.5997654151808));
#6496=CARTESIAN_POINT('Ctrl Pts',(-43.6995308303615,18.8125,-105.5));
#6497=CARTESIAN_POINT('Ctrl Pts',(-6.46001186550229E-15,18.75,-105.5));
#6498=CARTESIAN_POINT('Ctrl Pts',(43.6995308303615,18.6875,-105.5));
#6499=CARTESIAN_POINT('Ctrl Pts',(74.5997654151808,18.625,-74.5997654151808));
#6500=CARTESIAN_POINT('Ctrl Pts',(105.5,18.5625,-43.6995308303616));
#6501=CARTESIAN_POINT('Ctrl Pts',(105.5,18.5,-1.29200237310046E-14));
#6502=CARTESIAN_POINT('Ctrl Pts',(105.5,18.4375,43.6995308303615));
#6503=CARTESIAN_POINT('Ctrl Pts',(74.5997654151808,18.375,74.5997654151808));
#6504=CARTESIAN_POINT('Ctrl Pts',(43.6995308303616,18.3125,105.5));
#6505=CARTESIAN_POINT('Ctrl Pts',(1.93800355965069E-14,18.25,105.5));
#6506=CARTESIAN_POINT('Ctrl Pts',(1.93800355965069E-14,19.3750000027312,
105.5));
#6507=CARTESIAN_POINT('Ctrl Pts',(-43.6995308303616,19.3125000027312,105.5));
#6508=CARTESIAN_POINT('Ctrl Pts',(-74.5997654151808,19.2500000027312,74.5997654151808));
#6509=CARTESIAN_POINT('Ctrl Pts',(-105.5,19.1875000027312,43.6995308303616));
#6510=CARTESIAN_POINT('Ctrl Pts',(-105.5,19.1250000027312,0.));
#6511=CARTESIAN_POINT('Ctrl Pts',(-105.5,19.0625000027312,-43.6995308303615));
#6512=CARTESIAN_POINT('Ctrl Pts',(-74.5997654151808,19.0000000027312,-74.5997654151808));
#6513=CARTESIAN_POINT('Ctrl Pts',(-43.6995308303615,18.9375000027312,-105.5));
#6514=CARTESIAN_POINT('Ctrl Pts',(-6.46001186550229E-15,18.8750000027312,
-105.5));
#6515=CARTESIAN_POINT('Ctrl Pts',(43.6995308303615,18.8125000027312,-105.5));
#6516=CARTESIAN_POINT('Ctrl Pts',(74.5997654151808,18.7500000027312,-74.5997654151808));
#6517=CARTESIAN_POINT('Ctrl Pts',(105.5,18.6875000027312,-43.6995308303616));
#6518=CARTESIAN_POINT('Ctrl Pts',(105.5,18.6250000027312,-1.29200237310046E-14));
#6519=CARTESIAN_POINT('Ctrl Pts',(105.5,18.5625000027312,43.6995308303615));
#6520=CARTESIAN_POINT('Ctrl Pts',(74.5997654151808,18.5000000027312,74.5997654151808));
#6521=CARTESIAN_POINT('Ctrl Pts',(43.6995308303616,18.4375000027312,105.5));
#6522=CARTESIAN_POINT('Ctrl Pts',(1.93800355965069E-14,18.3750000027312,
105.5));
#6523=CARTESIAN_POINT('Origin',(0.,105.,0.));
#6524=CARTESIAN_POINT('',(3.23000593275114E-15,20.3750000027312,105.5));
#6525=CARTESIAN_POINT('',(3.23000593275114E-15,20.25,105.5));
#6526=CARTESIAN_POINT('',(-1.29200237310046E-14,105.,105.5));
#6527=CARTESIAN_POINT('Ctrl Pts',(1.93800355965069E-14,20.25,105.5));
#6528=CARTESIAN_POINT('Ctrl Pts',(-43.6995308303616,20.1875,105.5));
#6529=CARTESIAN_POINT('Ctrl Pts',(-74.5997654151808,20.125,74.5997654151808));
#6530=CARTESIAN_POINT('Ctrl Pts',(-105.5,20.0625,43.6995308303616));
#6531=CARTESIAN_POINT('Ctrl Pts',(-105.5,20.,0.));
#6532=CARTESIAN_POINT('Ctrl Pts',(-105.5,19.9375,-43.6995308303615));
#6533=CARTESIAN_POINT('Ctrl Pts',(-74.5997654151808,19.875,-74.5997654151808));
#6534=CARTESIAN_POINT('Ctrl Pts',(-43.6995308303615,19.8125,-105.5));
#6535=CARTESIAN_POINT('Ctrl Pts',(-6.46001186550229E-15,19.75,-105.5));
#6536=CARTESIAN_POINT('Ctrl Pts',(43.6995308303615,19.6875,-105.5));
#6537=CARTESIAN_POINT('Ctrl Pts',(74.5997654151808,19.625,-74.5997654151808));
#6538=CARTESIAN_POINT('Ctrl Pts',(105.5,19.5625,-43.6995308303616));
#6539=CARTESIAN_POINT('Ctrl Pts',(105.5,19.5,-1.29200237310046E-14));
#6540=CARTESIAN_POINT('Ctrl Pts',(105.5,19.4375,43.6995308303615));
#6541=CARTESIAN_POINT('Ctrl Pts',(74.5997654151808,19.375,74.5997654151808));
#6542=CARTESIAN_POINT('Ctrl Pts',(43.6995308303616,19.3125,105.5));
#6543=CARTESIAN_POINT('Ctrl Pts',(1.93800355965069E-14,19.25,105.5));
#6544=CARTESIAN_POINT('Ctrl Pts',(1.93800355965069E-14,20.3750000027312,
105.5));
#6545=CARTESIAN_POINT('Ctrl Pts',(-43.6995308303616,20.3125000027312,105.5));
#6546=CARTESIAN_POINT('Ctrl Pts',(-74.5997654151808,20.2500000027312,74.5997654151808));
#6547=CARTESIAN_POINT('Ctrl Pts',(-105.5,20.1875000027312,43.6995308303616));
#6548=CARTESIAN_POINT('Ctrl Pts',(-105.5,20.1250000027312,0.));
#6549=CARTESIAN_POINT('Ctrl Pts',(-105.5,20.0625000027312,-43.6995308303615));
#6550=CARTESIAN_POINT('Ctrl Pts',(-74.5997654151808,20.0000000027312,-74.5997654151808));
#6551=CARTESIAN_POINT('Ctrl Pts',(-43.6995308303615,19.9375000027312,-105.5));
#6552=CARTESIAN_POINT('Ctrl Pts',(-6.46001186550229E-15,19.8750000027312,
-105.5));
#6553=CARTESIAN_POINT('Ctrl Pts',(43.6995308303615,19.8125000027312,-105.5));
#6554=CARTESIAN_POINT('Ctrl Pts',(74.5997654151808,19.7500000027312,-74.5997654151808));
#6555=CARTESIAN_POINT('Ctrl Pts',(105.5,19.6875000027312,-43.6995308303616));
#6556=CARTESIAN_POINT('Ctrl Pts',(105.5,19.6250000027312,-1.29200237310046E-14));
#6557=CARTESIAN_POINT('Ctrl Pts',(105.5,19.5625000027312,43.6995308303615));
#6558=CARTESIAN_POINT('Ctrl Pts',(74.5997654151808,19.5000000027312,74.5997654151808));
#6559=CARTESIAN_POINT('Ctrl Pts',(43.6995308303616,19.4375000027312,105.5));
#6560=CARTESIAN_POINT('Ctrl Pts',(1.93800355965069E-14,19.3750000027312,
105.5));
#6561=CARTESIAN_POINT('Origin',(0.,105.,0.));
#6562=CARTESIAN_POINT('',(3.23000593275114E-15,21.3750000027312,105.5));
#6563=CARTESIAN_POINT('',(3.23000593275114E-15,21.25,105.5));
#6564=CARTESIAN_POINT('',(-1.29200237310046E-14,105.,105.5));
#6565=CARTESIAN_POINT('Ctrl Pts',(1.93800355965069E-14,21.25,105.5));
#6566=CARTESIAN_POINT('Ctrl Pts',(-43.6995308303616,21.1875,105.5));
#6567=CARTESIAN_POINT('Ctrl Pts',(-74.5997654151808,21.125,74.5997654151808));
#6568=CARTESIAN_POINT('Ctrl Pts',(-105.5,21.0625,43.6995308303616));
#6569=CARTESIAN_POINT('Ctrl Pts',(-105.5,21.,0.));
#6570=CARTESIAN_POINT('Ctrl Pts',(-105.5,20.9375,-43.6995308303615));
#6571=CARTESIAN_POINT('Ctrl Pts',(-74.5997654151808,20.875,-74.5997654151808));
#6572=CARTESIAN_POINT('Ctrl Pts',(-43.6995308303615,20.8125,-105.5));
#6573=CARTESIAN_POINT('Ctrl Pts',(-6.46001186550229E-15,20.75,-105.5));
#6574=CARTESIAN_POINT('Ctrl Pts',(43.6995308303615,20.6875,-105.5));
#6575=CARTESIAN_POINT('Ctrl Pts',(74.5997654151808,20.625,-74.5997654151808));
#6576=CARTESIAN_POINT('Ctrl Pts',(105.5,20.5625,-43.6995308303616));
#6577=CARTESIAN_POINT('Ctrl Pts',(105.5,20.5,-1.29200237310046E-14));
#6578=CARTESIAN_POINT('Ctrl Pts',(105.5,20.4375,43.6995308303615));
#6579=CARTESIAN_POINT('Ctrl Pts',(74.5997654151808,20.375,74.5997654151808));
#6580=CARTESIAN_POINT('Ctrl Pts',(43.6995308303616,20.3125,105.5));
#6581=CARTESIAN_POINT('Ctrl Pts',(1.93800355965069E-14,20.25,105.5));
#6582=CARTESIAN_POINT('Ctrl Pts',(1.93800355965069E-14,21.3750000027312,
105.5));
#6583=CARTESIAN_POINT('Ctrl Pts',(-43.6995308303616,21.3125000027312,105.5));
#6584=CARTESIAN_POINT('Ctrl Pts',(-74.5997654151808,21.2500000027312,74.5997654151808));
#6585=CARTESIAN_POINT('Ctrl Pts',(-105.5,21.1875000027312,43.6995308303616));
#6586=CARTESIAN_POINT('Ctrl Pts',(-105.5,21.1250000027312,0.));
#6587=CARTESIAN_POINT('Ctrl Pts',(-105.5,21.0625000027312,-43.6995308303615));
#6588=CARTESIAN_POINT('Ctrl Pts',(-74.5997654151808,21.0000000027312,-74.5997654151808));
#6589=CARTESIAN_POINT('Ctrl Pts',(-43.6995308303615,20.9375000027312,-105.5));
#6590=CARTESIAN_POINT('Ctrl Pts',(-6.46001186550229E-15,20.8750000027312,
-105.5));
#6591=CARTESIAN_POINT('Ctrl Pts',(43.6995308303615,20.8125000027312,-105.5));
#6592=CARTESIAN_POINT('Ctrl Pts',(74.5997654151808,20.7500000027312,-74.5997654151808));
#6593=CARTESIAN_POINT('Ctrl Pts',(105.5,20.6875000027312,-43.6995308303616));
#6594=CARTESIAN_POINT('Ctrl Pts',(105.5,20.6250000027312,-1.29200237310046E-14));
#6595=CARTESIAN_POINT('Ctrl Pts',(105.5,20.5625000027312,43.6995308303615));
#6596=CARTESIAN_POINT('Ctrl Pts',(74.5997654151808,20.5000000027312,74.5997654151808));
#6597=CARTESIAN_POINT('Ctrl Pts',(43.6995308303616,20.4375000027312,105.5));
#6598=CARTESIAN_POINT('Ctrl Pts',(1.93800355965069E-14,20.3750000027312,
105.5));
#6599=CARTESIAN_POINT('Origin',(0.,105.,0.));
#6600=CARTESIAN_POINT('',(3.23000593275114E-15,22.3750000027312,105.5));
#6601=CARTESIAN_POINT('',(3.23000593275114E-15,22.25,105.5));
#6602=CARTESIAN_POINT('',(-1.29200237310046E-14,105.,105.5));
#6603=CARTESIAN_POINT('Ctrl Pts',(1.93800355965069E-14,22.25,105.5));
#6604=CARTESIAN_POINT('Ctrl Pts',(-43.6995308303616,22.1875,105.5));
#6605=CARTESIAN_POINT('Ctrl Pts',(-74.5997654151808,22.125,74.5997654151808));
#6606=CARTESIAN_POINT('Ctrl Pts',(-105.5,22.0625,43.6995308303616));
#6607=CARTESIAN_POINT('Ctrl Pts',(-105.5,22.,0.));
#6608=CARTESIAN_POINT('Ctrl Pts',(-105.5,21.9375,-43.6995308303615));
#6609=CARTESIAN_POINT('Ctrl Pts',(-74.5997654151808,21.875,-74.5997654151808));
#6610=CARTESIAN_POINT('Ctrl Pts',(-43.6995308303615,21.8125,-105.5));
#6611=CARTESIAN_POINT('Ctrl Pts',(-6.46001186550229E-15,21.75,-105.5));
#6612=CARTESIAN_POINT('Ctrl Pts',(43.6995308303615,21.6875,-105.5));
#6613=CARTESIAN_POINT('Ctrl Pts',(74.5997654151808,21.625,-74.5997654151808));
#6614=CARTESIAN_POINT('Ctrl Pts',(105.5,21.5625,-43.6995308303616));
#6615=CARTESIAN_POINT('Ctrl Pts',(105.5,21.5,-1.29200237310046E-14));
#6616=CARTESIAN_POINT('Ctrl Pts',(105.5,21.4375,43.6995308303615));
#6617=CARTESIAN_POINT('Ctrl Pts',(74.5997654151808,21.375,74.5997654151808));
#6618=CARTESIAN_POINT('Ctrl Pts',(43.6995308303616,21.3125,105.5));
#6619=CARTESIAN_POINT('Ctrl Pts',(1.93800355965069E-14,21.25,105.5));
#6620=CARTESIAN_POINT('Ctrl Pts',(1.93800355965069E-14,22.3750000027312,
105.5));
#6621=CARTESIAN_POINT('Ctrl Pts',(-43.6995308303616,22.3125000027312,105.5));
#6622=CARTESIAN_POINT('Ctrl Pts',(-74.5997654151808,22.2500000027312,74.5997654151808));
#6623=CARTESIAN_POINT('Ctrl Pts',(-105.5,22.1875000027312,43.6995308303616));
#6624=CARTESIAN_POINT('Ctrl Pts',(-105.5,22.1250000027312,0.));
#6625=CARTESIAN_POINT('Ctrl Pts',(-105.5,22.0625000027312,-43.6995308303615));
#6626=CARTESIAN_POINT('Ctrl Pts',(-74.5997654151808,22.0000000027312,-74.5997654151808));
#6627=CARTESIAN_POINT('Ctrl Pts',(-43.6995308303615,21.9375000027312,-105.5));
#6628=CARTESIAN_POINT('Ctrl Pts',(-6.46001186550229E-15,21.8750000027312,
-105.5));
#6629=CARTESIAN_POINT('Ctrl Pts',(43.6995308303615,21.8125000027312,-105.5));
#6630=CARTESIAN_POINT('Ctrl Pts',(74.5997654151808,21.7500000027312,-74.5997654151808));
#6631=CARTESIAN_POINT('Ctrl Pts',(105.5,21.6875000027312,-43.6995308303616));
#6632=CARTESIAN_POINT('Ctrl Pts',(105.5,21.6250000027312,-1.29200237310046E-14));
#6633=CARTESIAN_POINT('Ctrl Pts',(105.5,21.5625000027312,43.6995308303615));
#6634=CARTESIAN_POINT('Ctrl Pts',(74.5997654151808,21.5000000027312,74.5997654151808));
#6635=CARTESIAN_POINT('Ctrl Pts',(43.6995308303616,21.4375000027312,105.5));
#6636=CARTESIAN_POINT('Ctrl Pts',(1.93800355965069E-14,21.3750000027312,
105.5));
#6637=CARTESIAN_POINT('Origin',(0.,105.,0.));
#6638=CARTESIAN_POINT('',(3.23000593275114E-15,23.3750000027312,105.5));
#6639=CARTESIAN_POINT('',(3.23000593275114E-15,23.25,105.5));
#6640=CARTESIAN_POINT('',(-1.29200237310046E-14,105.,105.5));
#6641=CARTESIAN_POINT('Ctrl Pts',(1.93800355965069E-14,23.25,105.5));
#6642=CARTESIAN_POINT('Ctrl Pts',(-43.6995308303616,23.1875,105.5));
#6643=CARTESIAN_POINT('Ctrl Pts',(-74.5997654151808,23.125,74.5997654151808));
#6644=CARTESIAN_POINT('Ctrl Pts',(-105.5,23.0625,43.6995308303616));
#6645=CARTESIAN_POINT('Ctrl Pts',(-105.5,23.,0.));
#6646=CARTESIAN_POINT('Ctrl Pts',(-105.5,22.9375,-43.6995308303615));
#6647=CARTESIAN_POINT('Ctrl Pts',(-74.5997654151808,22.875,-74.5997654151808));
#6648=CARTESIAN_POINT('Ctrl Pts',(-43.6995308303615,22.8125,-105.5));
#6649=CARTESIAN_POINT('Ctrl Pts',(-6.46001186550229E-15,22.75,-105.5));
#6650=CARTESIAN_POINT('Ctrl Pts',(43.6995308303615,22.6875,-105.5));
#6651=CARTESIAN_POINT('Ctrl Pts',(74.5997654151808,22.625,-74.5997654151808));
#6652=CARTESIAN_POINT('Ctrl Pts',(105.5,22.5625,-43.6995308303616));
#6653=CARTESIAN_POINT('Ctrl Pts',(105.5,22.5,-1.29200237310046E-14));
#6654=CARTESIAN_POINT('Ctrl Pts',(105.5,22.4375,43.6995308303615));
#6655=CARTESIAN_POINT('Ctrl Pts',(74.5997654151808,22.375,74.5997654151808));
#6656=CARTESIAN_POINT('Ctrl Pts',(43.6995308303616,22.3125,105.5));
#6657=CARTESIAN_POINT('Ctrl Pts',(1.93800355965069E-14,22.25,105.5));
#6658=CARTESIAN_POINT('Ctrl Pts',(1.93800355965069E-14,23.3750000027312,
105.5));
#6659=CARTESIAN_POINT('Ctrl Pts',(-43.6995308303616,23.3125000027312,105.5));
#6660=CARTESIAN_POINT('Ctrl Pts',(-74.5997654151808,23.2500000027312,74.5997654151808));
#6661=CARTESIAN_POINT('Ctrl Pts',(-105.5,23.1875000027312,43.6995308303616));
#6662=CARTESIAN_POINT('Ctrl Pts',(-105.5,23.1250000027312,0.));
#6663=CARTESIAN_POINT('Ctrl Pts',(-105.5,23.0625000027312,-43.6995308303615));
#6664=CARTESIAN_POINT('Ctrl Pts',(-74.5997654151808,23.0000000027312,-74.5997654151808));
#6665=CARTESIAN_POINT('Ctrl Pts',(-43.6995308303615,22.9375000027312,-105.5));
#6666=CARTESIAN_POINT('Ctrl Pts',(-6.46001186550229E-15,22.8750000027312,
-105.5));
#6667=CARTESIAN_POINT('Ctrl Pts',(43.6995308303615,22.8125000027312,-105.5));
#6668=CARTESIAN_POINT('Ctrl Pts',(74.5997654151808,22.7500000027312,-74.5997654151808));
#6669=CARTESIAN_POINT('Ctrl Pts',(105.5,22.6875000027312,-43.6995308303616));
#6670=CARTESIAN_POINT('Ctrl Pts',(105.5,22.6250000027312,-1.29200237310046E-14));
#6671=CARTESIAN_POINT('Ctrl Pts',(105.5,22.5625000027312,43.6995308303615));
#6672=CARTESIAN_POINT('Ctrl Pts',(74.5997654151808,22.5000000027312,74.5997654151808));
#6673=CARTESIAN_POINT('Ctrl Pts',(43.6995308303616,22.4375000027312,105.5));
#6674=CARTESIAN_POINT('Ctrl Pts',(1.93800355965069E-14,22.3750000027312,
105.5));
#6675=CARTESIAN_POINT('Origin',(0.,105.,0.));
#6676=CARTESIAN_POINT('',(3.23000593275114E-15,24.3750000027312,105.5));
#6677=CARTESIAN_POINT('',(3.23000593275114E-15,24.25,105.5));
#6678=CARTESIAN_POINT('',(-1.29200237310046E-14,105.,105.5));
#6679=CARTESIAN_POINT('Ctrl Pts',(1.93800355965069E-14,24.25,105.5));
#6680=CARTESIAN_POINT('Ctrl Pts',(-43.6995308303616,24.1875,105.5));
#6681=CARTESIAN_POINT('Ctrl Pts',(-74.5997654151808,24.125,74.5997654151808));
#6682=CARTESIAN_POINT('Ctrl Pts',(-105.5,24.0625,43.6995308303616));
#6683=CARTESIAN_POINT('Ctrl Pts',(-105.5,24.,0.));
#6684=CARTESIAN_POINT('Ctrl Pts',(-105.5,23.9375,-43.6995308303615));
#6685=CARTESIAN_POINT('Ctrl Pts',(-74.5997654151808,23.875,-74.5997654151808));
#6686=CARTESIAN_POINT('Ctrl Pts',(-43.6995308303615,23.8125,-105.5));
#6687=CARTESIAN_POINT('Ctrl Pts',(-6.46001186550229E-15,23.75,-105.5));
#6688=CARTESIAN_POINT('Ctrl Pts',(43.6995308303615,23.6875,-105.5));
#6689=CARTESIAN_POINT('Ctrl Pts',(74.5997654151808,23.625,-74.5997654151808));
#6690=CARTESIAN_POINT('Ctrl Pts',(105.5,23.5625,-43.6995308303616));
#6691=CARTESIAN_POINT('Ctrl Pts',(105.5,23.5,-1.29200237310046E-14));
#6692=CARTESIAN_POINT('Ctrl Pts',(105.5,23.4375,43.6995308303615));
#6693=CARTESIAN_POINT('Ctrl Pts',(74.5997654151808,23.375,74.5997654151808));
#6694=CARTESIAN_POINT('Ctrl Pts',(43.6995308303616,23.3125,105.5));
#6695=CARTESIAN_POINT('Ctrl Pts',(1.93800355965069E-14,23.25,105.5));
#6696=CARTESIAN_POINT('Ctrl Pts',(1.93800355965069E-14,24.3750000027312,
105.5));
#6697=CARTESIAN_POINT('Ctrl Pts',(-43.6995308303616,24.3125000027312,105.5));
#6698=CARTESIAN_POINT('Ctrl Pts',(-74.5997654151808,24.2500000027312,74.5997654151808));
#6699=CARTESIAN_POINT('Ctrl Pts',(-105.5,24.1875000027312,43.6995308303616));
#6700=CARTESIAN_POINT('Ctrl Pts',(-105.5,24.1250000027312,0.));
#6701=CARTESIAN_POINT('Ctrl Pts',(-105.5,24.0625000027312,-43.6995308303615));
#6702=CARTESIAN_POINT('Ctrl Pts',(-74.5997654151808,24.0000000027312,-74.5997654151808));
#6703=CARTESIAN_POINT('Ctrl Pts',(-43.6995308303615,23.9375000027312,-105.5));
#6704=CARTESIAN_POINT('Ctrl Pts',(-6.46001186550229E-15,23.8750000027312,
-105.5));
#6705=CARTESIAN_POINT('Ctrl Pts',(43.6995308303615,23.8125000027312,-105.5));
#6706=CARTESIAN_POINT('Ctrl Pts',(74.5997654151808,23.7500000027312,-74.5997654151808));
#6707=CARTESIAN_POINT('Ctrl Pts',(105.5,23.6875000027312,-43.6995308303616));
#6708=CARTESIAN_POINT('Ctrl Pts',(105.5,23.6250000027312,-1.29200237310046E-14));
#6709=CARTESIAN_POINT('Ctrl Pts',(105.5,23.5625000027312,43.6995308303615));
#6710=CARTESIAN_POINT('Ctrl Pts',(74.5997654151808,23.5000000027312,74.5997654151808));
#6711=CARTESIAN_POINT('Ctrl Pts',(43.6995308303616,23.4375000027312,105.5));
#6712=CARTESIAN_POINT('Ctrl Pts',(1.93800355965069E-14,23.3750000027312,
105.5));
#6713=CARTESIAN_POINT('Origin',(0.,105.,0.));
#6714=CARTESIAN_POINT('',(3.23000593275114E-15,25.3750000027312,105.5));
#6715=CARTESIAN_POINT('',(3.23000593275114E-15,25.25,105.5));
#6716=CARTESIAN_POINT('',(-1.29200237310046E-14,105.,105.5));
#6717=CARTESIAN_POINT('Ctrl Pts',(1.93800355965069E-14,25.25,105.5));
#6718=CARTESIAN_POINT('Ctrl Pts',(-43.6995308303616,25.1875,105.5));
#6719=CARTESIAN_POINT('Ctrl Pts',(-74.5997654151808,25.125,74.5997654151808));
#6720=CARTESIAN_POINT('Ctrl Pts',(-105.5,25.0625,43.6995308303616));
#6721=CARTESIAN_POINT('Ctrl Pts',(-105.5,25.,0.));
#6722=CARTESIAN_POINT('Ctrl Pts',(-105.5,24.9375,-43.6995308303615));
#6723=CARTESIAN_POINT('Ctrl Pts',(-74.5997654151808,24.875,-74.5997654151808));
#6724=CARTESIAN_POINT('Ctrl Pts',(-43.6995308303615,24.8125,-105.5));
#6725=CARTESIAN_POINT('Ctrl Pts',(-6.46001186550229E-15,24.75,-105.5));
#6726=CARTESIAN_POINT('Ctrl Pts',(43.6995308303615,24.6875,-105.5));
#6727=CARTESIAN_POINT('Ctrl Pts',(74.5997654151808,24.625,-74.5997654151808));
#6728=CARTESIAN_POINT('Ctrl Pts',(105.5,24.5625,-43.6995308303616));
#6729=CARTESIAN_POINT('Ctrl Pts',(105.5,24.5,-1.29200237310046E-14));
#6730=CARTESIAN_POINT('Ctrl Pts',(105.5,24.4375,43.6995308303615));
#6731=CARTESIAN_POINT('Ctrl Pts',(74.5997654151808,24.375,74.5997654151808));
#6732=CARTESIAN_POINT('Ctrl Pts',(43.6995308303616,24.3125,105.5));
#6733=CARTESIAN_POINT('Ctrl Pts',(1.93800355965069E-14,24.25,105.5));
#6734=CARTESIAN_POINT('Ctrl Pts',(1.93800355965069E-14,25.3750000027312,
105.5));
#6735=CARTESIAN_POINT('Ctrl Pts',(-43.6995308303616,25.3125000027312,105.5));
#6736=CARTESIAN_POINT('Ctrl Pts',(-74.5997654151808,25.2500000027312,74.5997654151808));
#6737=CARTESIAN_POINT('Ctrl Pts',(-105.5,25.1875000027312,43.6995308303616));
#6738=CARTESIAN_POINT('Ctrl Pts',(-105.5,25.1250000027312,0.));
#6739=CARTESIAN_POINT('Ctrl Pts',(-105.5,25.0625000027312,-43.6995308303615));
#6740=CARTESIAN_POINT('Ctrl Pts',(-74.5997654151808,25.0000000027312,-74.5997654151808));
#6741=CARTESIAN_POINT('Ctrl Pts',(-43.6995308303615,24.9375000027312,-105.5));
#6742=CARTESIAN_POINT('Ctrl Pts',(-6.46001186550229E-15,24.8750000027312,
-105.5));
#6743=CARTESIAN_POINT('Ctrl Pts',(43.6995308303615,24.8125000027312,-105.5));
#6744=CARTESIAN_POINT('Ctrl Pts',(74.5997654151808,24.7500000027312,-74.5997654151808));
#6745=CARTESIAN_POINT('Ctrl Pts',(105.5,24.6875000027312,-43.6995308303616));
#6746=CARTESIAN_POINT('Ctrl Pts',(105.5,24.6250000027312,-1.29200237310046E-14));
#6747=CARTESIAN_POINT('Ctrl Pts',(105.5,24.5625000027312,43.6995308303615));
#6748=CARTESIAN_POINT('Ctrl Pts',(74.5997654151808,24.5000000027312,74.5997654151808));
#6749=CARTESIAN_POINT('Ctrl Pts',(43.6995308303616,24.4375000027312,105.5));
#6750=CARTESIAN_POINT('Ctrl Pts',(1.93800355965069E-14,24.3750000027312,
105.5));
#6751=CARTESIAN_POINT('Origin',(0.,105.,0.));
#6752=CARTESIAN_POINT('',(3.23000593275114E-15,26.3750000027312,105.5));
#6753=CARTESIAN_POINT('',(3.23000593275114E-15,26.25,105.5));
#6754=CARTESIAN_POINT('',(-1.29200237310046E-14,105.,105.5));
#6755=CARTESIAN_POINT('Ctrl Pts',(1.93800355965069E-14,26.25,105.5));
#6756=CARTESIAN_POINT('Ctrl Pts',(-43.6995308303616,26.1875,105.5));
#6757=CARTESIAN_POINT('Ctrl Pts',(-74.5997654151808,26.125,74.5997654151808));
#6758=CARTESIAN_POINT('Ctrl Pts',(-105.5,26.0625,43.6995308303616));
#6759=CARTESIAN_POINT('Ctrl Pts',(-105.5,26.,0.));
#6760=CARTESIAN_POINT('Ctrl Pts',(-105.5,25.9375,-43.6995308303615));
#6761=CARTESIAN_POINT('Ctrl Pts',(-74.5997654151808,25.875,-74.5997654151808));
#6762=CARTESIAN_POINT('Ctrl Pts',(-43.6995308303615,25.8125,-105.5));
#6763=CARTESIAN_POINT('Ctrl Pts',(-6.46001186550229E-15,25.75,-105.5));
#6764=CARTESIAN_POINT('Ctrl Pts',(43.6995308303615,25.6875,-105.5));
#6765=CARTESIAN_POINT('Ctrl Pts',(74.5997654151808,25.625,-74.5997654151808));
#6766=CARTESIAN_POINT('Ctrl Pts',(105.5,25.5625,-43.6995308303616));
#6767=CARTESIAN_POINT('Ctrl Pts',(105.5,25.5,-1.29200237310046E-14));
#6768=CARTESIAN_POINT('Ctrl Pts',(105.5,25.4375,43.6995308303615));
#6769=CARTESIAN_POINT('Ctrl Pts',(74.5997654151808,25.375,74.5997654151808));
#6770=CARTESIAN_POINT('Ctrl Pts',(43.6995308303616,25.3125,105.5));
#6771=CARTESIAN_POINT('Ctrl Pts',(1.93800355965069E-14,25.25,105.5));
#6772=CARTESIAN_POINT('Ctrl Pts',(1.93800355965069E-14,26.3750000027312,
105.5));
#6773=CARTESIAN_POINT('Ctrl Pts',(-43.6995308303616,26.3125000027312,105.5));
#6774=CARTESIAN_POINT('Ctrl Pts',(-74.5997654151808,26.2500000027312,74.5997654151808));
#6775=CARTESIAN_POINT('Ctrl Pts',(-105.5,26.1875000027312,43.6995308303616));
#6776=CARTESIAN_POINT('Ctrl Pts',(-105.5,26.1250000027312,0.));
#6777=CARTESIAN_POINT('Ctrl Pts',(-105.5,26.0625000027312,-43.6995308303615));
#6778=CARTESIAN_POINT('Ctrl Pts',(-74.5997654151808,26.0000000027312,-74.5997654151808));
#6779=CARTESIAN_POINT('Ctrl Pts',(-43.6995308303615,25.9375000027312,-105.5));
#6780=CARTESIAN_POINT('Ctrl Pts',(-6.46001186550229E-15,25.8750000027312,
-105.5));
#6781=CARTESIAN_POINT('Ctrl Pts',(43.6995308303615,25.8125000027312,-105.5));
#6782=CARTESIAN_POINT('Ctrl Pts',(74.5997654151808,25.7500000027312,-74.5997654151808));
#6783=CARTESIAN_POINT('Ctrl Pts',(105.5,25.6875000027312,-43.6995308303616));
#6784=CARTESIAN_POINT('Ctrl Pts',(105.5,25.6250000027312,-1.29200237310046E-14));
#6785=CARTESIAN_POINT('Ctrl Pts',(105.5,25.5625000027312,43.6995308303615));
#6786=CARTESIAN_POINT('Ctrl Pts',(74.5997654151808,25.5000000027312,74.5997654151808));
#6787=CARTESIAN_POINT('Ctrl Pts',(43.6995308303616,25.4375000027312,105.5));
#6788=CARTESIAN_POINT('Ctrl Pts',(1.93800355965069E-14,25.3750000027312,
105.5));
#6789=CARTESIAN_POINT('Origin',(0.,105.,0.));
#6790=CARTESIAN_POINT('',(3.23000593275114E-15,27.3750000027312,105.5));
#6791=CARTESIAN_POINT('',(3.23000593275114E-15,27.25,105.5));
#6792=CARTESIAN_POINT('',(-1.29200237310046E-14,105.,105.5));
#6793=CARTESIAN_POINT('Ctrl Pts',(1.93800355965069E-14,27.25,105.5));
#6794=CARTESIAN_POINT('Ctrl Pts',(-43.6995308303616,27.1875,105.5));
#6795=CARTESIAN_POINT('Ctrl Pts',(-74.5997654151808,27.125,74.5997654151808));
#6796=CARTESIAN_POINT('Ctrl Pts',(-105.5,27.0625,43.6995308303616));
#6797=CARTESIAN_POINT('Ctrl Pts',(-105.5,27.,0.));
#6798=CARTESIAN_POINT('Ctrl Pts',(-105.5,26.9375,-43.6995308303615));
#6799=CARTESIAN_POINT('Ctrl Pts',(-74.5997654151808,26.875,-74.5997654151808));
#6800=CARTESIAN_POINT('Ctrl Pts',(-43.6995308303615,26.8125,-105.5));
#6801=CARTESIAN_POINT('Ctrl Pts',(-6.46001186550229E-15,26.75,-105.5));
#6802=CARTESIAN_POINT('Ctrl Pts',(43.6995308303615,26.6875,-105.5));
#6803=CARTESIAN_POINT('Ctrl Pts',(74.5997654151808,26.625,-74.5997654151808));
#6804=CARTESIAN_POINT('Ctrl Pts',(105.5,26.5625,-43.6995308303616));
#6805=CARTESIAN_POINT('Ctrl Pts',(105.5,26.5,-1.29200237310046E-14));
#6806=CARTESIAN_POINT('Ctrl Pts',(105.5,26.4375,43.6995308303615));
#6807=CARTESIAN_POINT('Ctrl Pts',(74.5997654151808,26.375,74.5997654151808));
#6808=CARTESIAN_POINT('Ctrl Pts',(43.6995308303616,26.3125,105.5));
#6809=CARTESIAN_POINT('Ctrl Pts',(1.93800355965069E-14,26.25,105.5));
#6810=CARTESIAN_POINT('Ctrl Pts',(1.93800355965069E-14,27.3750000027312,
105.5));
#6811=CARTESIAN_POINT('Ctrl Pts',(-43.6995308303616,27.3125000027312,105.5));
#6812=CARTESIAN_POINT('Ctrl Pts',(-74.5997654151808,27.2500000027312,74.5997654151808));
#6813=CARTESIAN_POINT('Ctrl Pts',(-105.5,27.1875000027312,43.6995308303616));
#6814=CARTESIAN_POINT('Ctrl Pts',(-105.5,27.1250000027312,0.));
#6815=CARTESIAN_POINT('Ctrl Pts',(-105.5,27.0625000027312,-43.6995308303615));
#6816=CARTESIAN_POINT('Ctrl Pts',(-74.5997654151808,27.0000000027312,-74.5997654151808));
#6817=CARTESIAN_POINT('Ctrl Pts',(-43.6995308303615,26.9375000027312,-105.5));
#6818=CARTESIAN_POINT('Ctrl Pts',(-6.46001186550229E-15,26.8750000027312,
-105.5));
#6819=CARTESIAN_POINT('Ctrl Pts',(43.6995308303615,26.8125000027312,-105.5));
#6820=CARTESIAN_POINT('Ctrl Pts',(74.5997654151808,26.7500000027312,-74.5997654151808));
#6821=CARTESIAN_POINT('Ctrl Pts',(105.5,26.6875000027312,-43.6995308303616));
#6822=CARTESIAN_POINT('Ctrl Pts',(105.5,26.6250000027312,-1.29200237310046E-14));
#6823=CARTESIAN_POINT('Ctrl Pts',(105.5,26.5625000027312,43.6995308303615));
#6824=CARTESIAN_POINT('Ctrl Pts',(74.5997654151808,26.5000000027312,74.5997654151808));
#6825=CARTESIAN_POINT('Ctrl Pts',(43.6995308303616,26.4375000027312,105.5));
#6826=CARTESIAN_POINT('Ctrl Pts',(1.93800355965069E-14,26.3750000027312,
105.5));
#6827=CARTESIAN_POINT('Origin',(0.,105.,0.));
#6828=CARTESIAN_POINT('',(3.23000593275114E-15,28.3750000027312,105.5));
#6829=CARTESIAN_POINT('',(3.23000593275114E-15,28.25,105.5));
#6830=CARTESIAN_POINT('',(-1.29200237310046E-14,105.,105.5));
#6831=CARTESIAN_POINT('Ctrl Pts',(1.93800355965069E-14,28.25,105.5));
#6832=CARTESIAN_POINT('Ctrl Pts',(-43.6995308303616,28.1875,105.5));
#6833=CARTESIAN_POINT('Ctrl Pts',(-74.5997654151808,28.125,74.5997654151808));
#6834=CARTESIAN_POINT('Ctrl Pts',(-105.5,28.0625,43.6995308303616));
#6835=CARTESIAN_POINT('Ctrl Pts',(-105.5,28.,0.));
#6836=CARTESIAN_POINT('Ctrl Pts',(-105.5,27.9375,-43.6995308303615));
#6837=CARTESIAN_POINT('Ctrl Pts',(-74.5997654151808,27.875,-74.5997654151808));
#6838=CARTESIAN_POINT('Ctrl Pts',(-43.6995308303615,27.8125,-105.5));
#6839=CARTESIAN_POINT('Ctrl Pts',(-6.46001186550229E-15,27.75,-105.5));
#6840=CARTESIAN_POINT('Ctrl Pts',(43.6995308303615,27.6875,-105.5));
#6841=CARTESIAN_POINT('Ctrl Pts',(74.5997654151808,27.625,-74.5997654151808));
#6842=CARTESIAN_POINT('Ctrl Pts',(105.5,27.5625,-43.6995308303616));
#6843=CARTESIAN_POINT('Ctrl Pts',(105.5,27.5,-1.29200237310046E-14));
#6844=CARTESIAN_POINT('Ctrl Pts',(105.5,27.4375,43.6995308303615));
#6845=CARTESIAN_POINT('Ctrl Pts',(74.5997654151808,27.375,74.5997654151808));
#6846=CARTESIAN_POINT('Ctrl Pts',(43.6995308303616,27.3125,105.5));
#6847=CARTESIAN_POINT('Ctrl Pts',(1.93800355965069E-14,27.25,105.5));
#6848=CARTESIAN_POINT('Ctrl Pts',(1.93800355965069E-14,28.3750000027312,
105.5));
#6849=CARTESIAN_POINT('Ctrl Pts',(-43.6995308303616,28.3125000027312,105.5));
#6850=CARTESIAN_POINT('Ctrl Pts',(-74.5997654151808,28.2500000027312,74.5997654151808));
#6851=CARTESIAN_POINT('Ctrl Pts',(-105.5,28.1875000027312,43.6995308303616));
#6852=CARTESIAN_POINT('Ctrl Pts',(-105.5,28.1250000027312,0.));
#6853=CARTESIAN_POINT('Ctrl Pts',(-105.5,28.0625000027312,-43.6995308303615));
#6854=CARTESIAN_POINT('Ctrl Pts',(-74.5997654151808,28.0000000027312,-74.5997654151808));
#6855=CARTESIAN_POINT('Ctrl Pts',(-43.6995308303615,27.9375000027312,-105.5));
#6856=CARTESIAN_POINT('Ctrl Pts',(-6.46001186550229E-15,27.8750000027312,
-105.5));
#6857=CARTESIAN_POINT('Ctrl Pts',(43.6995308303615,27.8125000027312,-105.5));
#6858=CARTESIAN_POINT('Ctrl Pts',(74.5997654151808,27.7500000027312,-74.5997654151808));
#6859=CARTESIAN_POINT('Ctrl Pts',(105.5,27.6875000027312,-43.6995308303616));
#6860=CARTESIAN_POINT('Ctrl Pts',(105.5,27.6250000027312,-1.29200237310046E-14));
#6861=CARTESIAN_POINT('Ctrl Pts',(105.5,27.5625000027312,43.6995308303615));
#6862=CARTESIAN_POINT('Ctrl Pts',(74.5997654151808,27.5000000027312,74.5997654151808));
#6863=CARTESIAN_POINT('Ctrl Pts',(43.6995308303616,27.4375000027312,105.5));
#6864=CARTESIAN_POINT('Ctrl Pts',(1.93800355965069E-14,27.3750000027312,
105.5));
#6865=CARTESIAN_POINT('Origin',(0.,105.,0.));
#6866=CARTESIAN_POINT('',(3.23000593275114E-15,29.3750000027312,105.5));
#6867=CARTESIAN_POINT('',(3.23000593275114E-15,29.25,105.5));
#6868=CARTESIAN_POINT('',(-1.29200237310046E-14,105.,105.5));
#6869=CARTESIAN_POINT('Ctrl Pts',(1.93800355965069E-14,29.25,105.5));
#6870=CARTESIAN_POINT('Ctrl Pts',(-43.6995308303616,29.1875,105.5));
#6871=CARTESIAN_POINT('Ctrl Pts',(-74.5997654151808,29.125,74.5997654151808));
#6872=CARTESIAN_POINT('Ctrl Pts',(-105.5,29.0625,43.6995308303616));
#6873=CARTESIAN_POINT('Ctrl Pts',(-105.5,29.,0.));
#6874=CARTESIAN_POINT('Ctrl Pts',(-105.5,28.9375,-43.6995308303615));
#6875=CARTESIAN_POINT('Ctrl Pts',(-74.5997654151808,28.875,-74.5997654151808));
#6876=CARTESIAN_POINT('Ctrl Pts',(-43.6995308303615,28.8125,-105.5));
#6877=CARTESIAN_POINT('Ctrl Pts',(-6.46001186550229E-15,28.75,-105.5));
#6878=CARTESIAN_POINT('Ctrl Pts',(43.6995308303615,28.6875,-105.5));
#6879=CARTESIAN_POINT('Ctrl Pts',(74.5997654151808,28.625,-74.5997654151808));
#6880=CARTESIAN_POINT('Ctrl Pts',(105.5,28.5625,-43.6995308303616));
#6881=CARTESIAN_POINT('Ctrl Pts',(105.5,28.5,-1.29200237310046E-14));
#6882=CARTESIAN_POINT('Ctrl Pts',(105.5,28.4375,43.6995308303615));
#6883=CARTESIAN_POINT('Ctrl Pts',(74.5997654151808,28.375,74.5997654151808));
#6884=CARTESIAN_POINT('Ctrl Pts',(43.6995308303616,28.3125,105.5));
#6885=CARTESIAN_POINT('Ctrl Pts',(1.93800355965069E-14,28.25,105.5));
#6886=CARTESIAN_POINT('Ctrl Pts',(1.93800355965069E-14,29.3750000027312,
105.5));
#6887=CARTESIAN_POINT('Ctrl Pts',(-43.6995308303616,29.3125000027312,105.5));
#6888=CARTESIAN_POINT('Ctrl Pts',(-74.5997654151808,29.2500000027312,74.5997654151808));
#6889=CARTESIAN_POINT('Ctrl Pts',(-105.5,29.1875000027312,43.6995308303616));
#6890=CARTESIAN_POINT('Ctrl Pts',(-105.5,29.1250000027312,0.));
#6891=CARTESIAN_POINT('Ctrl Pts',(-105.5,29.0625000027312,-43.6995308303615));
#6892=CARTESIAN_POINT('Ctrl Pts',(-74.5997654151808,29.0000000027312,-74.5997654151808));
#6893=CARTESIAN_POINT('Ctrl Pts',(-43.6995308303615,28.9375000027312,-105.5));
#6894=CARTESIAN_POINT('Ctrl Pts',(-6.46001186550229E-15,28.8750000027312,
-105.5));
#6895=CARTESIAN_POINT('Ctrl Pts',(43.6995308303615,28.8125000027312,-105.5));
#6896=CARTESIAN_POINT('Ctrl Pts',(74.5997654151808,28.7500000027312,-74.5997654151808));
#6897=CARTESIAN_POINT('Ctrl Pts',(105.5,28.6875000027312,-43.6995308303616));
#6898=CARTESIAN_POINT('Ctrl Pts',(105.5,28.6250000027312,-1.29200237310046E-14));
#6899=CARTESIAN_POINT('Ctrl Pts',(105.5,28.5625000027312,43.6995308303615));
#6900=CARTESIAN_POINT('Ctrl Pts',(74.5997654151808,28.5000000027312,74.5997654151808));
#6901=CARTESIAN_POINT('Ctrl Pts',(43.6995308303616,28.4375000027312,105.5));
#6902=CARTESIAN_POINT('Ctrl Pts',(1.93800355965069E-14,28.3750000027312,
105.5));
#6903=CARTESIAN_POINT('Origin',(0.,105.,0.));
#6904=CARTESIAN_POINT('',(3.23000593275114E-15,30.3750000027312,105.5));
#6905=CARTESIAN_POINT('',(3.23000593275114E-15,30.25,105.5));
#6906=CARTESIAN_POINT('',(-1.29200237310046E-14,105.,105.5));
#6907=CARTESIAN_POINT('Ctrl Pts',(1.93800355965069E-14,30.25,105.5));
#6908=CARTESIAN_POINT('Ctrl Pts',(-43.6995308303616,30.1875,105.5));
#6909=CARTESIAN_POINT('Ctrl Pts',(-74.5997654151808,30.125,74.5997654151808));
#6910=CARTESIAN_POINT('Ctrl Pts',(-105.5,30.0625,43.6995308303616));
#6911=CARTESIAN_POINT('Ctrl Pts',(-105.5,30.,0.));
#6912=CARTESIAN_POINT('Ctrl Pts',(-105.5,29.9375,-43.6995308303615));
#6913=CARTESIAN_POINT('Ctrl Pts',(-74.5997654151808,29.875,-74.5997654151808));
#6914=CARTESIAN_POINT('Ctrl Pts',(-43.6995308303615,29.8125,-105.5));
#6915=CARTESIAN_POINT('Ctrl Pts',(-6.46001186550229E-15,29.75,-105.5));
#6916=CARTESIAN_POINT('Ctrl Pts',(43.6995308303615,29.6875,-105.5));
#6917=CARTESIAN_POINT('Ctrl Pts',(74.5997654151808,29.625,-74.5997654151808));
#6918=CARTESIAN_POINT('Ctrl Pts',(105.5,29.5625,-43.6995308303616));
#6919=CARTESIAN_POINT('Ctrl Pts',(105.5,29.5,-1.29200237310046E-14));
#6920=CARTESIAN_POINT('Ctrl Pts',(105.5,29.4375,43.6995308303615));
#6921=CARTESIAN_POINT('Ctrl Pts',(74.5997654151808,29.375,74.5997654151808));
#6922=CARTESIAN_POINT('Ctrl Pts',(43.6995308303616,29.3125,105.5));
#6923=CARTESIAN_POINT('Ctrl Pts',(1.93800355965069E-14,29.25,105.5));
#6924=CARTESIAN_POINT('Ctrl Pts',(1.93800355965069E-14,30.3750000027312,
105.5));
#6925=CARTESIAN_POINT('Ctrl Pts',(-43.6995308303616,30.3125000027312,105.5));
#6926=CARTESIAN_POINT('Ctrl Pts',(-74.5997654151808,30.2500000027312,74.5997654151808));
#6927=CARTESIAN_POINT('Ctrl Pts',(-105.5,30.1875000027312,43.6995308303616));
#6928=CARTESIAN_POINT('Ctrl Pts',(-105.5,30.1250000027312,0.));
#6929=CARTESIAN_POINT('Ctrl Pts',(-105.5,30.0625000027312,-43.6995308303615));
#6930=CARTESIAN_POINT('Ctrl Pts',(-74.5997654151808,30.0000000027312,-74.5997654151808));
#6931=CARTESIAN_POINT('Ctrl Pts',(-43.6995308303615,29.9375000027312,-105.5));
#6932=CARTESIAN_POINT('Ctrl Pts',(-6.46001186550229E-15,29.8750000027312,
-105.5));
#6933=CARTESIAN_POINT('Ctrl Pts',(43.6995308303615,29.8125000027312,-105.5));
#6934=CARTESIAN_POINT('Ctrl Pts',(74.5997654151808,29.7500000027312,-74.5997654151808));
#6935=CARTESIAN_POINT('Ctrl Pts',(105.5,29.6875000027312,-43.6995308303616));
#6936=CARTESIAN_POINT('Ctrl Pts',(105.5,29.6250000027312,-1.29200237310046E-14));
#6937=CARTESIAN_POINT('Ctrl Pts',(105.5,29.5625000027312,43.6995308303615));
#6938=CARTESIAN_POINT('Ctrl Pts',(74.5997654151808,29.5000000027312,74.5997654151808));
#6939=CARTESIAN_POINT('Ctrl Pts',(43.6995308303616,29.4375000027312,105.5));
#6940=CARTESIAN_POINT('Ctrl Pts',(1.93800355965069E-14,29.3750000027312,
105.5));
#6941=CARTESIAN_POINT('Origin',(0.,105.,0.));
#6942=CARTESIAN_POINT('',(3.23000593275114E-15,31.3750000027312,105.5));
#6943=CARTESIAN_POINT('',(3.23000593275114E-15,31.25,105.5));
#6944=CARTESIAN_POINT('',(-1.29200237310046E-14,105.,105.5));
#6945=CARTESIAN_POINT('Ctrl Pts',(1.93800355965069E-14,31.25,105.5));
#6946=CARTESIAN_POINT('Ctrl Pts',(-43.6995308303616,31.1875,105.5));
#6947=CARTESIAN_POINT('Ctrl Pts',(-74.5997654151808,31.125,74.5997654151808));
#6948=CARTESIAN_POINT('Ctrl Pts',(-105.5,31.0625,43.6995308303616));
#6949=CARTESIAN_POINT('Ctrl Pts',(-105.5,31.,0.));
#6950=CARTESIAN_POINT('Ctrl Pts',(-105.5,30.9375,-43.6995308303615));
#6951=CARTESIAN_POINT('Ctrl Pts',(-74.5997654151808,30.875,-74.5997654151808));
#6952=CARTESIAN_POINT('Ctrl Pts',(-43.6995308303615,30.8125,-105.5));
#6953=CARTESIAN_POINT('Ctrl Pts',(-6.46001186550229E-15,30.75,-105.5));
#6954=CARTESIAN_POINT('Ctrl Pts',(43.6995308303615,30.6875,-105.5));
#6955=CARTESIAN_POINT('Ctrl Pts',(74.5997654151808,30.625,-74.5997654151808));
#6956=CARTESIAN_POINT('Ctrl Pts',(105.5,30.5625,-43.6995308303616));
#6957=CARTESIAN_POINT('Ctrl Pts',(105.5,30.5,-1.29200237310046E-14));
#6958=CARTESIAN_POINT('Ctrl Pts',(105.5,30.4375,43.6995308303615));
#6959=CARTESIAN_POINT('Ctrl Pts',(74.5997654151808,30.375,74.5997654151808));
#6960=CARTESIAN_POINT('Ctrl Pts',(43.6995308303616,30.3125,105.5));
#6961=CARTESIAN_POINT('Ctrl Pts',(1.93800355965069E-14,30.25,105.5));
#6962=CARTESIAN_POINT('Ctrl Pts',(1.93800355965069E-14,31.3750000027312,
105.5));
#6963=CARTESIAN_POINT('Ctrl Pts',(-43.6995308303616,31.3125000027312,105.5));
#6964=CARTESIAN_POINT('Ctrl Pts',(-74.5997654151808,31.2500000027312,74.5997654151808));
#6965=CARTESIAN_POINT('Ctrl Pts',(-105.5,31.1875000027312,43.6995308303616));
#6966=CARTESIAN_POINT('Ctrl Pts',(-105.5,31.1250000027312,0.));
#6967=CARTESIAN_POINT('Ctrl Pts',(-105.5,31.0625000027312,-43.6995308303615));
#6968=CARTESIAN_POINT('Ctrl Pts',(-74.5997654151808,31.0000000027312,-74.5997654151808));
#6969=CARTESIAN_POINT('Ctrl Pts',(-43.6995308303615,30.9375000027312,-105.5));
#6970=CARTESIAN_POINT('Ctrl Pts',(-6.46001186550229E-15,30.8750000027312,
-105.5));
#6971=CARTESIAN_POINT('Ctrl Pts',(43.6995308303615,30.8125000027312,-105.5));
#6972=CARTESIAN_POINT('Ctrl Pts',(74.5997654151808,30.7500000027312,-74.5997654151808));
#6973=CARTESIAN_POINT('Ctrl Pts',(105.5,30.6875000027312,-43.6995308303616));
#6974=CARTESIAN_POINT('Ctrl Pts',(105.5,30.6250000027312,-1.29200237310046E-14));
#6975=CARTESIAN_POINT('Ctrl Pts',(105.5,30.5625000027312,43.6995308303615));
#6976=CARTESIAN_POINT('Ctrl Pts',(74.5997654151808,30.5000000027312,74.5997654151808));
#6977=CARTESIAN_POINT('Ctrl Pts',(43.6995308303616,30.4375000027312,105.5));
#6978=CARTESIAN_POINT('Ctrl Pts',(1.93800355965069E-14,30.3750000027312,
105.5));
#6979=CARTESIAN_POINT('Origin',(0.,105.,0.));
#6980=CARTESIAN_POINT('',(3.23000593275114E-15,32.3750000027312,105.5));
#6981=CARTESIAN_POINT('',(3.23000593275114E-15,32.25,105.5));
#6982=CARTESIAN_POINT('',(-1.29200237310046E-14,105.,105.5));
#6983=CARTESIAN_POINT('Ctrl Pts',(1.93800355965069E-14,32.25,105.5));
#6984=CARTESIAN_POINT('Ctrl Pts',(-43.6995308303616,32.1875,105.5));
#6985=CARTESIAN_POINT('Ctrl Pts',(-74.5997654151808,32.125,74.5997654151808));
#6986=CARTESIAN_POINT('Ctrl Pts',(-105.5,32.0625,43.6995308303616));
#6987=CARTESIAN_POINT('Ctrl Pts',(-105.5,32.,0.));
#6988=CARTESIAN_POINT('Ctrl Pts',(-105.5,31.9375,-43.6995308303615));
#6989=CARTESIAN_POINT('Ctrl Pts',(-74.5997654151808,31.875,-74.5997654151808));
#6990=CARTESIAN_POINT('Ctrl Pts',(-43.6995308303615,31.8125,-105.5));
#6991=CARTESIAN_POINT('Ctrl Pts',(-6.46001186550229E-15,31.75,-105.5));
#6992=CARTESIAN_POINT('Ctrl Pts',(43.6995308303615,31.6875,-105.5));
#6993=CARTESIAN_POINT('Ctrl Pts',(74.5997654151808,31.625,-74.5997654151808));
#6994=CARTESIAN_POINT('Ctrl Pts',(105.5,31.5625,-43.6995308303616));
#6995=CARTESIAN_POINT('Ctrl Pts',(105.5,31.5,-1.29200237310046E-14));
#6996=CARTESIAN_POINT('Ctrl Pts',(105.5,31.4375,43.6995308303615));
#6997=CARTESIAN_POINT('Ctrl Pts',(74.5997654151808,31.375,74.5997654151808));
#6998=CARTESIAN_POINT('Ctrl Pts',(43.6995308303616,31.3125,105.5));
#6999=CARTESIAN_POINT('Ctrl Pts',(1.93800355965069E-14,31.25,105.5));
#7000=CARTESIAN_POINT('Ctrl Pts',(1.93800355965069E-14,32.3750000027312,
105.5));
#7001=CARTESIAN_POINT('Ctrl Pts',(-43.6995308303616,32.3125000027312,105.5));
#7002=CARTESIAN_POINT('Ctrl Pts',(-74.5997654151808,32.2500000027312,74.5997654151808));
#7003=CARTESIAN_POINT('Ctrl Pts',(-105.5,32.1875000027312,43.6995308303616));
#7004=CARTESIAN_POINT('Ctrl Pts',(-105.5,32.1250000027312,0.));
#7005=CARTESIAN_POINT('Ctrl Pts',(-105.5,32.0625000027312,-43.6995308303615));
#7006=CARTESIAN_POINT('Ctrl Pts',(-74.5997654151808,32.0000000027312,-74.5997654151808));
#7007=CARTESIAN_POINT('Ctrl Pts',(-43.6995308303615,31.9375000027312,-105.5));
#7008=CARTESIAN_POINT('Ctrl Pts',(-6.46001186550229E-15,31.8750000027312,
-105.5));
#7009=CARTESIAN_POINT('Ctrl Pts',(43.6995308303615,31.8125000027312,-105.5));
#7010=CARTESIAN_POINT('Ctrl Pts',(74.5997654151808,31.7500000027312,-74.5997654151808));
#7011=CARTESIAN_POINT('Ctrl Pts',(105.5,31.6875000027312,-43.6995308303616));
#7012=CARTESIAN_POINT('Ctrl Pts',(105.5,31.6250000027312,-1.29200237310046E-14));
#7013=CARTESIAN_POINT('Ctrl Pts',(105.5,31.5625000027312,43.6995308303615));
#7014=CARTESIAN_POINT('Ctrl Pts',(74.5997654151808,31.5000000027312,74.5997654151808));
#7015=CARTESIAN_POINT('Ctrl Pts',(43.6995308303616,31.4375000027312,105.5));
#7016=CARTESIAN_POINT('Ctrl Pts',(1.93800355965069E-14,31.3750000027312,
105.5));
#7017=CARTESIAN_POINT('Origin',(0.,105.,0.));
#7018=CARTESIAN_POINT('',(3.23000593275114E-15,33.3750000027312,105.5));
#7019=CARTESIAN_POINT('',(3.23000593275114E-15,33.25,105.5));
#7020=CARTESIAN_POINT('',(-1.29200237310046E-14,105.,105.5));
#7021=CARTESIAN_POINT('Ctrl Pts',(1.93800355965069E-14,33.25,105.5));
#7022=CARTESIAN_POINT('Ctrl Pts',(-43.6995308303616,33.1875,105.5));
#7023=CARTESIAN_POINT('Ctrl Pts',(-74.5997654151808,33.125,74.5997654151808));
#7024=CARTESIAN_POINT('Ctrl Pts',(-105.5,33.0625,43.6995308303616));
#7025=CARTESIAN_POINT('Ctrl Pts',(-105.5,33.,0.));
#7026=CARTESIAN_POINT('Ctrl Pts',(-105.5,32.9375,-43.6995308303615));
#7027=CARTESIAN_POINT('Ctrl Pts',(-74.5997654151808,32.875,-74.5997654151808));
#7028=CARTESIAN_POINT('Ctrl Pts',(-43.6995308303615,32.8125,-105.5));
#7029=CARTESIAN_POINT('Ctrl Pts',(-6.46001186550229E-15,32.75,-105.5));
#7030=CARTESIAN_POINT('Ctrl Pts',(43.6995308303615,32.6875,-105.5));
#7031=CARTESIAN_POINT('Ctrl Pts',(74.5997654151808,32.625,-74.5997654151808));
#7032=CARTESIAN_POINT('Ctrl Pts',(105.5,32.5625,-43.6995308303616));
#7033=CARTESIAN_POINT('Ctrl Pts',(105.5,32.5,-1.29200237310046E-14));
#7034=CARTESIAN_POINT('Ctrl Pts',(105.5,32.4375,43.6995308303615));
#7035=CARTESIAN_POINT('Ctrl Pts',(74.5997654151808,32.375,74.5997654151808));
#7036=CARTESIAN_POINT('Ctrl Pts',(43.6995308303616,32.3125,105.5));
#7037=CARTESIAN_POINT('Ctrl Pts',(1.93800355965069E-14,32.25,105.5));
#7038=CARTESIAN_POINT('Ctrl Pts',(1.93800355965069E-14,33.3750000027312,
105.5));
#7039=CARTESIAN_POINT('Ctrl Pts',(-43.6995308303616,33.3125000027312,105.5));
#7040=CARTESIAN_POINT('Ctrl Pts',(-74.5997654151808,33.2500000027312,74.5997654151808));
#7041=CARTESIAN_POINT('Ctrl Pts',(-105.5,33.1875000027312,43.6995308303616));
#7042=CARTESIAN_POINT('Ctrl Pts',(-105.5,33.1250000027312,0.));
#7043=CARTESIAN_POINT('Ctrl Pts',(-105.5,33.0625000027312,-43.6995308303615));
#7044=CARTESIAN_POINT('Ctrl Pts',(-74.5997654151808,33.0000000027312,-74.5997654151808));
#7045=CARTESIAN_POINT('Ctrl Pts',(-43.6995308303615,32.9375000027312,-105.5));
#7046=CARTESIAN_POINT('Ctrl Pts',(-6.46001186550229E-15,32.8750000027312,
-105.5));
#7047=CARTESIAN_POINT('Ctrl Pts',(43.6995308303615,32.8125000027312,-105.5));
#7048=CARTESIAN_POINT('Ctrl Pts',(74.5997654151808,32.7500000027312,-74.5997654151808));
#7049=CARTESIAN_POINT('Ctrl Pts',(105.5,32.6875000027312,-43.6995308303616));
#7050=CARTESIAN_POINT('Ctrl Pts',(105.5,32.6250000027312,-1.29200237310046E-14));
#7051=CARTESIAN_POINT('Ctrl Pts',(105.5,32.5625000027312,43.6995308303615));
#7052=CARTESIAN_POINT('Ctrl Pts',(74.5997654151808,32.5000000027312,74.5997654151808));
#7053=CARTESIAN_POINT('Ctrl Pts',(43.6995308303616,32.4375000027312,105.5));
#7054=CARTESIAN_POINT('Ctrl Pts',(1.93800355965069E-14,32.3750000027312,
105.5));
#7055=CARTESIAN_POINT('Origin',(0.,105.,0.));
#7056=CARTESIAN_POINT('',(3.23000593275114E-15,34.3750000027312,105.5));
#7057=CARTESIAN_POINT('',(3.23000593275114E-15,34.25,105.5));
#7058=CARTESIAN_POINT('',(-1.29200237310046E-14,105.,105.5));
#7059=CARTESIAN_POINT('Ctrl Pts',(1.93800355965069E-14,34.25,105.5));
#7060=CARTESIAN_POINT('Ctrl Pts',(-43.6995308303616,34.1875,105.5));
#7061=CARTESIAN_POINT('Ctrl Pts',(-74.5997654151808,34.125,74.5997654151808));
#7062=CARTESIAN_POINT('Ctrl Pts',(-105.5,34.0625,43.6995308303616));
#7063=CARTESIAN_POINT('Ctrl Pts',(-105.5,34.,0.));
#7064=CARTESIAN_POINT('Ctrl Pts',(-105.5,33.9375,-43.6995308303615));
#7065=CARTESIAN_POINT('Ctrl Pts',(-74.5997654151808,33.875,-74.5997654151808));
#7066=CARTESIAN_POINT('Ctrl Pts',(-43.6995308303615,33.8125,-105.5));
#7067=CARTESIAN_POINT('Ctrl Pts',(-6.46001186550229E-15,33.75,-105.5));
#7068=CARTESIAN_POINT('Ctrl Pts',(43.6995308303615,33.6875,-105.5));
#7069=CARTESIAN_POINT('Ctrl Pts',(74.5997654151808,33.625,-74.5997654151808));
#7070=CARTESIAN_POINT('Ctrl Pts',(105.5,33.5625,-43.6995308303616));
#7071=CARTESIAN_POINT('Ctrl Pts',(105.5,33.5,-1.29200237310046E-14));
#7072=CARTESIAN_POINT('Ctrl Pts',(105.5,33.4375,43.6995308303615));
#7073=CARTESIAN_POINT('Ctrl Pts',(74.5997654151808,33.375,74.5997654151808));
#7074=CARTESIAN_POINT('Ctrl Pts',(43.6995308303616,33.3125,105.5));
#7075=CARTESIAN_POINT('Ctrl Pts',(1.93800355965069E-14,33.25,105.5));
#7076=CARTESIAN_POINT('Ctrl Pts',(1.93800355965069E-14,34.3750000027312,
105.5));
#7077=CARTESIAN_POINT('Ctrl Pts',(-43.6995308303616,34.3125000027312,105.5));
#7078=CARTESIAN_POINT('Ctrl Pts',(-74.5997654151808,34.2500000027312,74.5997654151808));
#7079=CARTESIAN_POINT('Ctrl Pts',(-105.5,34.1875000027312,43.6995308303616));
#7080=CARTESIAN_POINT('Ctrl Pts',(-105.5,34.1250000027312,0.));
#7081=CARTESIAN_POINT('Ctrl Pts',(-105.5,34.0625000027312,-43.6995308303615));
#7082=CARTESIAN_POINT('Ctrl Pts',(-74.5997654151808,34.0000000027312,-74.5997654151808));
#7083=CARTESIAN_POINT('Ctrl Pts',(-43.6995308303615,33.9375000027312,-105.5));
#7084=CARTESIAN_POINT('Ctrl Pts',(-6.46001186550229E-15,33.8750000027312,
-105.5));
#7085=CARTESIAN_POINT('Ctrl Pts',(43.6995308303615,33.8125000027312,-105.5));
#7086=CARTESIAN_POINT('Ctrl Pts',(74.5997654151808,33.7500000027312,-74.5997654151808));
#7087=CARTESIAN_POINT('Ctrl Pts',(105.5,33.6875000027312,-43.6995308303616));
#7088=CARTESIAN_POINT('Ctrl Pts',(105.5,33.6250000027312,-1.29200237310046E-14));
#7089=CARTESIAN_POINT('Ctrl Pts',(105.5,33.5625000027312,43.6995308303615));
#7090=CARTESIAN_POINT('Ctrl Pts',(74.5997654151808,33.5000000027312,74.5997654151808));
#7091=CARTESIAN_POINT('Ctrl Pts',(43.6995308303616,33.4375000027312,105.5));
#7092=CARTESIAN_POINT('Ctrl Pts',(1.93800355965069E-14,33.3750000027312,
105.5));
#7093=CARTESIAN_POINT('Origin',(0.,105.,0.));
#7094=CARTESIAN_POINT('',(3.23000593275114E-15,35.3750000027312,105.5));
#7095=CARTESIAN_POINT('',(3.23000593275114E-15,35.25,105.5));
#7096=CARTESIAN_POINT('',(-1.29200237310046E-14,105.,105.5));
#7097=CARTESIAN_POINT('Ctrl Pts',(1.93800355965069E-14,35.25,105.5));
#7098=CARTESIAN_POINT('Ctrl Pts',(-43.6995308303616,35.1875,105.5));
#7099=CARTESIAN_POINT('Ctrl Pts',(-74.5997654151808,35.125,74.5997654151808));
#7100=CARTESIAN_POINT('Ctrl Pts',(-105.5,35.0625,43.6995308303616));
#7101=CARTESIAN_POINT('Ctrl Pts',(-105.5,35.,0.));
#7102=CARTESIAN_POINT('Ctrl Pts',(-105.5,34.9375,-43.6995308303615));
#7103=CARTESIAN_POINT('Ctrl Pts',(-74.5997654151808,34.875,-74.5997654151808));
#7104=CARTESIAN_POINT('Ctrl Pts',(-43.6995308303615,34.8125,-105.5));
#7105=CARTESIAN_POINT('Ctrl Pts',(-6.46001186550229E-15,34.75,-105.5));
#7106=CARTESIAN_POINT('Ctrl Pts',(43.6995308303615,34.6875,-105.5));
#7107=CARTESIAN_POINT('Ctrl Pts',(74.5997654151808,34.625,-74.5997654151808));
#7108=CARTESIAN_POINT('Ctrl Pts',(105.5,34.5625,-43.6995308303616));
#7109=CARTESIAN_POINT('Ctrl Pts',(105.5,34.5,-1.29200237310046E-14));
#7110=CARTESIAN_POINT('Ctrl Pts',(105.5,34.4375,43.6995308303615));
#7111=CARTESIAN_POINT('Ctrl Pts',(74.5997654151808,34.375,74.5997654151808));
#7112=CARTESIAN_POINT('Ctrl Pts',(43.6995308303616,34.3125,105.5));
#7113=CARTESIAN_POINT('Ctrl Pts',(1.93800355965069E-14,34.25,105.5));
#7114=CARTESIAN_POINT('Ctrl Pts',(1.93800355965069E-14,35.3750000027312,
105.5));
#7115=CARTESIAN_POINT('Ctrl Pts',(-43.6995308303616,35.3125000027312,105.5));
#7116=CARTESIAN_POINT('Ctrl Pts',(-74.5997654151808,35.2500000027312,74.5997654151808));
#7117=CARTESIAN_POINT('Ctrl Pts',(-105.5,35.1875000027312,43.6995308303616));
#7118=CARTESIAN_POINT('Ctrl Pts',(-105.5,35.1250000027312,0.));
#7119=CARTESIAN_POINT('Ctrl Pts',(-105.5,35.0625000027312,-43.6995308303615));
#7120=CARTESIAN_POINT('Ctrl Pts',(-74.5997654151808,35.0000000027312,-74.5997654151808));
#7121=CARTESIAN_POINT('Ctrl Pts',(-43.6995308303615,34.9375000027312,-105.5));
#7122=CARTESIAN_POINT('Ctrl Pts',(-6.46001186550229E-15,34.8750000027312,
-105.5));
#7123=CARTESIAN_POINT('Ctrl Pts',(43.6995308303615,34.8125000027312,-105.5));
#7124=CARTESIAN_POINT('Ctrl Pts',(74.5997654151808,34.7500000027312,-74.5997654151808));
#7125=CARTESIAN_POINT('Ctrl Pts',(105.5,34.6875000027312,-43.6995308303616));
#7126=CARTESIAN_POINT('Ctrl Pts',(105.5,34.6250000027312,-1.29200237310046E-14));
#7127=CARTESIAN_POINT('Ctrl Pts',(105.5,34.5625000027312,43.6995308303615));
#7128=CARTESIAN_POINT('Ctrl Pts',(74.5997654151808,34.5000000027312,74.5997654151808));
#7129=CARTESIAN_POINT('Ctrl Pts',(43.6995308303616,34.4375000027312,105.5));
#7130=CARTESIAN_POINT('Ctrl Pts',(1.93800355965069E-14,34.3750000027312,
105.5));
#7131=CARTESIAN_POINT('Origin',(0.,105.,0.));
#7132=CARTESIAN_POINT('',(3.23000593275114E-15,36.3750000027312,105.5));
#7133=CARTESIAN_POINT('',(3.23000593275114E-15,36.25,105.5));
#7134=CARTESIAN_POINT('',(-1.29200237310046E-14,105.,105.5));
#7135=CARTESIAN_POINT('Ctrl Pts',(1.93800355965069E-14,36.25,105.5));
#7136=CARTESIAN_POINT('Ctrl Pts',(-43.6995308303616,36.1875,105.5));
#7137=CARTESIAN_POINT('Ctrl Pts',(-74.5997654151808,36.125,74.5997654151808));
#7138=CARTESIAN_POINT('Ctrl Pts',(-105.5,36.0625,43.6995308303616));
#7139=CARTESIAN_POINT('Ctrl Pts',(-105.5,36.,0.));
#7140=CARTESIAN_POINT('Ctrl Pts',(-105.5,35.9375,-43.6995308303615));
#7141=CARTESIAN_POINT('Ctrl Pts',(-74.5997654151808,35.875,-74.5997654151808));
#7142=CARTESIAN_POINT('Ctrl Pts',(-43.6995308303615,35.8125,-105.5));
#7143=CARTESIAN_POINT('Ctrl Pts',(-6.46001186550229E-15,35.75,-105.5));
#7144=CARTESIAN_POINT('Ctrl Pts',(43.6995308303615,35.6875,-105.5));
#7145=CARTESIAN_POINT('Ctrl Pts',(74.5997654151808,35.625,-74.5997654151808));
#7146=CARTESIAN_POINT('Ctrl Pts',(105.5,35.5625,-43.6995308303616));
#7147=CARTESIAN_POINT('Ctrl Pts',(105.5,35.5,-1.29200237310046E-14));
#7148=CARTESIAN_POINT('Ctrl Pts',(105.5,35.4375,43.6995308303615));
#7149=CARTESIAN_POINT('Ctrl Pts',(74.5997654151808,35.375,74.5997654151808));
#7150=CARTESIAN_POINT('Ctrl Pts',(43.6995308303616,35.3125,105.5));
#7151=CARTESIAN_POINT('Ctrl Pts',(1.93800355965069E-14,35.25,105.5));
#7152=CARTESIAN_POINT('Ctrl Pts',(1.93800355965069E-14,36.3750000027312,
105.5));
#7153=CARTESIAN_POINT('Ctrl Pts',(-43.6995308303616,36.3125000027312,105.5));
#7154=CARTESIAN_POINT('Ctrl Pts',(-74.5997654151808,36.2500000027312,74.5997654151808));
#7155=CARTESIAN_POINT('Ctrl Pts',(-105.5,36.1875000027312,43.6995308303616));
#7156=CARTESIAN_POINT('Ctrl Pts',(-105.5,36.1250000027312,0.));
#7157=CARTESIAN_POINT('Ctrl Pts',(-105.5,36.0625000027312,-43.6995308303615));
#7158=CARTESIAN_POINT('Ctrl Pts',(-74.5997654151808,36.0000000027312,-74.5997654151808));
#7159=CARTESIAN_POINT('Ctrl Pts',(-43.6995308303615,35.9375000027312,-105.5));
#7160=CARTESIAN_POINT('Ctrl Pts',(-6.46001186550229E-15,35.8750000027312,
-105.5));
#7161=CARTESIAN_POINT('Ctrl Pts',(43.6995308303615,35.8125000027312,-105.5));
#7162=CARTESIAN_POINT('Ctrl Pts',(74.5997654151808,35.7500000027312,-74.5997654151808));
#7163=CARTESIAN_POINT('Ctrl Pts',(105.5,35.6875000027312,-43.6995308303616));
#7164=CARTESIAN_POINT('Ctrl Pts',(105.5,35.6250000027312,-1.29200237310046E-14));
#7165=CARTESIAN_POINT('Ctrl Pts',(105.5,35.5625000027312,43.6995308303615));
#7166=CARTESIAN_POINT('Ctrl Pts',(74.5997654151808,35.5000000027312,74.5997654151808));
#7167=CARTESIAN_POINT('Ctrl Pts',(43.6995308303616,35.4375000027312,105.5));
#7168=CARTESIAN_POINT('Ctrl Pts',(1.93800355965069E-14,35.3750000027312,
105.5));
#7169=CARTESIAN_POINT('Origin',(0.,105.,0.));
#7170=CARTESIAN_POINT('',(3.23000593275114E-15,37.3750000027312,105.5));
#7171=CARTESIAN_POINT('',(3.23000593275114E-15,37.25,105.5));
#7172=CARTESIAN_POINT('',(-1.29200237310046E-14,105.,105.5));
#7173=CARTESIAN_POINT('Ctrl Pts',(1.93800355965069E-14,37.25,105.5));
#7174=CARTESIAN_POINT('Ctrl Pts',(-43.6995308303616,37.1875,105.5));
#7175=CARTESIAN_POINT('Ctrl Pts',(-74.5997654151808,37.125,74.5997654151808));
#7176=CARTESIAN_POINT('Ctrl Pts',(-105.5,37.0625,43.6995308303616));
#7177=CARTESIAN_POINT('Ctrl Pts',(-105.5,37.,0.));
#7178=CARTESIAN_POINT('Ctrl Pts',(-105.5,36.9375,-43.6995308303615));
#7179=CARTESIAN_POINT('Ctrl Pts',(-74.5997654151808,36.875,-74.5997654151808));
#7180=CARTESIAN_POINT('Ctrl Pts',(-43.6995308303615,36.8125,-105.5));
#7181=CARTESIAN_POINT('Ctrl Pts',(-6.46001186550229E-15,36.75,-105.5));
#7182=CARTESIAN_POINT('Ctrl Pts',(43.6995308303615,36.6875,-105.5));
#7183=CARTESIAN_POINT('Ctrl Pts',(74.5997654151808,36.625,-74.5997654151808));
#7184=CARTESIAN_POINT('Ctrl Pts',(105.5,36.5625,-43.6995308303616));
#7185=CARTESIAN_POINT('Ctrl Pts',(105.5,36.5,-1.29200237310046E-14));
#7186=CARTESIAN_POINT('Ctrl Pts',(105.5,36.4375,43.6995308303615));
#7187=CARTESIAN_POINT('Ctrl Pts',(74.5997654151808,36.375,74.5997654151808));
#7188=CARTESIAN_POINT('Ctrl Pts',(43.6995308303616,36.3125,105.5));
#7189=CARTESIAN_POINT('Ctrl Pts',(1.93800355965069E-14,36.25,105.5));
#7190=CARTESIAN_POINT('Ctrl Pts',(1.93800355965069E-14,37.3750000027312,
105.5));
#7191=CARTESIAN_POINT('Ctrl Pts',(-43.6995308303616,37.3125000027312,105.5));
#7192=CARTESIAN_POINT('Ctrl Pts',(-74.5997654151808,37.2500000027312,74.5997654151808));
#7193=CARTESIAN_POINT('Ctrl Pts',(-105.5,37.1875000027312,43.6995308303616));
#7194=CARTESIAN_POINT('Ctrl Pts',(-105.5,37.1250000027312,0.));
#7195=CARTESIAN_POINT('Ctrl Pts',(-105.5,37.0625000027312,-43.6995308303615));
#7196=CARTESIAN_POINT('Ctrl Pts',(-74.5997654151808,37.0000000027312,-74.5997654151808));
#7197=CARTESIAN_POINT('Ctrl Pts',(-43.6995308303615,36.9375000027312,-105.5));
#7198=CARTESIAN_POINT('Ctrl Pts',(-6.46001186550229E-15,36.8750000027312,
-105.5));
#7199=CARTESIAN_POINT('Ctrl Pts',(43.6995308303615,36.8125000027312,-105.5));
#7200=CARTESIAN_POINT('Ctrl Pts',(74.5997654151808,36.7500000027312,-74.5997654151808));
#7201=CARTESIAN_POINT('Ctrl Pts',(105.5,36.6875000027312,-43.6995308303616));
#7202=CARTESIAN_POINT('Ctrl Pts',(105.5,36.6250000027312,-1.29200237310046E-14));
#7203=CARTESIAN_POINT('Ctrl Pts',(105.5,36.5625000027312,43.6995308303615));
#7204=CARTESIAN_POINT('Ctrl Pts',(74.5997654151808,36.5000000027312,74.5997654151808));
#7205=CARTESIAN_POINT('Ctrl Pts',(43.6995308303616,36.4375000027312,105.5));
#7206=CARTESIAN_POINT('Ctrl Pts',(1.93800355965069E-14,36.3750000027312,
105.5));
#7207=CARTESIAN_POINT('Origin',(0.,105.,0.));
#7208=CARTESIAN_POINT('',(3.23000593275114E-15,38.3750000027312,105.5));
#7209=CARTESIAN_POINT('',(3.23000593275114E-15,38.25,105.5));
#7210=CARTESIAN_POINT('',(-1.29200237310046E-14,105.,105.5));
#7211=CARTESIAN_POINT('Ctrl Pts',(1.93800355965069E-14,38.25,105.5));
#7212=CARTESIAN_POINT('Ctrl Pts',(-43.6995308303616,38.1875,105.5));
#7213=CARTESIAN_POINT('Ctrl Pts',(-74.5997654151808,38.125,74.5997654151808));
#7214=CARTESIAN_POINT('Ctrl Pts',(-105.5,38.0625,43.6995308303616));
#7215=CARTESIAN_POINT('Ctrl Pts',(-105.5,38.,0.));
#7216=CARTESIAN_POINT('Ctrl Pts',(-105.5,37.9375,-43.6995308303615));
#7217=CARTESIAN_POINT('Ctrl Pts',(-74.5997654151808,37.875,-74.5997654151808));
#7218=CARTESIAN_POINT('Ctrl Pts',(-43.6995308303615,37.8125,-105.5));
#7219=CARTESIAN_POINT('Ctrl Pts',(-6.46001186550229E-15,37.75,-105.5));
#7220=CARTESIAN_POINT('Ctrl Pts',(43.6995308303615,37.6875,-105.5));
#7221=CARTESIAN_POINT('Ctrl Pts',(74.5997654151808,37.625,-74.5997654151808));
#7222=CARTESIAN_POINT('Ctrl Pts',(105.5,37.5625,-43.6995308303616));
#7223=CARTESIAN_POINT('Ctrl Pts',(105.5,37.5,-1.29200237310046E-14));
#7224=CARTESIAN_POINT('Ctrl Pts',(105.5,37.4375,43.6995308303615));
#7225=CARTESIAN_POINT('Ctrl Pts',(74.5997654151808,37.375,74.5997654151808));
#7226=CARTESIAN_POINT('Ctrl Pts',(43.6995308303616,37.3125,105.5));
#7227=CARTESIAN_POINT('Ctrl Pts',(1.93800355965069E-14,37.25,105.5));
#7228=CARTESIAN_POINT('Ctrl Pts',(1.93800355965069E-14,38.3750000027312,
105.5));
#7229=CARTESIAN_POINT('Ctrl Pts',(-43.6995308303616,38.3125000027312,105.5));
#7230=CARTESIAN_POINT('Ctrl Pts',(-74.5997654151808,38.2500000027312,74.5997654151808));
#7231=CARTESIAN_POINT('Ctrl Pts',(-105.5,38.1875000027312,43.6995308303616));
#7232=CARTESIAN_POINT('Ctrl Pts',(-105.5,38.1250000027312,0.));
#7233=CARTESIAN_POINT('Ctrl Pts',(-105.5,38.0625000027312,-43.6995308303615));
#7234=CARTESIAN_POINT('Ctrl Pts',(-74.5997654151808,38.0000000027312,-74.5997654151808));
#7235=CARTESIAN_POINT('Ctrl Pts',(-43.6995308303615,37.9375000027312,-105.5));
#7236=CARTESIAN_POINT('Ctrl Pts',(-6.46001186550229E-15,37.8750000027312,
-105.5));
#7237=CARTESIAN_POINT('Ctrl Pts',(43.6995308303615,37.8125000027312,-105.5));
#7238=CARTESIAN_POINT('Ctrl Pts',(74.5997654151808,37.7500000027312,-74.5997654151808));
#7239=CARTESIAN_POINT('Ctrl Pts',(105.5,37.6875000027312,-43.6995308303616));
#7240=CARTESIAN_POINT('Ctrl Pts',(105.5,37.6250000027312,-1.29200237310046E-14));
#7241=CARTESIAN_POINT('Ctrl Pts',(105.5,37.5625000027312,43.6995308303615));
#7242=CARTESIAN_POINT('Ctrl Pts',(74.5997654151808,37.5000000027312,74.5997654151808));
#7243=CARTESIAN_POINT('Ctrl Pts',(43.6995308303616,37.4375000027312,105.5));
#7244=CARTESIAN_POINT('Ctrl Pts',(1.93800355965069E-14,37.3750000027312,
105.5));
#7245=CARTESIAN_POINT('Origin',(0.,105.,0.));
#7246=CARTESIAN_POINT('',(3.23000593275114E-15,39.3750000027312,105.5));
#7247=CARTESIAN_POINT('',(3.23000593275114E-15,39.25,105.5));
#7248=CARTESIAN_POINT('',(-1.29200237310046E-14,105.,105.5));
#7249=CARTESIAN_POINT('Ctrl Pts',(1.93800355965069E-14,39.25,105.5));
#7250=CARTESIAN_POINT('Ctrl Pts',(-43.6995308303616,39.1875,105.5));
#7251=CARTESIAN_POINT('Ctrl Pts',(-74.5997654151808,39.125,74.5997654151808));
#7252=CARTESIAN_POINT('Ctrl Pts',(-105.5,39.0625,43.6995308303616));
#7253=CARTESIAN_POINT('Ctrl Pts',(-105.5,39.,0.));
#7254=CARTESIAN_POINT('Ctrl Pts',(-105.5,38.9375,-43.6995308303615));
#7255=CARTESIAN_POINT('Ctrl Pts',(-74.5997654151808,38.875,-74.5997654151808));
#7256=CARTESIAN_POINT('Ctrl Pts',(-43.6995308303615,38.8125,-105.5));
#7257=CARTESIAN_POINT('Ctrl Pts',(-6.46001186550229E-15,38.75,-105.5));
#7258=CARTESIAN_POINT('Ctrl Pts',(43.6995308303615,38.6875,-105.5));
#7259=CARTESIAN_POINT('Ctrl Pts',(74.5997654151808,38.625,-74.5997654151808));
#7260=CARTESIAN_POINT('Ctrl Pts',(105.5,38.5625,-43.6995308303616));
#7261=CARTESIAN_POINT('Ctrl Pts',(105.5,38.5,-1.29200237310046E-14));
#7262=CARTESIAN_POINT('Ctrl Pts',(105.5,38.4375,43.6995308303615));
#7263=CARTESIAN_POINT('Ctrl Pts',(74.5997654151808,38.375,74.5997654151808));
#7264=CARTESIAN_POINT('Ctrl Pts',(43.6995308303616,38.3125,105.5));
#7265=CARTESIAN_POINT('Ctrl Pts',(1.93800355965069E-14,38.25,105.5));
#7266=CARTESIAN_POINT('Ctrl Pts',(1.93800355965069E-14,39.3750000027312,
105.5));
#7267=CARTESIAN_POINT('Ctrl Pts',(-43.6995308303616,39.3125000027312,105.5));
#7268=CARTESIAN_POINT('Ctrl Pts',(-74.5997654151808,39.2500000027312,74.5997654151808));
#7269=CARTESIAN_POINT('Ctrl Pts',(-105.5,39.1875000027312,43.6995308303616));
#7270=CARTESIAN_POINT('Ctrl Pts',(-105.5,39.1250000027312,0.));
#7271=CARTESIAN_POINT('Ctrl Pts',(-105.5,39.0625000027312,-43.6995308303615));
#7272=CARTESIAN_POINT('Ctrl Pts',(-74.5997654151808,39.0000000027312,-74.5997654151808));
#7273=CARTESIAN_POINT('Ctrl Pts',(-43.6995308303615,38.9375000027312,-105.5));
#7274=CARTESIAN_POINT('Ctrl Pts',(-6.46001186550229E-15,38.8750000027312,
-105.5));
#7275=CARTESIAN_POINT('Ctrl Pts',(43.6995308303615,38.8125000027312,-105.5));
#7276=CARTESIAN_POINT('Ctrl Pts',(74.5997654151808,38.7500000027312,-74.5997654151808));
#7277=CARTESIAN_POINT('Ctrl Pts',(105.5,38.6875000027312,-43.6995308303616));
#7278=CARTESIAN_POINT('Ctrl Pts',(105.5,38.6250000027312,-1.29200237310046E-14));
#7279=CARTESIAN_POINT('Ctrl Pts',(105.5,38.5625000027312,43.6995308303615));
#7280=CARTESIAN_POINT('Ctrl Pts',(74.5997654151808,38.5000000027312,74.5997654151808));
#7281=CARTESIAN_POINT('Ctrl Pts',(43.6995308303616,38.4375000027312,105.5));
#7282=CARTESIAN_POINT('Ctrl Pts',(1.93800355965069E-14,38.3750000027312,
105.5));
#7283=CARTESIAN_POINT('Origin',(0.,105.,0.));
#7284=CARTESIAN_POINT('',(3.23000593275114E-15,40.3750000027312,105.5));
#7285=CARTESIAN_POINT('',(3.23000593275114E-15,40.25,105.5));
#7286=CARTESIAN_POINT('',(-1.29200237310046E-14,105.,105.5));
#7287=CARTESIAN_POINT('Ctrl Pts',(1.93800355965069E-14,40.25,105.5));
#7288=CARTESIAN_POINT('Ctrl Pts',(-43.6995308303616,40.1875,105.5));
#7289=CARTESIAN_POINT('Ctrl Pts',(-74.5997654151808,40.125,74.5997654151808));
#7290=CARTESIAN_POINT('Ctrl Pts',(-105.5,40.0625,43.6995308303616));
#7291=CARTESIAN_POINT('Ctrl Pts',(-105.5,40.,0.));
#7292=CARTESIAN_POINT('Ctrl Pts',(-105.5,39.9375,-43.6995308303615));
#7293=CARTESIAN_POINT('Ctrl Pts',(-74.5997654151808,39.875,-74.5997654151808));
#7294=CARTESIAN_POINT('Ctrl Pts',(-43.6995308303615,39.8125,-105.5));
#7295=CARTESIAN_POINT('Ctrl Pts',(-6.46001186550229E-15,39.75,-105.5));
#7296=CARTESIAN_POINT('Ctrl Pts',(43.6995308303615,39.6875,-105.5));
#7297=CARTESIAN_POINT('Ctrl Pts',(74.5997654151808,39.625,-74.5997654151808));
#7298=CARTESIAN_POINT('Ctrl Pts',(105.5,39.5625,-43.6995308303616));
#7299=CARTESIAN_POINT('Ctrl Pts',(105.5,39.5,-1.29200237310046E-14));
#7300=CARTESIAN_POINT('Ctrl Pts',(105.5,39.4375,43.6995308303615));
#7301=CARTESIAN_POINT('Ctrl Pts',(74.5997654151808,39.375,74.5997654151808));
#7302=CARTESIAN_POINT('Ctrl Pts',(43.6995308303616,39.3125,105.5));
#7303=CARTESIAN_POINT('Ctrl Pts',(1.93800355965069E-14,39.25,105.5));
#7304=CARTESIAN_POINT('Ctrl Pts',(1.93800355965069E-14,40.3750000027312,
105.5));
#7305=CARTESIAN_POINT('Ctrl Pts',(-43.6995308303616,40.3125000027312,105.5));
#7306=CARTESIAN_POINT('Ctrl Pts',(-74.5997654151808,40.2500000027312,74.5997654151808));
#7307=CARTESIAN_POINT('Ctrl Pts',(-105.5,40.1875000027312,43.6995308303616));
#7308=CARTESIAN_POINT('Ctrl Pts',(-105.5,40.1250000027312,0.));
#7309=CARTESIAN_POINT('Ctrl Pts',(-105.5,40.0625000027312,-43.6995308303615));
#7310=CARTESIAN_POINT('Ctrl Pts',(-74.5997654151808,40.0000000027312,-74.5997654151808));
#7311=CARTESIAN_POINT('Ctrl Pts',(-43.6995308303615,39.9375000027312,-105.5));
#7312=CARTESIAN_POINT('Ctrl Pts',(-6.46001186550229E-15,39.8750000027312,
-105.5));
#7313=CARTESIAN_POINT('Ctrl Pts',(43.6995308303615,39.8125000027312,-105.5));
#7314=CARTESIAN_POINT('Ctrl Pts',(74.5997654151808,39.7500000027312,-74.5997654151808));
#7315=CARTESIAN_POINT('Ctrl Pts',(105.5,39.6875000027312,-43.6995308303616));
#7316=CARTESIAN_POINT('Ctrl Pts',(105.5,39.6250000027312,-1.29200237310046E-14));
#7317=CARTESIAN_POINT('Ctrl Pts',(105.5,39.5625000027312,43.6995308303615));
#7318=CARTESIAN_POINT('Ctrl Pts',(74.5997654151808,39.5000000027312,74.5997654151808));
#7319=CARTESIAN_POINT('Ctrl Pts',(43.6995308303616,39.4375000027312,105.5));
#7320=CARTESIAN_POINT('Ctrl Pts',(1.93800355965069E-14,39.3750000027312,
105.5));
#7321=CARTESIAN_POINT('Origin',(0.,105.,0.));
#7322=CARTESIAN_POINT('',(3.23000593275114E-15,41.3750000027312,105.5));
#7323=CARTESIAN_POINT('',(3.23000593275114E-15,41.25,105.5));
#7324=CARTESIAN_POINT('',(-1.29200237310046E-14,105.,105.5));
#7325=CARTESIAN_POINT('Ctrl Pts',(1.93800355965069E-14,41.25,105.5));
#7326=CARTESIAN_POINT('Ctrl Pts',(-43.6995308303616,41.1875,105.5));
#7327=CARTESIAN_POINT('Ctrl Pts',(-74.5997654151808,41.125,74.5997654151808));
#7328=CARTESIAN_POINT('Ctrl Pts',(-105.5,41.0625,43.6995308303616));
#7329=CARTESIAN_POINT('Ctrl Pts',(-105.5,41.,0.));
#7330=CARTESIAN_POINT('Ctrl Pts',(-105.5,40.9375,-43.6995308303615));
#7331=CARTESIAN_POINT('Ctrl Pts',(-74.5997654151808,40.875,-74.5997654151808));
#7332=CARTESIAN_POINT('Ctrl Pts',(-43.6995308303615,40.8125,-105.5));
#7333=CARTESIAN_POINT('Ctrl Pts',(-6.46001186550229E-15,40.75,-105.5));
#7334=CARTESIAN_POINT('Ctrl Pts',(43.6995308303615,40.6875,-105.5));
#7335=CARTESIAN_POINT('Ctrl Pts',(74.5997654151808,40.625,-74.5997654151808));
#7336=CARTESIAN_POINT('Ctrl Pts',(105.5,40.5625,-43.6995308303616));
#7337=CARTESIAN_POINT('Ctrl Pts',(105.5,40.5,-1.29200237310046E-14));
#7338=CARTESIAN_POINT('Ctrl Pts',(105.5,40.4375,43.6995308303615));
#7339=CARTESIAN_POINT('Ctrl Pts',(74.5997654151808,40.375,74.5997654151808));
#7340=CARTESIAN_POINT('Ctrl Pts',(43.6995308303616,40.3125,105.5));
#7341=CARTESIAN_POINT('Ctrl Pts',(1.93800355965069E-14,40.25,105.5));
#7342=CARTESIAN_POINT('Ctrl Pts',(1.93800355965069E-14,41.3750000027312,
105.5));
#7343=CARTESIAN_POINT('Ctrl Pts',(-43.6995308303616,41.3125000027312,105.5));
#7344=CARTESIAN_POINT('Ctrl Pts',(-74.5997654151808,41.2500000027312,74.5997654151808));
#7345=CARTESIAN_POINT('Ctrl Pts',(-105.5,41.1875000027312,43.6995308303616));
#7346=CARTESIAN_POINT('Ctrl Pts',(-105.5,41.1250000027312,0.));
#7347=CARTESIAN_POINT('Ctrl Pts',(-105.5,41.0625000027312,-43.6995308303615));
#7348=CARTESIAN_POINT('Ctrl Pts',(-74.5997654151808,41.0000000027312,-74.5997654151808));
#7349=CARTESIAN_POINT('Ctrl Pts',(-43.6995308303615,40.9375000027312,-105.5));
#7350=CARTESIAN_POINT('Ctrl Pts',(-6.46001186550229E-15,40.8750000027312,
-105.5));
#7351=CARTESIAN_POINT('Ctrl Pts',(43.6995308303615,40.8125000027312,-105.5));
#7352=CARTESIAN_POINT('Ctrl Pts',(74.5997654151808,40.7500000027312,-74.5997654151808));
#7353=CARTESIAN_POINT('Ctrl Pts',(105.5,40.6875000027312,-43.6995308303616));
#7354=CARTESIAN_POINT('Ctrl Pts',(105.5,40.6250000027312,-1.29200237310046E-14));
#7355=CARTESIAN_POINT('Ctrl Pts',(105.5,40.5625000027312,43.6995308303615));
#7356=CARTESIAN_POINT('Ctrl Pts',(74.5997654151808,40.5000000027312,74.5997654151808));
#7357=CARTESIAN_POINT('Ctrl Pts',(43.6995308303616,40.4375000027312,105.5));
#7358=CARTESIAN_POINT('Ctrl Pts',(1.93800355965069E-14,40.3750000027312,
105.5));
#7359=CARTESIAN_POINT('Origin',(0.,105.,0.));
#7360=CARTESIAN_POINT('',(3.23000593275114E-15,42.3750000027312,105.5));
#7361=CARTESIAN_POINT('',(3.23000593275114E-15,42.25,105.5));
#7362=CARTESIAN_POINT('',(-1.29200237310046E-14,105.,105.5));
#7363=CARTESIAN_POINT('Ctrl Pts',(1.93800355965069E-14,42.25,105.5));
#7364=CARTESIAN_POINT('Ctrl Pts',(-43.6995308303616,42.1875,105.5));
#7365=CARTESIAN_POINT('Ctrl Pts',(-74.5997654151808,42.125,74.5997654151808));
#7366=CARTESIAN_POINT('Ctrl Pts',(-105.5,42.0625,43.6995308303616));
#7367=CARTESIAN_POINT('Ctrl Pts',(-105.5,42.,0.));
#7368=CARTESIAN_POINT('Ctrl Pts',(-105.5,41.9375,-43.6995308303615));
#7369=CARTESIAN_POINT('Ctrl Pts',(-74.5997654151808,41.875,-74.5997654151808));
#7370=CARTESIAN_POINT('Ctrl Pts',(-43.6995308303615,41.8125,-105.5));
#7371=CARTESIAN_POINT('Ctrl Pts',(-6.46001186550229E-15,41.75,-105.5));
#7372=CARTESIAN_POINT('Ctrl Pts',(43.6995308303615,41.6875,-105.5));
#7373=CARTESIAN_POINT('Ctrl Pts',(74.5997654151808,41.625,-74.5997654151808));
#7374=CARTESIAN_POINT('Ctrl Pts',(105.5,41.5625,-43.6995308303616));
#7375=CARTESIAN_POINT('Ctrl Pts',(105.5,41.5,-1.29200237310046E-14));
#7376=CARTESIAN_POINT('Ctrl Pts',(105.5,41.4375,43.6995308303615));
#7377=CARTESIAN_POINT('Ctrl Pts',(74.5997654151808,41.375,74.5997654151808));
#7378=CARTESIAN_POINT('Ctrl Pts',(43.6995308303616,41.3125,105.5));
#7379=CARTESIAN_POINT('Ctrl Pts',(1.93800355965069E-14,41.25,105.5));
#7380=CARTESIAN_POINT('Ctrl Pts',(1.93800355965069E-14,42.3750000027312,
105.5));
#7381=CARTESIAN_POINT('Ctrl Pts',(-43.6995308303616,42.3125000027312,105.5));
#7382=CARTESIAN_POINT('Ctrl Pts',(-74.5997654151808,42.2500000027312,74.5997654151808));
#7383=CARTESIAN_POINT('Ctrl Pts',(-105.5,42.1875000027312,43.6995308303616));
#7384=CARTESIAN_POINT('Ctrl Pts',(-105.5,42.1250000027312,0.));
#7385=CARTESIAN_POINT('Ctrl Pts',(-105.5,42.0625000027312,-43.6995308303615));
#7386=CARTESIAN_POINT('Ctrl Pts',(-74.5997654151808,42.0000000027312,-74.5997654151808));
#7387=CARTESIAN_POINT('Ctrl Pts',(-43.6995308303615,41.9375000027312,-105.5));
#7388=CARTESIAN_POINT('Ctrl Pts',(-6.46001186550229E-15,41.8750000027312,
-105.5));
#7389=CARTESIAN_POINT('Ctrl Pts',(43.6995308303615,41.8125000027312,-105.5));
#7390=CARTESIAN_POINT('Ctrl Pts',(74.5997654151808,41.7500000027312,-74.5997654151808));
#7391=CARTESIAN_POINT('Ctrl Pts',(105.5,41.6875000027312,-43.6995308303616));
#7392=CARTESIAN_POINT('Ctrl Pts',(105.5,41.6250000027312,-1.29200237310046E-14));
#7393=CARTESIAN_POINT('Ctrl Pts',(105.5,41.5625000027312,43.6995308303615));
#7394=CARTESIAN_POINT('Ctrl Pts',(74.5997654151808,41.5000000027312,74.5997654151808));
#7395=CARTESIAN_POINT('Ctrl Pts',(43.6995308303616,41.4375000027312,105.5));
#7396=CARTESIAN_POINT('Ctrl Pts',(1.93800355965069E-14,41.3750000027312,
105.5));
#7397=CARTESIAN_POINT('Origin',(0.,105.,0.));
#7398=CARTESIAN_POINT('',(3.23000593275114E-15,43.3750000027312,105.5));
#7399=CARTESIAN_POINT('',(3.23000593275114E-15,43.25,105.5));
#7400=CARTESIAN_POINT('',(-1.29200237310046E-14,105.,105.5));
#7401=CARTESIAN_POINT('Ctrl Pts',(1.93800355965069E-14,43.25,105.5));
#7402=CARTESIAN_POINT('Ctrl Pts',(-43.6995308303616,43.1875,105.5));
#7403=CARTESIAN_POINT('Ctrl Pts',(-74.5997654151808,43.125,74.5997654151808));
#7404=CARTESIAN_POINT('Ctrl Pts',(-105.5,43.0625,43.6995308303616));
#7405=CARTESIAN_POINT('Ctrl Pts',(-105.5,43.,0.));
#7406=CARTESIAN_POINT('Ctrl Pts',(-105.5,42.9375,-43.6995308303615));
#7407=CARTESIAN_POINT('Ctrl Pts',(-74.5997654151808,42.875,-74.5997654151808));
#7408=CARTESIAN_POINT('Ctrl Pts',(-43.6995308303615,42.8125,-105.5));
#7409=CARTESIAN_POINT('Ctrl Pts',(-6.46001186550229E-15,42.75,-105.5));
#7410=CARTESIAN_POINT('Ctrl Pts',(43.6995308303615,42.6875,-105.5));
#7411=CARTESIAN_POINT('Ctrl Pts',(74.5997654151808,42.625,-74.5997654151808));
#7412=CARTESIAN_POINT('Ctrl Pts',(105.5,42.5625,-43.6995308303616));
#7413=CARTESIAN_POINT('Ctrl Pts',(105.5,42.5,-1.29200237310046E-14));
#7414=CARTESIAN_POINT('Ctrl Pts',(105.5,42.4375,43.6995308303615));
#7415=CARTESIAN_POINT('Ctrl Pts',(74.5997654151808,42.375,74.5997654151808));
#7416=CARTESIAN_POINT('Ctrl Pts',(43.6995308303616,42.3125,105.5));
#7417=CARTESIAN_POINT('Ctrl Pts',(1.93800355965069E-14,42.25,105.5));
#7418=CARTESIAN_POINT('Ctrl Pts',(1.93800355965069E-14,43.3750000027312,
105.5));
#7419=CARTESIAN_POINT('Ctrl Pts',(-43.6995308303616,43.3125000027312,105.5));
#7420=CARTESIAN_POINT('Ctrl Pts',(-74.5997654151808,43.2500000027312,74.5997654151808));
#7421=CARTESIAN_POINT('Ctrl Pts',(-105.5,43.1875000027312,43.6995308303616));
#7422=CARTESIAN_POINT('Ctrl Pts',(-105.5,43.1250000027312,0.));
#7423=CARTESIAN_POINT('Ctrl Pts',(-105.5,43.0625000027312,-43.6995308303615));
#7424=CARTESIAN_POINT('Ctrl Pts',(-74.5997654151808,43.0000000027312,-74.5997654151808));
#7425=CARTESIAN_POINT('Ctrl Pts',(-43.6995308303615,42.9375000027312,-105.5));
#7426=CARTESIAN_POINT('Ctrl Pts',(-6.46001186550229E-15,42.8750000027312,
-105.5));
#7427=CARTESIAN_POINT('Ctrl Pts',(43.6995308303615,42.8125000027312,-105.5));
#7428=CARTESIAN_POINT('Ctrl Pts',(74.5997654151808,42.7500000027312,-74.5997654151808));
#7429=CARTESIAN_POINT('Ctrl Pts',(105.5,42.6875000027312,-43.6995308303616));
#7430=CARTESIAN_POINT('Ctrl Pts',(105.5,42.6250000027312,-1.29200237310046E-14));
#7431=CARTESIAN_POINT('Ctrl Pts',(105.5,42.5625000027312,43.6995308303615));
#7432=CARTESIAN_POINT('Ctrl Pts',(74.5997654151808,42.5000000027312,74.5997654151808));
#7433=CARTESIAN_POINT('Ctrl Pts',(43.6995308303616,42.4375000027312,105.5));
#7434=CARTESIAN_POINT('Ctrl Pts',(1.93800355965069E-14,42.3750000027312,
105.5));
#7435=CARTESIAN_POINT('Origin',(0.,105.,0.));
#7436=CARTESIAN_POINT('',(3.23000593275114E-15,44.3750000027312,105.5));
#7437=CARTESIAN_POINT('',(3.23000593275114E-15,44.25,105.5));
#7438=CARTESIAN_POINT('',(-1.29200237310046E-14,105.,105.5));
#7439=CARTESIAN_POINT('Ctrl Pts',(1.93800355965069E-14,44.25,105.5));
#7440=CARTESIAN_POINT('Ctrl Pts',(-43.6995308303616,44.1875,105.5));
#7441=CARTESIAN_POINT('Ctrl Pts',(-74.5997654151808,44.125,74.5997654151808));
#7442=CARTESIAN_POINT('Ctrl Pts',(-105.5,44.0625,43.6995308303616));
#7443=CARTESIAN_POINT('Ctrl Pts',(-105.5,44.,0.));
#7444=CARTESIAN_POINT('Ctrl Pts',(-105.5,43.9375,-43.6995308303615));
#7445=CARTESIAN_POINT('Ctrl Pts',(-74.5997654151808,43.875,-74.5997654151808));
#7446=CARTESIAN_POINT('Ctrl Pts',(-43.6995308303615,43.8125,-105.5));
#7447=CARTESIAN_POINT('Ctrl Pts',(-6.46001186550229E-15,43.75,-105.5));
#7448=CARTESIAN_POINT('Ctrl Pts',(43.6995308303615,43.6875,-105.5));
#7449=CARTESIAN_POINT('Ctrl Pts',(74.5997654151808,43.625,-74.5997654151808));
#7450=CARTESIAN_POINT('Ctrl Pts',(105.5,43.5625,-43.6995308303616));
#7451=CARTESIAN_POINT('Ctrl Pts',(105.5,43.5,-1.29200237310046E-14));
#7452=CARTESIAN_POINT('Ctrl Pts',(105.5,43.4375,43.6995308303615));
#7453=CARTESIAN_POINT('Ctrl Pts',(74.5997654151808,43.375,74.5997654151808));
#7454=CARTESIAN_POINT('Ctrl Pts',(43.6995308303616,43.3125,105.5));
#7455=CARTESIAN_POINT('Ctrl Pts',(1.93800355965069E-14,43.25,105.5));
#7456=CARTESIAN_POINT('Ctrl Pts',(1.93800355965069E-14,44.3750000027312,
105.5));
#7457=CARTESIAN_POINT('Ctrl Pts',(-43.6995308303616,44.3125000027312,105.5));
#7458=CARTESIAN_POINT('Ctrl Pts',(-74.5997654151808,44.2500000027312,74.5997654151808));
#7459=CARTESIAN_POINT('Ctrl Pts',(-105.5,44.1875000027312,43.6995308303616));
#7460=CARTESIAN_POINT('Ctrl Pts',(-105.5,44.1250000027312,0.));
#7461=CARTESIAN_POINT('Ctrl Pts',(-105.5,44.0625000027312,-43.6995308303615));
#7462=CARTESIAN_POINT('Ctrl Pts',(-74.5997654151808,44.0000000027312,-74.5997654151808));
#7463=CARTESIAN_POINT('Ctrl Pts',(-43.6995308303615,43.9375000027312,-105.5));
#7464=CARTESIAN_POINT('Ctrl Pts',(-6.46001186550229E-15,43.8750000027312,
-105.5));
#7465=CARTESIAN_POINT('Ctrl Pts',(43.6995308303615,43.8125000027312,-105.5));
#7466=CARTESIAN_POINT('Ctrl Pts',(74.5997654151808,43.7500000027312,-74.5997654151808));
#7467=CARTESIAN_POINT('Ctrl Pts',(105.5,43.6875000027312,-43.6995308303616));
#7468=CARTESIAN_POINT('Ctrl Pts',(105.5,43.6250000027312,-1.29200237310046E-14));
#7469=CARTESIAN_POINT('Ctrl Pts',(105.5,43.5625000027312,43.6995308303615));
#7470=CARTESIAN_POINT('Ctrl Pts',(74.5997654151808,43.5000000027312,74.5997654151808));
#7471=CARTESIAN_POINT('Ctrl Pts',(43.6995308303616,43.4375000027312,105.5));
#7472=CARTESIAN_POINT('Ctrl Pts',(1.93800355965069E-14,43.3750000027312,
105.5));
#7473=CARTESIAN_POINT('Origin',(0.,105.,0.));
#7474=CARTESIAN_POINT('',(3.23000593275114E-15,45.3750000027312,105.5));
#7475=CARTESIAN_POINT('',(3.23000593275114E-15,45.25,105.5));
#7476=CARTESIAN_POINT('',(-1.29200237310046E-14,105.,105.5));
#7477=CARTESIAN_POINT('Ctrl Pts',(1.93800355965069E-14,45.25,105.5));
#7478=CARTESIAN_POINT('Ctrl Pts',(-43.6995308303616,45.1875,105.5));
#7479=CARTESIAN_POINT('Ctrl Pts',(-74.5997654151808,45.125,74.5997654151808));
#7480=CARTESIAN_POINT('Ctrl Pts',(-105.5,45.0625,43.6995308303616));
#7481=CARTESIAN_POINT('Ctrl Pts',(-105.5,45.,0.));
#7482=CARTESIAN_POINT('Ctrl Pts',(-105.5,44.9375,-43.6995308303615));
#7483=CARTESIAN_POINT('Ctrl Pts',(-74.5997654151808,44.875,-74.5997654151808));
#7484=CARTESIAN_POINT('Ctrl Pts',(-43.6995308303615,44.8125,-105.5));
#7485=CARTESIAN_POINT('Ctrl Pts',(-6.46001186550229E-15,44.75,-105.5));
#7486=CARTESIAN_POINT('Ctrl Pts',(43.6995308303615,44.6875,-105.5));
#7487=CARTESIAN_POINT('Ctrl Pts',(74.5997654151808,44.625,-74.5997654151808));
#7488=CARTESIAN_POINT('Ctrl Pts',(105.5,44.5625,-43.6995308303616));
#7489=CARTESIAN_POINT('Ctrl Pts',(105.5,44.5,-1.29200237310046E-14));
#7490=CARTESIAN_POINT('Ctrl Pts',(105.5,44.4375,43.6995308303615));
#7491=CARTESIAN_POINT('Ctrl Pts',(74.5997654151808,44.375,74.5997654151808));
#7492=CARTESIAN_POINT('Ctrl Pts',(43.6995308303616,44.3125,105.5));
#7493=CARTESIAN_POINT('Ctrl Pts',(1.93800355965069E-14,44.25,105.5));
#7494=CARTESIAN_POINT('Ctrl Pts',(1.93800355965069E-14,45.3750000027312,
105.5));
#7495=CARTESIAN_POINT('Ctrl Pts',(-43.6995308303616,45.3125000027312,105.5));
#7496=CARTESIAN_POINT('Ctrl Pts',(-74.5997654151808,45.2500000027312,74.5997654151808));
#7497=CARTESIAN_POINT('Ctrl Pts',(-105.5,45.1875000027312,43.6995308303616));
#7498=CARTESIAN_POINT('Ctrl Pts',(-105.5,45.1250000027312,0.));
#7499=CARTESIAN_POINT('Ctrl Pts',(-105.5,45.0625000027312,-43.6995308303615));
#7500=CARTESIAN_POINT('Ctrl Pts',(-74.5997654151808,45.0000000027312,-74.5997654151808));
#7501=CARTESIAN_POINT('Ctrl Pts',(-43.6995308303615,44.9375000027312,-105.5));
#7502=CARTESIAN_POINT('Ctrl Pts',(-6.46001186550229E-15,44.8750000027312,
-105.5));
#7503=CARTESIAN_POINT('Ctrl Pts',(43.6995308303615,44.8125000027312,-105.5));
#7504=CARTESIAN_POINT('Ctrl Pts',(74.5997654151808,44.7500000027312,-74.5997654151808));
#7505=CARTESIAN_POINT('Ctrl Pts',(105.5,44.6875000027312,-43.6995308303616));
#7506=CARTESIAN_POINT('Ctrl Pts',(105.5,44.6250000027312,-1.29200237310046E-14));
#7507=CARTESIAN_POINT('Ctrl Pts',(105.5,44.5625000027312,43.6995308303615));
#7508=CARTESIAN_POINT('Ctrl Pts',(74.5997654151808,44.5000000027312,74.5997654151808));
#7509=CARTESIAN_POINT('Ctrl Pts',(43.6995308303616,44.4375000027312,105.5));
#7510=CARTESIAN_POINT('Ctrl Pts',(1.93800355965069E-14,44.3750000027312,
105.5));
#7511=CARTESIAN_POINT('Origin',(0.,105.,0.));
#7512=CARTESIAN_POINT('',(3.23000593275114E-15,46.3750000027312,105.5));
#7513=CARTESIAN_POINT('',(3.23000593275114E-15,46.25,105.5));
#7514=CARTESIAN_POINT('',(-1.29200237310046E-14,105.,105.5));
#7515=CARTESIAN_POINT('Ctrl Pts',(1.93800355965069E-14,46.25,105.5));
#7516=CARTESIAN_POINT('Ctrl Pts',(-43.6995308303616,46.1875,105.5));
#7517=CARTESIAN_POINT('Ctrl Pts',(-74.5997654151808,46.125,74.5997654151808));
#7518=CARTESIAN_POINT('Ctrl Pts',(-105.5,46.0625,43.6995308303616));
#7519=CARTESIAN_POINT('Ctrl Pts',(-105.5,46.,0.));
#7520=CARTESIAN_POINT('Ctrl Pts',(-105.5,45.9375,-43.6995308303615));
#7521=CARTESIAN_POINT('Ctrl Pts',(-74.5997654151808,45.875,-74.5997654151808));
#7522=CARTESIAN_POINT('Ctrl Pts',(-43.6995308303615,45.8125,-105.5));
#7523=CARTESIAN_POINT('Ctrl Pts',(-6.46001186550229E-15,45.75,-105.5));
#7524=CARTESIAN_POINT('Ctrl Pts',(43.6995308303615,45.6875,-105.5));
#7525=CARTESIAN_POINT('Ctrl Pts',(74.5997654151808,45.625,-74.5997654151808));
#7526=CARTESIAN_POINT('Ctrl Pts',(105.5,45.5625,-43.6995308303616));
#7527=CARTESIAN_POINT('Ctrl Pts',(105.5,45.5,-1.29200237310046E-14));
#7528=CARTESIAN_POINT('Ctrl Pts',(105.5,45.4375,43.6995308303615));
#7529=CARTESIAN_POINT('Ctrl Pts',(74.5997654151808,45.375,74.5997654151808));
#7530=CARTESIAN_POINT('Ctrl Pts',(43.6995308303616,45.3125,105.5));
#7531=CARTESIAN_POINT('Ctrl Pts',(1.93800355965069E-14,45.25,105.5));
#7532=CARTESIAN_POINT('Ctrl Pts',(1.93800355965069E-14,46.3750000027312,
105.5));
#7533=CARTESIAN_POINT('Ctrl Pts',(-43.6995308303616,46.3125000027312,105.5));
#7534=CARTESIAN_POINT('Ctrl Pts',(-74.5997654151808,46.2500000027312,74.5997654151808));
#7535=CARTESIAN_POINT('Ctrl Pts',(-105.5,46.1875000027312,43.6995308303616));
#7536=CARTESIAN_POINT('Ctrl Pts',(-105.5,46.1250000027312,0.));
#7537=CARTESIAN_POINT('Ctrl Pts',(-105.5,46.0625000027312,-43.6995308303615));
#7538=CARTESIAN_POINT('Ctrl Pts',(-74.5997654151808,46.0000000027312,-74.5997654151808));
#7539=CARTESIAN_POINT('Ctrl Pts',(-43.6995308303615,45.9375000027312,-105.5));
#7540=CARTESIAN_POINT('Ctrl Pts',(-6.46001186550229E-15,45.8750000027312,
-105.5));
#7541=CARTESIAN_POINT('Ctrl Pts',(43.6995308303615,45.8125000027312,-105.5));
#7542=CARTESIAN_POINT('Ctrl Pts',(74.5997654151808,45.7500000027312,-74.5997654151808));
#7543=CARTESIAN_POINT('Ctrl Pts',(105.5,45.6875000027312,-43.6995308303616));
#7544=CARTESIAN_POINT('Ctrl Pts',(105.5,45.6250000027312,-1.29200237310046E-14));
#7545=CARTESIAN_POINT('Ctrl Pts',(105.5,45.5625000027312,43.6995308303615));
#7546=CARTESIAN_POINT('Ctrl Pts',(74.5997654151808,45.5000000027312,74.5997654151808));
#7547=CARTESIAN_POINT('Ctrl Pts',(43.6995308303616,45.4375000027312,105.5));
#7548=CARTESIAN_POINT('Ctrl Pts',(1.93800355965069E-14,45.3750000027312,
105.5));
#7549=CARTESIAN_POINT('Origin',(0.,105.,0.));
#7550=CARTESIAN_POINT('',(3.23000593275114E-15,47.3750000027312,105.5));
#7551=CARTESIAN_POINT('',(3.23000593275114E-15,47.25,105.5));
#7552=CARTESIAN_POINT('',(-1.29200237310046E-14,105.,105.5));
#7553=CARTESIAN_POINT('Ctrl Pts',(1.93800355965069E-14,47.25,105.5));
#7554=CARTESIAN_POINT('Ctrl Pts',(-43.6995308303616,47.1875,105.5));
#7555=CARTESIAN_POINT('Ctrl Pts',(-74.5997654151808,47.125,74.5997654151808));
#7556=CARTESIAN_POINT('Ctrl Pts',(-105.5,47.0625,43.6995308303616));
#7557=CARTESIAN_POINT('Ctrl Pts',(-105.5,47.,0.));
#7558=CARTESIAN_POINT('Ctrl Pts',(-105.5,46.9375,-43.6995308303615));
#7559=CARTESIAN_POINT('Ctrl Pts',(-74.5997654151808,46.875,-74.5997654151808));
#7560=CARTESIAN_POINT('Ctrl Pts',(-43.6995308303615,46.8125,-105.5));
#7561=CARTESIAN_POINT('Ctrl Pts',(-6.46001186550229E-15,46.75,-105.5));
#7562=CARTESIAN_POINT('Ctrl Pts',(43.6995308303615,46.6875,-105.5));
#7563=CARTESIAN_POINT('Ctrl Pts',(74.5997654151808,46.625,-74.5997654151808));
#7564=CARTESIAN_POINT('Ctrl Pts',(105.5,46.5625,-43.6995308303616));
#7565=CARTESIAN_POINT('Ctrl Pts',(105.5,46.5,-1.29200237310046E-14));
#7566=CARTESIAN_POINT('Ctrl Pts',(105.5,46.4375,43.6995308303615));
#7567=CARTESIAN_POINT('Ctrl Pts',(74.5997654151808,46.375,74.5997654151808));
#7568=CARTESIAN_POINT('Ctrl Pts',(43.6995308303616,46.3125,105.5));
#7569=CARTESIAN_POINT('Ctrl Pts',(1.93800355965069E-14,46.25,105.5));
#7570=CARTESIAN_POINT('Ctrl Pts',(1.93800355965069E-14,47.3750000027312,
105.5));
#7571=CARTESIAN_POINT('Ctrl Pts',(-43.6995308303616,47.3125000027312,105.5));
#7572=CARTESIAN_POINT('Ctrl Pts',(-74.5997654151808,47.2500000027312,74.5997654151808));
#7573=CARTESIAN_POINT('Ctrl Pts',(-105.5,47.1875000027312,43.6995308303616));
#7574=CARTESIAN_POINT('Ctrl Pts',(-105.5,47.1250000027312,0.));
#7575=CARTESIAN_POINT('Ctrl Pts',(-105.5,47.0625000027312,-43.6995308303615));
#7576=CARTESIAN_POINT('Ctrl Pts',(-74.5997654151808,47.0000000027312,-74.5997654151808));
#7577=CARTESIAN_POINT('Ctrl Pts',(-43.6995308303615,46.9375000027312,-105.5));
#7578=CARTESIAN_POINT('Ctrl Pts',(-6.46001186550229E-15,46.8750000027312,
-105.5));
#7579=CARTESIAN_POINT('Ctrl Pts',(43.6995308303615,46.8125000027312,-105.5));
#7580=CARTESIAN_POINT('Ctrl Pts',(74.5997654151808,46.7500000027312,-74.5997654151808));
#7581=CARTESIAN_POINT('Ctrl Pts',(105.5,46.6875000027312,-43.6995308303616));
#7582=CARTESIAN_POINT('Ctrl Pts',(105.5,46.6250000027312,-1.29200237310046E-14));
#7583=CARTESIAN_POINT('Ctrl Pts',(105.5,46.5625000027312,43.6995308303615));
#7584=CARTESIAN_POINT('Ctrl Pts',(74.5997654151808,46.5000000027312,74.5997654151808));
#7585=CARTESIAN_POINT('Ctrl Pts',(43.6995308303616,46.4375000027312,105.5));
#7586=CARTESIAN_POINT('Ctrl Pts',(1.93800355965069E-14,46.3750000027312,
105.5));
#7587=CARTESIAN_POINT('Origin',(0.,105.,0.));
#7588=CARTESIAN_POINT('',(0.,100.,105.5));
#7589=CARTESIAN_POINT('Origin',(0.,100.,0.));
#7590=CARTESIAN_POINT('',(3.23000593275114E-15,49.25,105.5));
#7591=CARTESIAN_POINT('',(-1.29200237310046E-14,105.,105.5));
#7592=CARTESIAN_POINT('',(3.23000593275114E-15,48.25,105.5));
#7593=CARTESIAN_POINT('Ctrl Pts',(1.93800355965069E-14,49.25,105.5));
#7594=CARTESIAN_POINT('Ctrl Pts',(-43.6995308303616,49.1875,105.5));
#7595=CARTESIAN_POINT('Ctrl Pts',(-74.5997654151808,49.125,74.5997654151808));
#7596=CARTESIAN_POINT('Ctrl Pts',(-105.5,49.0625,43.6995308303616));
#7597=CARTESIAN_POINT('Ctrl Pts',(-105.5,49.,0.));
#7598=CARTESIAN_POINT('Ctrl Pts',(-105.5,48.9375,-43.6995308303615));
#7599=CARTESIAN_POINT('Ctrl Pts',(-74.5997654151808,48.875,-74.5997654151808));
#7600=CARTESIAN_POINT('Ctrl Pts',(-43.6995308303615,48.8125,-105.5));
#7601=CARTESIAN_POINT('Ctrl Pts',(-6.46001186550229E-15,48.75,-105.5));
#7602=CARTESIAN_POINT('Ctrl Pts',(43.6995308303615,48.6875,-105.5));
#7603=CARTESIAN_POINT('Ctrl Pts',(74.5997654151808,48.625,-74.5997654151808));
#7604=CARTESIAN_POINT('Ctrl Pts',(105.5,48.5625,-43.6995308303616));
#7605=CARTESIAN_POINT('Ctrl Pts',(105.5,48.5,-1.29200237310046E-14));
#7606=CARTESIAN_POINT('Ctrl Pts',(105.5,48.4375,43.6995308303615));
#7607=CARTESIAN_POINT('Ctrl Pts',(74.5997654151808,48.375,74.5997654151808));
#7608=CARTESIAN_POINT('Ctrl Pts',(43.6995308303616,48.3125,105.5));
#7609=CARTESIAN_POINT('Ctrl Pts',(1.93800355965069E-14,48.25,105.5));
#7610=CARTESIAN_POINT('',(3.23000593275114E-15,48.3750000027312,105.5));
#7611=CARTESIAN_POINT('',(-1.29200237310046E-14,105.,105.5));
#7612=CARTESIAN_POINT('',(-105.5,49.1250000027312,0.));
#7613=CARTESIAN_POINT('Ctrl Pts',(-105.5,49.1250000027312,0.));
#7614=CARTESIAN_POINT('Ctrl Pts',(-105.5,49.0625000027312,-43.6995308303615));
#7615=CARTESIAN_POINT('Ctrl Pts',(-74.5997654151808,49.0000000027312,-74.5997654151808));
#7616=CARTESIAN_POINT('Ctrl Pts',(-43.6995308303615,48.9375000027312,-105.5));
#7617=CARTESIAN_POINT('Ctrl Pts',(-6.46001186550229E-15,48.8750000027312,
-105.5));
#7618=CARTESIAN_POINT('Ctrl Pts',(43.6995308303615,48.8125000027312,-105.5));
#7619=CARTESIAN_POINT('Ctrl Pts',(74.5997654151808,48.7500000027312,-74.5997654151808));
#7620=CARTESIAN_POINT('Ctrl Pts',(105.5,48.6875000027312,-43.6995308303616));
#7621=CARTESIAN_POINT('Ctrl Pts',(105.5,48.6250000027312,-1.29200237310046E-14));
#7622=CARTESIAN_POINT('Ctrl Pts',(105.5,48.5625000027312,43.6995308303615));
#7623=CARTESIAN_POINT('Ctrl Pts',(74.5997654151808,48.5000000027312,74.5997654151808));
#7624=CARTESIAN_POINT('Ctrl Pts',(43.6995308303616,48.4375000027312,105.5));
#7625=CARTESIAN_POINT('Ctrl Pts',(1.93800355965069E-14,48.3750000027312,
105.5));
#7626=CARTESIAN_POINT('',(-105.5,50.,0.));
#7627=CARTESIAN_POINT('',(-105.5,50.,0.));
#7628=CARTESIAN_POINT('Ctrl Pts',(-105.5,50.,0.));
#7629=CARTESIAN_POINT('Ctrl Pts',(-105.5,49.9375,-43.6995308303615));
#7630=CARTESIAN_POINT('Ctrl Pts',(-74.5997654151808,49.875,-74.5997654151808));
#7631=CARTESIAN_POINT('Ctrl Pts',(-43.6995308303615,49.8125,-105.5));
#7632=CARTESIAN_POINT('Ctrl Pts',(-6.46001186550229E-15,49.75,-105.5));
#7633=CARTESIAN_POINT('Ctrl Pts',(43.6995308303615,49.6875,-105.5));
#7634=CARTESIAN_POINT('Ctrl Pts',(74.5997654151808,49.625,-74.5997654151808));
#7635=CARTESIAN_POINT('Ctrl Pts',(105.5,49.5625,-43.6995308303616));
#7636=CARTESIAN_POINT('Ctrl Pts',(105.5,49.5,-1.29200237310046E-14));
#7637=CARTESIAN_POINT('Ctrl Pts',(105.5,49.4375,43.6995308303615));
#7638=CARTESIAN_POINT('Ctrl Pts',(74.5997654151808,49.375,74.5997654151808));
#7639=CARTESIAN_POINT('Ctrl Pts',(43.6995308303616,49.3125,105.5));
#7640=CARTESIAN_POINT('Ctrl Pts',(1.93800355965069E-14,49.25,105.5));
#7641=CARTESIAN_POINT('Origin',(0.,105.,0.));
#7642=CARTESIAN_POINT('',(0.,10.0000000000002,120.5));
#7643=CARTESIAN_POINT('',(-1.47569939297256E-14,10.0000000000002,-120.5));
#7644=CARTESIAN_POINT('Origin',(0.,10.0000000000002,0.));
#7645=CARTESIAN_POINT('Origin',(0.,10.0000000000002,0.));
#7646=CARTESIAN_POINT('',(0.,100.,120.5));
#7647=CARTESIAN_POINT('',(-1.47569939297256E-14,105.,120.5));
#7648=CARTESIAN_POINT('Origin',(0.,100.,0.));
#7649=CARTESIAN_POINT('',(120.084345357753,50.,9.99999999999999));
#7650=CARTESIAN_POINT('',(120.084345357753,50.,-9.99999999999999));
#7651=CARTESIAN_POINT('Ctrl Pts',(120.084345357753,50.,9.99999999999999));
#7652=CARTESIAN_POINT('Ctrl Pts',(120.084345357753,48.7437566650744,9.99999999999999));
#7653=CARTESIAN_POINT('Ctrl Pts',(120.10608848982,47.4041746217151,9.74882112932349));
#7654=CARTESIAN_POINT('Ctrl Pts',(120.184575491108,44.9405529209964,8.72810511950586));
#7655=CARTESIAN_POINT('Ctrl Pts',(120.240180997842,43.816464013271,7.95859963700194));
#7656=CARTESIAN_POINT('Ctrl Pts',(120.344523336394,42.0414017916464,6.18353741537737));
#7657=CARTESIAN_POINT('Ctrl Pts',(120.400045183931,41.2718952010862,5.05944787646731));
#7658=CARTESIAN_POINT('Ctrl Pts',(120.478340752227,40.2511783443158,2.59582408417372));
#7659=CARTESIAN_POINT('Ctrl Pts',(120.5,40.,1.25624131276716));
#7660=CARTESIAN_POINT('Ctrl Pts',(120.5,40.,-1.25624131276716));
#7661=CARTESIAN_POINT('Ctrl Pts',(120.478340752227,40.2511783443158,-2.59582408417371));
#7662=CARTESIAN_POINT('Ctrl Pts',(120.400045183931,41.2718952010862,-5.05944787646731));
#7663=CARTESIAN_POINT('Ctrl Pts',(120.344523336394,42.0414017916464,-6.18353741537737));
#7664=CARTESIAN_POINT('Ctrl Pts',(120.240180997842,43.816464013271,-7.95859963700194));
#7665=CARTESIAN_POINT('Ctrl Pts',(120.184575491108,44.9405529209964,-8.72810511950586));
#7666=CARTESIAN_POINT('Ctrl Pts',(120.10608848982,47.4041746217151,-9.74882112932349));
#7667=CARTESIAN_POINT('Ctrl Pts',(120.084345357753,48.7437566650744,-9.99999999999999));
#7668=CARTESIAN_POINT('Ctrl Pts',(120.084345357753,50.,-9.99999999999999));
#7669=CARTESIAN_POINT('Ctrl Pts',(120.084345357753,50.,-9.99999999999999));
#7670=CARTESIAN_POINT('Ctrl Pts',(120.084345357753,51.2562433349256,-9.99999999999999));
#7671=CARTESIAN_POINT('Ctrl Pts',(120.10608848982,52.5958253782849,-9.74882112932349));
#7672=CARTESIAN_POINT('Ctrl Pts',(120.184575491108,55.0594470790036,-8.72810511950586));
#7673=CARTESIAN_POINT('Ctrl Pts',(120.240180997842,56.183535986729,-7.95859963700194));
#7674=CARTESIAN_POINT('Ctrl Pts',(120.344523336394,57.9585982083536,-6.18353741537737));
#7675=CARTESIAN_POINT('Ctrl Pts',(120.400045183931,58.7281047989138,-5.05944787646731));
#7676=CARTESIAN_POINT('Ctrl Pts',(120.478340752227,59.7488216556842,-2.59582408417371));
#7677=CARTESIAN_POINT('Ctrl Pts',(120.5,60.,-1.25624131276716));
#7678=CARTESIAN_POINT('Ctrl Pts',(120.5,60.,1.25624131276716));
#7679=CARTESIAN_POINT('Ctrl Pts',(120.478340752227,59.7488216556842,2.59582408417372));
#7680=CARTESIAN_POINT('Ctrl Pts',(120.400045183931,58.7281047989138,5.05944787646731));
#7681=CARTESIAN_POINT('Ctrl Pts',(120.344523336394,57.9585982083536,6.18353741537737));
#7682=CARTESIAN_POINT('Ctrl Pts',(120.240180997842,56.183535986729,7.95859963700194));
#7683=CARTESIAN_POINT('Ctrl Pts',(120.184575491108,55.0594470790036,8.72810511950586));
#7684=CARTESIAN_POINT('Ctrl Pts',(120.10608848982,52.5958253782849,9.74882112932349));
#7685=CARTESIAN_POINT('Ctrl Pts',(120.084345357753,51.2562433349256,9.99999999999999));
#7686=CARTESIAN_POINT('Ctrl Pts',(120.084345357753,50.,9.99999999999999));
#7687=CARTESIAN_POINT('',(-120.084345357753,50.,9.99999999999999));
#7688=CARTESIAN_POINT('',(-120.084345357753,50.,-9.99999999999999));
#7689=CARTESIAN_POINT('Ctrl Pts',(-120.084345357753,50.,9.99999999999999));
#7690=CARTESIAN_POINT('Ctrl Pts',(-120.084345357753,51.2562433349256,9.99999999999999));
#7691=CARTESIAN_POINT('Ctrl Pts',(-120.10608848982,52.5958253782849,9.74882112932349));
#7692=CARTESIAN_POINT('Ctrl Pts',(-120.184575491108,55.0594470790036,8.72810511950586));
#7693=CARTESIAN_POINT('Ctrl Pts',(-120.240180997842,56.183535986729,7.95859963700195));
#7694=CARTESIAN_POINT('Ctrl Pts',(-120.344523336394,57.9585982083536,6.18353741537737));
#7695=CARTESIAN_POINT('Ctrl Pts',(-120.400045183931,58.7281047989138,5.05944787646732));
#7696=CARTESIAN_POINT('Ctrl Pts',(-120.478340752227,59.7488216556842,2.59582408417372));
#7697=CARTESIAN_POINT('Ctrl Pts',(-120.5,60.,1.25624131276716));
#7698=CARTESIAN_POINT('Ctrl Pts',(-120.5,60.,-1.25624131276716));
#7699=CARTESIAN_POINT('Ctrl Pts',(-120.478340752227,59.7488216556842,-2.59582408417371));
#7700=CARTESIAN_POINT('Ctrl Pts',(-120.400045183931,58.7281047989138,-5.05944787646731));
#7701=CARTESIAN_POINT('Ctrl Pts',(-120.344523336394,57.9585982083536,-6.18353741537737));
#7702=CARTESIAN_POINT('Ctrl Pts',(-120.240180997842,56.183535986729,-7.95859963700194));
#7703=CARTESIAN_POINT('Ctrl Pts',(-120.184575491108,55.0594470790036,-8.72810511950586));
#7704=CARTESIAN_POINT('Ctrl Pts',(-120.10608848982,52.5958253782849,-9.74882112932349));
#7705=CARTESIAN_POINT('Ctrl Pts',(-120.084345357753,51.2562433349256,-9.99999999999999));
#7706=CARTESIAN_POINT('Ctrl Pts',(-120.084345357753,50.,-9.99999999999999));
#7707=CARTESIAN_POINT('Ctrl Pts',(-120.084345357753,50.,-9.99999999999999));
#7708=CARTESIAN_POINT('Ctrl Pts',(-120.084345357753,48.7437566650744,-9.99999999999999));
#7709=CARTESIAN_POINT('Ctrl Pts',(-120.10608848982,47.4041746217151,-9.74882112932349));
#7710=CARTESIAN_POINT('Ctrl Pts',(-120.184575491108,44.9405529209964,-8.72810511950586));
#7711=CARTESIAN_POINT('Ctrl Pts',(-120.240180997842,43.816464013271,-7.95859963700195));
#7712=CARTESIAN_POINT('Ctrl Pts',(-120.344523336394,42.0414017916464,-6.18353741537737));
#7713=CARTESIAN_POINT('Ctrl Pts',(-120.400045183931,41.2718952010862,-5.0594478764673));
#7714=CARTESIAN_POINT('Ctrl Pts',(-120.478340752227,40.2511783443158,-2.59582408417371));
#7715=CARTESIAN_POINT('Ctrl Pts',(-120.5,40.,-1.25624131276716));
#7716=CARTESIAN_POINT('Ctrl Pts',(-120.5,40.,1.25624131276716));
#7717=CARTESIAN_POINT('Ctrl Pts',(-120.478340752227,40.2511783443158,2.59582408417371));
#7718=CARTESIAN_POINT('Ctrl Pts',(-120.400045183931,41.2718952010862,5.05944787646731));
#7719=CARTESIAN_POINT('Ctrl Pts',(-120.344523336394,42.0414017916464,6.18353741537737));
#7720=CARTESIAN_POINT('Ctrl Pts',(-120.240180997842,43.816464013271,7.95859963700194));
#7721=CARTESIAN_POINT('Ctrl Pts',(-120.184575491108,44.9405529209964,8.72810511950586));
#7722=CARTESIAN_POINT('Ctrl Pts',(-120.10608848982,47.4041746217151,9.74882112932349));
#7723=CARTESIAN_POINT('Ctrl Pts',(-120.084345357753,48.7437566650744,9.99999999999999));
#7724=CARTESIAN_POINT('Ctrl Pts',(-120.084345357753,50.,9.99999999999999));
#7725=CARTESIAN_POINT('Origin',(0.,105.,0.));
#7726=CARTESIAN_POINT('Ctrl Pts',(1.93800355965069E-14,48.25,105.5));
#7727=CARTESIAN_POINT('Ctrl Pts',(-43.6995308303616,48.1875,105.5));
#7728=CARTESIAN_POINT('Ctrl Pts',(-74.5997654151808,48.125,74.5997654151808));
#7729=CARTESIAN_POINT('Ctrl Pts',(-105.5,48.0625,43.6995308303616));
#7730=CARTESIAN_POINT('Ctrl Pts',(-105.5,48.,0.));
#7731=CARTESIAN_POINT('Ctrl Pts',(-105.5,47.9375,-43.6995308303615));
#7732=CARTESIAN_POINT('Ctrl Pts',(-74.5997654151808,47.875,-74.5997654151808));
#7733=CARTESIAN_POINT('Ctrl Pts',(-43.6995308303615,47.8125,-105.5));
#7734=CARTESIAN_POINT('Ctrl Pts',(-6.46001186550229E-15,47.75,-105.5));
#7735=CARTESIAN_POINT('Ctrl Pts',(43.6995308303615,47.6875,-105.5));
#7736=CARTESIAN_POINT('Ctrl Pts',(74.5997654151808,47.625,-74.5997654151808));
#7737=CARTESIAN_POINT('Ctrl Pts',(105.5,47.5625,-43.6995308303616));
#7738=CARTESIAN_POINT('Ctrl Pts',(105.5,47.5,-1.29200237310046E-14));
#7739=CARTESIAN_POINT('Ctrl Pts',(105.5,47.4375,43.6995308303615));
#7740=CARTESIAN_POINT('Ctrl Pts',(74.5997654151808,47.375,74.5997654151808));
#7741=CARTESIAN_POINT('Ctrl Pts',(43.6995308303616,47.3125,105.5));
#7742=CARTESIAN_POINT('Ctrl Pts',(1.93800355965069E-14,47.25,105.5));
#7743=CARTESIAN_POINT('Ctrl Pts',(1.93800355965069E-14,48.3750000027312,
105.5));
#7744=CARTESIAN_POINT('Ctrl Pts',(-43.6995308303616,48.3125000027312,105.5));
#7745=CARTESIAN_POINT('Ctrl Pts',(-74.5997654151808,48.2500000027312,74.5997654151808));
#7746=CARTESIAN_POINT('Ctrl Pts',(-105.5,48.1875000027312,43.6995308303616));
#7747=CARTESIAN_POINT('Ctrl Pts',(-105.5,48.1250000027312,0.));
#7748=CARTESIAN_POINT('Ctrl Pts',(-105.5,48.0625000027312,-43.6995308303615));
#7749=CARTESIAN_POINT('Ctrl Pts',(-74.5997654151808,48.0000000027312,-74.5997654151808));
#7750=CARTESIAN_POINT('Ctrl Pts',(-43.6995308303615,47.9375000027312,-105.5));
#7751=CARTESIAN_POINT('Ctrl Pts',(-6.46001186550229E-15,47.8750000027312,
-105.5));
#7752=CARTESIAN_POINT('Ctrl Pts',(43.6995308303615,47.8125000027312,-105.5));
#7753=CARTESIAN_POINT('Ctrl Pts',(74.5997654151808,47.7500000027312,-74.5997654151808));
#7754=CARTESIAN_POINT('Ctrl Pts',(105.5,47.6875000027312,-43.6995308303616));
#7755=CARTESIAN_POINT('Ctrl Pts',(105.5,47.6250000027312,-1.29200237310046E-14));
#7756=CARTESIAN_POINT('Ctrl Pts',(105.5,47.5625000027312,43.6995308303615));
#7757=CARTESIAN_POINT('Ctrl Pts',(74.5997654151808,47.5000000027312,74.5997654151808));
#7758=CARTESIAN_POINT('Ctrl Pts',(43.6995308303616,47.4375000027312,105.5));
#7759=CARTESIAN_POINT('Ctrl Pts',(1.93800355965069E-14,47.3750000027312,
105.5));
#7760=CARTESIAN_POINT('Origin',(0.,105.,0.));
#7761=CARTESIAN_POINT('',(0.,105.,118.168461709225));
#7762=CARTESIAN_POINT('Origin',(0.,105.,0.));
#7763=CARTESIAN_POINT('',(-1.41446705301519E-14,105.,-115.5));
#7764=CARTESIAN_POINT('Origin',(0.,105.,0.));
#7765=CARTESIAN_POINT('Origin',(0.,0.,0.));
#7766=CARTESIAN_POINT('',(-1.40499437705757E-14,6.66133814775094E-15,-114.726497308104));
#7767=CARTESIAN_POINT('Origin',(0.,0.,0.));
#7768=CARTESIAN_POINT('Origin',(0.,0.,0.));
#7769=CARTESIAN_POINT('Origin',(0.,100.,0.));
#7770=CARTESIAN_POINT('',(-1.4058614088468E-14,100.,-114.797295826488));
#7771=CARTESIAN_POINT('Origin',(0.,100.,0.));
#7772=CARTESIAN_POINT('Origin',(0.,105.,0.));
#7773=CARTESIAN_POINT('',(-1.44714628392369E-14,105.,118.168461709225));
#7774=CARTESIAN_POINT('Origin',(-105.2293670625,49.8437500006828,0.));
#7775=CARTESIAN_POINT('',(-104.958734125,49.6875000013656,0.));
#7776=CARTESIAN_POINT('',(-105.5,49.1250000027312,0.));
#7777=CARTESIAN_POINT('Origin',(-105.2293670625,-0.156249999317216,0.));
#7778=CARTESIAN_POINT('',(-105.5,-1.04083408558608E-14,0.));
#7779=CARTESIAN_POINT('',(-105.5,-0.874999997268824,0.));
#7780=CARTESIAN_POINT('',(-104.958734125,-0.562499998634419,0.));
#7781=CARTESIAN_POINT('',(-105.5,-0.874999997268824,0.));
#7782=CARTESIAN_POINT('Ctrl Pts',(-104.958734125,49.6875000013656,0.));
#7783=CARTESIAN_POINT('Ctrl Pts',(-104.958734125,49.6250000013656,-43.4753311640868));
#7784=CARTESIAN_POINT('Ctrl Pts',(-74.2170326445434,49.5625000013656,-74.2170326445434));
#7785=CARTESIAN_POINT('Ctrl Pts',(-43.4753311640868,49.5000000013656,-104.958734125));
#7786=CARTESIAN_POINT('Ctrl Pts',(-6.42686888943697E-15,49.4375000013656,
-104.958734125));
#7787=CARTESIAN_POINT('Ctrl Pts',(43.4753311640868,49.3750000013656,-104.958734125));
#7788=CARTESIAN_POINT('Ctrl Pts',(74.2170326445434,49.3125000013656,-74.2170326445434));
#7789=CARTESIAN_POINT('Ctrl Pts',(104.958734125,49.2500000013656,-43.4753311640868));
#7790=CARTESIAN_POINT('Ctrl Pts',(104.958734125,49.1875000013656,-1.28537377788739E-14));
#7791=CARTESIAN_POINT('Ctrl Pts',(104.958734125,49.1250000013656,43.4753311640868));
#7792=CARTESIAN_POINT('Ctrl Pts',(74.2170326445434,49.0625000013656,74.2170326445434));
#7793=CARTESIAN_POINT('Ctrl Pts',(43.4753311640869,49.0000000013656,104.958734125));
#7794=CARTESIAN_POINT('Ctrl Pts',(1.92806066683109E-14,48.9375000013656,
104.958734125));
#7795=CARTESIAN_POINT('Ctrl Pts',(-43.4753311640868,48.8750000013656,104.958734125));
#7796=CARTESIAN_POINT('Ctrl Pts',(-74.2170326445434,48.8125000013656,74.2170326445434));
#7797=CARTESIAN_POINT('Ctrl Pts',(-104.958734125,48.7500000013656,43.4753311640869));
#7798=CARTESIAN_POINT('Ctrl Pts',(-104.958734125,48.6875000013656,0.));
#7799=CARTESIAN_POINT('Ctrl Pts',(-104.958734125,48.6250000013656,-43.4753311640868));
#7800=CARTESIAN_POINT('Ctrl Pts',(-74.2170326445434,48.5625000013656,-74.2170326445434));
#7801=CARTESIAN_POINT('Ctrl Pts',(-43.4753311640868,48.5000000013656,-104.958734125));
#7802=CARTESIAN_POINT('Ctrl Pts',(-6.42686888943697E-15,48.4375000013656,
-104.958734125));
#7803=CARTESIAN_POINT('Ctrl Pts',(43.4753311640868,48.3750000013656,-104.958734125));
#7804=CARTESIAN_POINT('Ctrl Pts',(74.2170326445434,48.3125000013656,-74.2170326445434));
#7805=CARTESIAN_POINT('Ctrl Pts',(104.958734125,48.2500000013656,-43.4753311640868));
#7806=CARTESIAN_POINT('Ctrl Pts',(104.958734125,48.1875000013656,-1.28537377788739E-14));
#7807=CARTESIAN_POINT('Ctrl Pts',(104.958734125,48.1250000013656,43.4753311640868));
#7808=CARTESIAN_POINT('Ctrl Pts',(74.2170326445434,48.0625000013656,74.2170326445434));
#7809=CARTESIAN_POINT('Ctrl Pts',(43.4753311640869,48.0000000013656,104.958734125));
#7810=CARTESIAN_POINT('Ctrl Pts',(1.92806066683109E-14,47.9375000013656,
104.958734125));
#7811=CARTESIAN_POINT('Ctrl Pts',(-43.4753311640868,47.8750000013656,104.958734125));
#7812=CARTESIAN_POINT('Ctrl Pts',(-74.2170326445434,47.8125000013656,74.2170326445434));
#7813=CARTESIAN_POINT('Ctrl Pts',(-104.958734125,47.7500000013656,43.4753311640869));
#7814=CARTESIAN_POINT('Ctrl Pts',(-104.958734125,47.6875000013656,0.));
#7815=CARTESIAN_POINT('Ctrl Pts',(-104.958734125,47.6250000013656,-43.4753311640868));
#7816=CARTESIAN_POINT('Ctrl Pts',(-74.2170326445434,47.5625000013656,-74.2170326445434));
#7817=CARTESIAN_POINT('Ctrl Pts',(-43.4753311640868,47.5000000013656,-104.958734125));
#7818=CARTESIAN_POINT('Ctrl Pts',(-6.42686888943697E-15,47.4375000013656,
-104.958734125));
#7819=CARTESIAN_POINT('Ctrl Pts',(43.4753311640868,47.3750000013656,-104.958734125));
#7820=CARTESIAN_POINT('Ctrl Pts',(74.2170326445434,47.3125000013656,-74.2170326445434));
#7821=CARTESIAN_POINT('Ctrl Pts',(104.958734125,47.2500000013656,-43.4753311640868));
#7822=CARTESIAN_POINT('Ctrl Pts',(104.958734125,47.1875000013656,-1.28537377788739E-14));
#7823=CARTESIAN_POINT('Ctrl Pts',(104.958734125,47.1250000013656,43.4753311640868));
#7824=CARTESIAN_POINT('Ctrl Pts',(74.2170326445434,47.0625000013656,74.2170326445434));
#7825=CARTESIAN_POINT('Ctrl Pts',(43.4753311640869,47.0000000013656,104.958734125));
#7826=CARTESIAN_POINT('Ctrl Pts',(1.92806066683109E-14,46.9375000013656,
104.958734125));
#7827=CARTESIAN_POINT('Ctrl Pts',(-43.4753311640868,46.8750000013656,104.958734125));
#7828=CARTESIAN_POINT('Ctrl Pts',(-74.2170326445434,46.8125000013656,74.2170326445434));
#7829=CARTESIAN_POINT('Ctrl Pts',(-104.958734125,46.7500000013656,43.4753311640869));
#7830=CARTESIAN_POINT('Ctrl Pts',(-104.958734125,46.6875000013656,0.));
#7831=CARTESIAN_POINT('Ctrl Pts',(-104.958734125,46.6250000013656,-43.4753311640868));
#7832=CARTESIAN_POINT('Ctrl Pts',(-74.2170326445434,46.5625000013656,-74.2170326445434));
#7833=CARTESIAN_POINT('Ctrl Pts',(-43.4753311640868,46.5000000013656,-104.958734125));
#7834=CARTESIAN_POINT('Ctrl Pts',(-6.42686888943697E-15,46.4375000013656,
-104.958734125));
#7835=CARTESIAN_POINT('Ctrl Pts',(43.4753311640868,46.3750000013656,-104.958734125));
#7836=CARTESIAN_POINT('Ctrl Pts',(74.2170326445434,46.3125000013656,-74.2170326445434));
#7837=CARTESIAN_POINT('Ctrl Pts',(104.958734125,46.2500000013656,-43.4753311640868));
#7838=CARTESIAN_POINT('Ctrl Pts',(104.958734125,46.1875000013656,-1.28537377788739E-14));
#7839=CARTESIAN_POINT('Ctrl Pts',(104.958734125,46.1250000013656,43.4753311640868));
#7840=CARTESIAN_POINT('Ctrl Pts',(74.2170326445434,46.0625000013656,74.2170326445434));
#7841=CARTESIAN_POINT('Ctrl Pts',(43.4753311640869,46.0000000013656,104.958734125));
#7842=CARTESIAN_POINT('Ctrl Pts',(1.92806066683109E-14,45.9375000013656,
104.958734125));
#7843=CARTESIAN_POINT('Ctrl Pts',(-43.4753311640868,45.8750000013656,104.958734125));
#7844=CARTESIAN_POINT('Ctrl Pts',(-74.2170326445434,45.8125000013656,74.2170326445434));
#7845=CARTESIAN_POINT('Ctrl Pts',(-104.958734125,45.7500000013656,43.4753311640869));
#7846=CARTESIAN_POINT('Ctrl Pts',(-104.958734125,45.6875000013656,0.));
#7847=CARTESIAN_POINT('Ctrl Pts',(-104.958734125,45.6250000013656,-43.4753311640868));
#7848=CARTESIAN_POINT('Ctrl Pts',(-74.2170326445434,45.5625000013656,-74.2170326445434));
#7849=CARTESIAN_POINT('Ctrl Pts',(-43.4753311640868,45.5000000013656,-104.958734125));
#7850=CARTESIAN_POINT('Ctrl Pts',(-6.42686888943697E-15,45.4375000013656,
-104.958734125));
#7851=CARTESIAN_POINT('Ctrl Pts',(43.4753311640868,45.3750000013656,-104.958734125));
#7852=CARTESIAN_POINT('Ctrl Pts',(74.2170326445434,45.3125000013656,-74.2170326445434));
#7853=CARTESIAN_POINT('Ctrl Pts',(104.958734125,45.2500000013656,-43.4753311640868));
#7854=CARTESIAN_POINT('Ctrl Pts',(104.958734125,45.1875000013656,-1.28537377788739E-14));
#7855=CARTESIAN_POINT('Ctrl Pts',(104.958734125,45.1250000013656,43.4753311640868));
#7856=CARTESIAN_POINT('Ctrl Pts',(74.2170326445434,45.0625000013656,74.2170326445434));
#7857=CARTESIAN_POINT('Ctrl Pts',(43.4753311640869,45.0000000013656,104.958734125));
#7858=CARTESIAN_POINT('Ctrl Pts',(1.92806066683109E-14,44.9375000013656,
104.958734125));
#7859=CARTESIAN_POINT('Ctrl Pts',(-43.4753311640868,44.8750000013656,104.958734125));
#7860=CARTESIAN_POINT('Ctrl Pts',(-74.2170326445434,44.8125000013656,74.2170326445434));
#7861=CARTESIAN_POINT('Ctrl Pts',(-104.958734125,44.7500000013656,43.4753311640869));
#7862=CARTESIAN_POINT('Ctrl Pts',(-104.958734125,44.6875000013656,0.));
#7863=CARTESIAN_POINT('Ctrl Pts',(-104.958734125,44.6250000013656,-43.4753311640868));
#7864=CARTESIAN_POINT('Ctrl Pts',(-74.2170326445434,44.5625000013656,-74.2170326445434));
#7865=CARTESIAN_POINT('Ctrl Pts',(-43.4753311640868,44.5000000013656,-104.958734125));
#7866=CARTESIAN_POINT('Ctrl Pts',(-6.42686888943697E-15,44.4375000013656,
-104.958734125));
#7867=CARTESIAN_POINT('Ctrl Pts',(43.4753311640868,44.3750000013656,-104.958734125));
#7868=CARTESIAN_POINT('Ctrl Pts',(74.2170326445434,44.3125000013656,-74.2170326445434));
#7869=CARTESIAN_POINT('Ctrl Pts',(104.958734125,44.2500000013656,-43.4753311640868));
#7870=CARTESIAN_POINT('Ctrl Pts',(104.958734125,44.1875000013656,-1.28537377788739E-14));
#7871=CARTESIAN_POINT('Ctrl Pts',(104.958734125,44.1250000013656,43.4753311640868));
#7872=CARTESIAN_POINT('Ctrl Pts',(74.2170326445434,44.0625000013656,74.2170326445434));
#7873=CARTESIAN_POINT('Ctrl Pts',(43.4753311640869,44.0000000013656,104.958734125));
#7874=CARTESIAN_POINT('Ctrl Pts',(1.92806066683109E-14,43.9375000013656,
104.958734125));
#7875=CARTESIAN_POINT('Ctrl Pts',(-43.4753311640868,43.8750000013656,104.958734125));
#7876=CARTESIAN_POINT('Ctrl Pts',(-74.2170326445434,43.8125000013656,74.2170326445434));
#7877=CARTESIAN_POINT('Ctrl Pts',(-104.958734125,43.7500000013656,43.4753311640869));
#7878=CARTESIAN_POINT('Ctrl Pts',(-104.958734125,43.6875000013656,0.));
#7879=CARTESIAN_POINT('Ctrl Pts',(-104.958734125,43.6250000013656,-43.4753311640868));
#7880=CARTESIAN_POINT('Ctrl Pts',(-74.2170326445434,43.5625000013656,-74.2170326445434));
#7881=CARTESIAN_POINT('Ctrl Pts',(-43.4753311640868,43.5000000013656,-104.958734125));
#7882=CARTESIAN_POINT('Ctrl Pts',(-6.42686888943697E-15,43.4375000013656,
-104.958734125));
#7883=CARTESIAN_POINT('Ctrl Pts',(43.4753311640868,43.3750000013656,-104.958734125));
#7884=CARTESIAN_POINT('Ctrl Pts',(74.2170326445434,43.3125000013656,-74.2170326445434));
#7885=CARTESIAN_POINT('Ctrl Pts',(104.958734125,43.2500000013656,-43.4753311640868));
#7886=CARTESIAN_POINT('Ctrl Pts',(104.958734125,43.1875000013656,-1.28537377788739E-14));
#7887=CARTESIAN_POINT('Ctrl Pts',(104.958734125,43.1250000013656,43.4753311640868));
#7888=CARTESIAN_POINT('Ctrl Pts',(74.2170326445434,43.0625000013656,74.2170326445434));
#7889=CARTESIAN_POINT('Ctrl Pts',(43.4753311640869,43.0000000013656,104.958734125));
#7890=CARTESIAN_POINT('Ctrl Pts',(1.92806066683109E-14,42.9375000013656,
104.958734125));
#7891=CARTESIAN_POINT('Ctrl Pts',(-43.4753311640868,42.8750000013656,104.958734125));
#7892=CARTESIAN_POINT('Ctrl Pts',(-74.2170326445434,42.8125000013656,74.2170326445434));
#7893=CARTESIAN_POINT('Ctrl Pts',(-104.958734125,42.7500000013656,43.4753311640869));
#7894=CARTESIAN_POINT('Ctrl Pts',(-104.958734125,42.6875000013656,0.));
#7895=CARTESIAN_POINT('Ctrl Pts',(-104.958734125,42.6250000013656,-43.4753311640868));
#7896=CARTESIAN_POINT('Ctrl Pts',(-74.2170326445434,42.5625000013656,-74.2170326445434));
#7897=CARTESIAN_POINT('Ctrl Pts',(-43.4753311640868,42.5000000013656,-104.958734125));
#7898=CARTESIAN_POINT('Ctrl Pts',(-6.42686888943697E-15,42.4375000013656,
-104.958734125));
#7899=CARTESIAN_POINT('Ctrl Pts',(43.4753311640868,42.3750000013656,-104.958734125));
#7900=CARTESIAN_POINT('Ctrl Pts',(74.2170326445434,42.3125000013656,-74.2170326445434));
#7901=CARTESIAN_POINT('Ctrl Pts',(104.958734125,42.2500000013656,-43.4753311640868));
#7902=CARTESIAN_POINT('Ctrl Pts',(104.958734125,42.1875000013656,-1.28537377788739E-14));
#7903=CARTESIAN_POINT('Ctrl Pts',(104.958734125,42.1250000013656,43.4753311640868));
#7904=CARTESIAN_POINT('Ctrl Pts',(74.2170326445434,42.0625000013656,74.2170326445434));
#7905=CARTESIAN_POINT('Ctrl Pts',(43.4753311640869,42.0000000013656,104.958734125));
#7906=CARTESIAN_POINT('Ctrl Pts',(1.92806066683109E-14,41.9375000013656,
104.958734125));
#7907=CARTESIAN_POINT('Ctrl Pts',(-43.4753311640868,41.8750000013656,104.958734125));
#7908=CARTESIAN_POINT('Ctrl Pts',(-74.2170326445434,41.8125000013656,74.2170326445434));
#7909=CARTESIAN_POINT('Ctrl Pts',(-104.958734125,41.7500000013656,43.4753311640869));
#7910=CARTESIAN_POINT('Ctrl Pts',(-104.958734125,41.6875000013656,0.));
#7911=CARTESIAN_POINT('Ctrl Pts',(-104.958734125,41.6250000013656,-43.4753311640868));
#7912=CARTESIAN_POINT('Ctrl Pts',(-74.2170326445434,41.5625000013656,-74.2170326445434));
#7913=CARTESIAN_POINT('Ctrl Pts',(-43.4753311640868,41.5000000013656,-104.958734125));
#7914=CARTESIAN_POINT('Ctrl Pts',(-6.42686888943697E-15,41.4375000013656,
-104.958734125));
#7915=CARTESIAN_POINT('Ctrl Pts',(43.4753311640868,41.3750000013656,-104.958734125));
#7916=CARTESIAN_POINT('Ctrl Pts',(74.2170326445434,41.3125000013656,-74.2170326445434));
#7917=CARTESIAN_POINT('Ctrl Pts',(104.958734125,41.2500000013656,-43.4753311640868));
#7918=CARTESIAN_POINT('Ctrl Pts',(104.958734125,41.1875000013656,-1.28537377788739E-14));
#7919=CARTESIAN_POINT('Ctrl Pts',(104.958734125,41.1250000013656,43.4753311640868));
#7920=CARTESIAN_POINT('Ctrl Pts',(74.2170326445434,41.0625000013656,74.2170326445434));
#7921=CARTESIAN_POINT('Ctrl Pts',(43.4753311640869,41.0000000013656,104.958734125));
#7922=CARTESIAN_POINT('Ctrl Pts',(1.92806066683109E-14,40.9375000013656,
104.958734125));
#7923=CARTESIAN_POINT('Ctrl Pts',(-43.4753311640868,40.8750000013656,104.958734125));
#7924=CARTESIAN_POINT('Ctrl Pts',(-74.2170326445434,40.8125000013656,74.2170326445434));
#7925=CARTESIAN_POINT('Ctrl Pts',(-104.958734125,40.7500000013656,43.4753311640869));
#7926=CARTESIAN_POINT('Ctrl Pts',(-104.958734125,40.6875000013656,0.));
#7927=CARTESIAN_POINT('Ctrl Pts',(-104.958734125,40.6250000013656,-43.4753311640868));
#7928=CARTESIAN_POINT('Ctrl Pts',(-74.2170326445434,40.5625000013656,-74.2170326445434));
#7929=CARTESIAN_POINT('Ctrl Pts',(-43.4753311640868,40.5000000013656,-104.958734125));
#7930=CARTESIAN_POINT('Ctrl Pts',(-6.42686888943697E-15,40.4375000013656,
-104.958734125));
#7931=CARTESIAN_POINT('Ctrl Pts',(43.4753311640868,40.3750000013656,-104.958734125));
#7932=CARTESIAN_POINT('Ctrl Pts',(74.2170326445434,40.3125000013656,-74.2170326445434));
#7933=CARTESIAN_POINT('Ctrl Pts',(104.958734125,40.2500000013656,-43.4753311640868));
#7934=CARTESIAN_POINT('Ctrl Pts',(104.958734125,40.1875000013656,-1.28537377788739E-14));
#7935=CARTESIAN_POINT('Ctrl Pts',(104.958734125,40.1250000013656,43.4753311640868));
#7936=CARTESIAN_POINT('Ctrl Pts',(74.2170326445434,40.0625000013656,74.2170326445434));
#7937=CARTESIAN_POINT('Ctrl Pts',(43.4753311640869,40.0000000013656,104.958734125));
#7938=CARTESIAN_POINT('Ctrl Pts',(1.92806066683109E-14,39.9375000013656,
104.958734125));
#7939=CARTESIAN_POINT('Ctrl Pts',(-43.4753311640868,39.8750000013656,104.958734125));
#7940=CARTESIAN_POINT('Ctrl Pts',(-74.2170326445434,39.8125000013656,74.2170326445434));
#7941=CARTESIAN_POINT('Ctrl Pts',(-104.958734125,39.7500000013656,43.4753311640869));
#7942=CARTESIAN_POINT('Ctrl Pts',(-104.958734125,39.6875000013656,0.));
#7943=CARTESIAN_POINT('Ctrl Pts',(-104.958734125,39.6250000013656,-43.4753311640868));
#7944=CARTESIAN_POINT('Ctrl Pts',(-74.2170326445434,39.5625000013656,-74.2170326445434));
#7945=CARTESIAN_POINT('Ctrl Pts',(-43.4753311640868,39.5000000013656,-104.958734125));
#7946=CARTESIAN_POINT('Ctrl Pts',(-6.42686888943697E-15,39.4375000013656,
-104.958734125));
#7947=CARTESIAN_POINT('Ctrl Pts',(43.4753311640868,39.3750000013656,-104.958734125));
#7948=CARTESIAN_POINT('Ctrl Pts',(74.2170326445434,39.3125000013656,-74.2170326445434));
#7949=CARTESIAN_POINT('Ctrl Pts',(104.958734125,39.2500000013656,-43.4753311640868));
#7950=CARTESIAN_POINT('Ctrl Pts',(104.958734125,39.1875000013656,-1.28537377788739E-14));
#7951=CARTESIAN_POINT('Ctrl Pts',(104.958734125,39.1250000013656,43.4753311640868));
#7952=CARTESIAN_POINT('Ctrl Pts',(74.2170326445434,39.0625000013656,74.2170326445434));
#7953=CARTESIAN_POINT('Ctrl Pts',(43.4753311640869,39.0000000013656,104.958734125));
#7954=CARTESIAN_POINT('Ctrl Pts',(1.92806066683109E-14,38.9375000013656,
104.958734125));
#7955=CARTESIAN_POINT('Ctrl Pts',(-43.4753311640868,38.8750000013656,104.958734125));
#7956=CARTESIAN_POINT('Ctrl Pts',(-74.2170326445434,38.8125000013656,74.2170326445434));
#7957=CARTESIAN_POINT('Ctrl Pts',(-104.958734125,38.7500000013656,43.4753311640869));
#7958=CARTESIAN_POINT('Ctrl Pts',(-104.958734125,38.6875000013656,0.));
#7959=CARTESIAN_POINT('Ctrl Pts',(-104.958734125,38.6250000013656,-43.4753311640868));
#7960=CARTESIAN_POINT('Ctrl Pts',(-74.2170326445434,38.5625000013656,-74.2170326445434));
#7961=CARTESIAN_POINT('Ctrl Pts',(-43.4753311640868,38.5000000013656,-104.958734125));
#7962=CARTESIAN_POINT('Ctrl Pts',(-6.42686888943697E-15,38.4375000013656,
-104.958734125));
#7963=CARTESIAN_POINT('Ctrl Pts',(43.4753311640868,38.3750000013656,-104.958734125));
#7964=CARTESIAN_POINT('Ctrl Pts',(74.2170326445434,38.3125000013656,-74.2170326445434));
#7965=CARTESIAN_POINT('Ctrl Pts',(104.958734125,38.2500000013656,-43.4753311640868));
#7966=CARTESIAN_POINT('Ctrl Pts',(104.958734125,38.1875000013656,-1.28537377788739E-14));
#7967=CARTESIAN_POINT('Ctrl Pts',(104.958734125,38.1250000013656,43.4753311640868));
#7968=CARTESIAN_POINT('Ctrl Pts',(74.2170326445434,38.0625000013656,74.2170326445434));
#7969=CARTESIAN_POINT('Ctrl Pts',(43.4753311640869,38.0000000013656,104.958734125));
#7970=CARTESIAN_POINT('Ctrl Pts',(1.92806066683109E-14,37.9375000013656,
104.958734125));
#7971=CARTESIAN_POINT('Ctrl Pts',(-43.4753311640868,37.8750000013656,104.958734125));
#7972=CARTESIAN_POINT('Ctrl Pts',(-74.2170326445434,37.8125000013656,74.2170326445434));
#7973=CARTESIAN_POINT('Ctrl Pts',(-104.958734125,37.7500000013656,43.4753311640869));
#7974=CARTESIAN_POINT('Ctrl Pts',(-104.958734125,37.6875000013656,0.));
#7975=CARTESIAN_POINT('Ctrl Pts',(-104.958734125,37.6250000013656,-43.4753311640868));
#7976=CARTESIAN_POINT('Ctrl Pts',(-74.2170326445434,37.5625000013656,-74.2170326445434));
#7977=CARTESIAN_POINT('Ctrl Pts',(-43.4753311640868,37.5000000013656,-104.958734125));
#7978=CARTESIAN_POINT('Ctrl Pts',(-6.42686888943697E-15,37.4375000013656,
-104.958734125));
#7979=CARTESIAN_POINT('Ctrl Pts',(43.4753311640868,37.3750000013656,-104.958734125));
#7980=CARTESIAN_POINT('Ctrl Pts',(74.2170326445434,37.3125000013656,-74.2170326445434));
#7981=CARTESIAN_POINT('Ctrl Pts',(104.958734125,37.2500000013656,-43.4753311640868));
#7982=CARTESIAN_POINT('Ctrl Pts',(104.958734125,37.1875000013656,-1.28537377788739E-14));
#7983=CARTESIAN_POINT('Ctrl Pts',(104.958734125,37.1250000013656,43.4753311640868));
#7984=CARTESIAN_POINT('Ctrl Pts',(74.2170326445434,37.0625000013656,74.2170326445434));
#7985=CARTESIAN_POINT('Ctrl Pts',(43.4753311640869,37.0000000013656,104.958734125));
#7986=CARTESIAN_POINT('Ctrl Pts',(1.92806066683109E-14,36.9375000013656,
104.958734125));
#7987=CARTESIAN_POINT('Ctrl Pts',(-43.4753311640868,36.8750000013656,104.958734125));
#7988=CARTESIAN_POINT('Ctrl Pts',(-74.2170326445434,36.8125000013656,74.2170326445434));
#7989=CARTESIAN_POINT('Ctrl Pts',(-104.958734125,36.7500000013656,43.4753311640869));
#7990=CARTESIAN_POINT('Ctrl Pts',(-104.958734125,36.6875000013656,0.));
#7991=CARTESIAN_POINT('Ctrl Pts',(-104.958734125,36.6250000013656,-43.4753311640868));
#7992=CARTESIAN_POINT('Ctrl Pts',(-74.2170326445434,36.5625000013656,-74.2170326445434));
#7993=CARTESIAN_POINT('Ctrl Pts',(-43.4753311640868,36.5000000013656,-104.958734125));
#7994=CARTESIAN_POINT('Ctrl Pts',(-6.42686888943697E-15,36.4375000013656,
-104.958734125));
#7995=CARTESIAN_POINT('Ctrl Pts',(43.4753311640868,36.3750000013656,-104.958734125));
#7996=CARTESIAN_POINT('Ctrl Pts',(74.2170326445434,36.3125000013656,-74.2170326445434));
#7997=CARTESIAN_POINT('Ctrl Pts',(104.958734125,36.2500000013656,-43.4753311640868));
#7998=CARTESIAN_POINT('Ctrl Pts',(104.958734125,36.1875000013656,-1.28537377788739E-14));
#7999=CARTESIAN_POINT('Ctrl Pts',(104.958734125,36.1250000013656,43.4753311640868));
#8000=CARTESIAN_POINT('Ctrl Pts',(74.2170326445434,36.0625000013656,74.2170326445434));
#8001=CARTESIAN_POINT('Ctrl Pts',(43.4753311640869,36.0000000013656,104.958734125));
#8002=CARTESIAN_POINT('Ctrl Pts',(1.92806066683109E-14,35.9375000013656,
104.958734125));
#8003=CARTESIAN_POINT('Ctrl Pts',(-43.4753311640868,35.8750000013656,104.958734125));
#8004=CARTESIAN_POINT('Ctrl Pts',(-74.2170326445434,35.8125000013656,74.2170326445434));
#8005=CARTESIAN_POINT('Ctrl Pts',(-104.958734125,35.7500000013656,43.4753311640869));
#8006=CARTESIAN_POINT('Ctrl Pts',(-104.958734125,35.6875000013656,0.));
#8007=CARTESIAN_POINT('Ctrl Pts',(-104.958734125,35.6250000013656,-43.4753311640868));
#8008=CARTESIAN_POINT('Ctrl Pts',(-74.2170326445434,35.5625000013656,-74.2170326445434));
#8009=CARTESIAN_POINT('Ctrl Pts',(-43.4753311640868,35.5000000013656,-104.958734125));
#8010=CARTESIAN_POINT('Ctrl Pts',(-6.42686888943697E-15,35.4375000013656,
-104.958734125));
#8011=CARTESIAN_POINT('Ctrl Pts',(43.4753311640868,35.3750000013656,-104.958734125));
#8012=CARTESIAN_POINT('Ctrl Pts',(74.2170326445434,35.3125000013656,-74.2170326445434));
#8013=CARTESIAN_POINT('Ctrl Pts',(104.958734125,35.2500000013656,-43.4753311640868));
#8014=CARTESIAN_POINT('Ctrl Pts',(104.958734125,35.1875000013656,-1.28537377788739E-14));
#8015=CARTESIAN_POINT('Ctrl Pts',(104.958734125,35.1250000013656,43.4753311640868));
#8016=CARTESIAN_POINT('Ctrl Pts',(74.2170326445434,35.0625000013656,74.2170326445434));
#8017=CARTESIAN_POINT('Ctrl Pts',(43.4753311640869,35.0000000013656,104.958734125));
#8018=CARTESIAN_POINT('Ctrl Pts',(1.92806066683109E-14,34.9375000013656,
104.958734125));
#8019=CARTESIAN_POINT('Ctrl Pts',(-43.4753311640868,34.8750000013656,104.958734125));
#8020=CARTESIAN_POINT('Ctrl Pts',(-74.2170326445434,34.8125000013656,74.2170326445434));
#8021=CARTESIAN_POINT('Ctrl Pts',(-104.958734125,34.7500000013656,43.4753311640869));
#8022=CARTESIAN_POINT('Ctrl Pts',(-104.958734125,34.6875000013656,0.));
#8023=CARTESIAN_POINT('Ctrl Pts',(-104.958734125,34.6250000013656,-43.4753311640868));
#8024=CARTESIAN_POINT('Ctrl Pts',(-74.2170326445434,34.5625000013656,-74.2170326445434));
#8025=CARTESIAN_POINT('Ctrl Pts',(-43.4753311640868,34.5000000013656,-104.958734125));
#8026=CARTESIAN_POINT('Ctrl Pts',(-6.42686888943697E-15,34.4375000013656,
-104.958734125));
#8027=CARTESIAN_POINT('Ctrl Pts',(43.4753311640868,34.3750000013656,-104.958734125));
#8028=CARTESIAN_POINT('Ctrl Pts',(74.2170326445434,34.3125000013656,-74.2170326445434));
#8029=CARTESIAN_POINT('Ctrl Pts',(104.958734125,34.2500000013656,-43.4753311640868));
#8030=CARTESIAN_POINT('Ctrl Pts',(104.958734125,34.1875000013656,-1.28537377788739E-14));
#8031=CARTESIAN_POINT('Ctrl Pts',(104.958734125,34.1250000013656,43.4753311640868));
#8032=CARTESIAN_POINT('Ctrl Pts',(74.2170326445434,34.0625000013656,74.2170326445434));
#8033=CARTESIAN_POINT('Ctrl Pts',(43.4753311640869,34.0000000013656,104.958734125));
#8034=CARTESIAN_POINT('Ctrl Pts',(1.92806066683109E-14,33.9375000013656,
104.958734125));
#8035=CARTESIAN_POINT('Ctrl Pts',(-43.4753311640868,33.8750000013656,104.958734125));
#8036=CARTESIAN_POINT('Ctrl Pts',(-74.2170326445434,33.8125000013656,74.2170326445434));
#8037=CARTESIAN_POINT('Ctrl Pts',(-104.958734125,33.7500000013656,43.4753311640869));
#8038=CARTESIAN_POINT('Ctrl Pts',(-104.958734125,33.6875000013656,0.));
#8039=CARTESIAN_POINT('Ctrl Pts',(-104.958734125,33.6250000013656,-43.4753311640868));
#8040=CARTESIAN_POINT('Ctrl Pts',(-74.2170326445434,33.5625000013656,-74.2170326445434));
#8041=CARTESIAN_POINT('Ctrl Pts',(-43.4753311640868,33.5000000013656,-104.958734125));
#8042=CARTESIAN_POINT('Ctrl Pts',(-6.42686888943697E-15,33.4375000013656,
-104.958734125));
#8043=CARTESIAN_POINT('Ctrl Pts',(43.4753311640868,33.3750000013656,-104.958734125));
#8044=CARTESIAN_POINT('Ctrl Pts',(74.2170326445434,33.3125000013656,-74.2170326445434));
#8045=CARTESIAN_POINT('Ctrl Pts',(104.958734125,33.2500000013656,-43.4753311640868));
#8046=CARTESIAN_POINT('Ctrl Pts',(104.958734125,33.1875000013656,-1.28537377788739E-14));
#8047=CARTESIAN_POINT('Ctrl Pts',(104.958734125,33.1250000013656,43.4753311640868));
#8048=CARTESIAN_POINT('Ctrl Pts',(74.2170326445434,33.0625000013656,74.2170326445434));
#8049=CARTESIAN_POINT('Ctrl Pts',(43.4753311640869,33.0000000013656,104.958734125));
#8050=CARTESIAN_POINT('Ctrl Pts',(1.92806066683109E-14,32.9375000013656,
104.958734125));
#8051=CARTESIAN_POINT('Ctrl Pts',(-43.4753311640868,32.8750000013656,104.958734125));
#8052=CARTESIAN_POINT('Ctrl Pts',(-74.2170326445434,32.8125000013656,74.2170326445434));
#8053=CARTESIAN_POINT('Ctrl Pts',(-104.958734125,32.7500000013656,43.4753311640869));
#8054=CARTESIAN_POINT('Ctrl Pts',(-104.958734125,32.6875000013656,0.));
#8055=CARTESIAN_POINT('Ctrl Pts',(-104.958734125,32.6250000013656,-43.4753311640868));
#8056=CARTESIAN_POINT('Ctrl Pts',(-74.2170326445434,32.5625000013656,-74.2170326445434));
#8057=CARTESIAN_POINT('Ctrl Pts',(-43.4753311640868,32.5000000013656,-104.958734125));
#8058=CARTESIAN_POINT('Ctrl Pts',(-6.42686888943697E-15,32.4375000013656,
-104.958734125));
#8059=CARTESIAN_POINT('Ctrl Pts',(43.4753311640868,32.3750000013656,-104.958734125));
#8060=CARTESIAN_POINT('Ctrl Pts',(74.2170326445434,32.3125000013656,-74.2170326445434));
#8061=CARTESIAN_POINT('Ctrl Pts',(104.958734125,32.2500000013656,-43.4753311640868));
#8062=CARTESIAN_POINT('Ctrl Pts',(104.958734125,32.1875000013656,-1.28537377788739E-14));
#8063=CARTESIAN_POINT('Ctrl Pts',(104.958734125,32.1250000013656,43.4753311640868));
#8064=CARTESIAN_POINT('Ctrl Pts',(74.2170326445434,32.0625000013656,74.2170326445434));
#8065=CARTESIAN_POINT('Ctrl Pts',(43.4753311640869,32.0000000013656,104.958734125));
#8066=CARTESIAN_POINT('Ctrl Pts',(1.92806066683109E-14,31.9375000013656,
104.958734125));
#8067=CARTESIAN_POINT('Ctrl Pts',(-43.4753311640868,31.8750000013656,104.958734125));
#8068=CARTESIAN_POINT('Ctrl Pts',(-74.2170326445434,31.8125000013656,74.2170326445434));
#8069=CARTESIAN_POINT('Ctrl Pts',(-104.958734125,31.7500000013656,43.4753311640869));
#8070=CARTESIAN_POINT('Ctrl Pts',(-104.958734125,31.6875000013656,0.));
#8071=CARTESIAN_POINT('Ctrl Pts',(-104.958734125,31.6250000013656,-43.4753311640868));
#8072=CARTESIAN_POINT('Ctrl Pts',(-74.2170326445434,31.5625000013656,-74.2170326445434));
#8073=CARTESIAN_POINT('Ctrl Pts',(-43.4753311640868,31.5000000013656,-104.958734125));
#8074=CARTESIAN_POINT('Ctrl Pts',(-6.42686888943697E-15,31.4375000013656,
-104.958734125));
#8075=CARTESIAN_POINT('Ctrl Pts',(43.4753311640868,31.3750000013656,-104.958734125));
#8076=CARTESIAN_POINT('Ctrl Pts',(74.2170326445434,31.3125000013656,-74.2170326445434));
#8077=CARTESIAN_POINT('Ctrl Pts',(104.958734125,31.2500000013656,-43.4753311640868));
#8078=CARTESIAN_POINT('Ctrl Pts',(104.958734125,31.1875000013656,-1.28537377788739E-14));
#8079=CARTESIAN_POINT('Ctrl Pts',(104.958734125,31.1250000013656,43.4753311640868));
#8080=CARTESIAN_POINT('Ctrl Pts',(74.2170326445434,31.0625000013656,74.2170326445434));
#8081=CARTESIAN_POINT('Ctrl Pts',(43.4753311640869,31.0000000013656,104.958734125));
#8082=CARTESIAN_POINT('Ctrl Pts',(1.92806066683109E-14,30.9375000013656,
104.958734125));
#8083=CARTESIAN_POINT('Ctrl Pts',(-43.4753311640868,30.8750000013656,104.958734125));
#8084=CARTESIAN_POINT('Ctrl Pts',(-74.2170326445434,30.8125000013656,74.2170326445434));
#8085=CARTESIAN_POINT('Ctrl Pts',(-104.958734125,30.7500000013656,43.4753311640869));
#8086=CARTESIAN_POINT('Ctrl Pts',(-104.958734125,30.6875000013656,0.));
#8087=CARTESIAN_POINT('Ctrl Pts',(-104.958734125,30.6250000013656,-43.4753311640868));
#8088=CARTESIAN_POINT('Ctrl Pts',(-74.2170326445434,30.5625000013656,-74.2170326445434));
#8089=CARTESIAN_POINT('Ctrl Pts',(-43.4753311640868,30.5000000013656,-104.958734125));
#8090=CARTESIAN_POINT('Ctrl Pts',(-6.42686888943697E-15,30.4375000013656,
-104.958734125));
#8091=CARTESIAN_POINT('Ctrl Pts',(43.4753311640868,30.3750000013656,-104.958734125));
#8092=CARTESIAN_POINT('Ctrl Pts',(74.2170326445434,30.3125000013656,-74.2170326445434));
#8093=CARTESIAN_POINT('Ctrl Pts',(104.958734125,30.2500000013656,-43.4753311640868));
#8094=CARTESIAN_POINT('Ctrl Pts',(104.958734125,30.1875000013656,-1.28537377788739E-14));
#8095=CARTESIAN_POINT('Ctrl Pts',(104.958734125,30.1250000013656,43.4753311640868));
#8096=CARTESIAN_POINT('Ctrl Pts',(74.2170326445434,30.0625000013656,74.2170326445434));
#8097=CARTESIAN_POINT('Ctrl Pts',(43.4753311640869,30.0000000013656,104.958734125));
#8098=CARTESIAN_POINT('Ctrl Pts',(1.92806066683109E-14,29.9375000013656,
104.958734125));
#8099=CARTESIAN_POINT('Ctrl Pts',(-43.4753311640868,29.8750000013656,104.958734125));
#8100=CARTESIAN_POINT('Ctrl Pts',(-74.2170326445434,29.8125000013656,74.2170326445434));
#8101=CARTESIAN_POINT('Ctrl Pts',(-104.958734125,29.7500000013656,43.4753311640869));
#8102=CARTESIAN_POINT('Ctrl Pts',(-104.958734125,29.6875000013656,0.));
#8103=CARTESIAN_POINT('Ctrl Pts',(-104.958734125,29.6250000013656,-43.4753311640868));
#8104=CARTESIAN_POINT('Ctrl Pts',(-74.2170326445434,29.5625000013656,-74.2170326445434));
#8105=CARTESIAN_POINT('Ctrl Pts',(-43.4753311640868,29.5000000013656,-104.958734125));
#8106=CARTESIAN_POINT('Ctrl Pts',(-6.42686888943697E-15,29.4375000013656,
-104.958734125));
#8107=CARTESIAN_POINT('Ctrl Pts',(43.4753311640868,29.3750000013656,-104.958734125));
#8108=CARTESIAN_POINT('Ctrl Pts',(74.2170326445434,29.3125000013656,-74.2170326445434));
#8109=CARTESIAN_POINT('Ctrl Pts',(104.958734125,29.2500000013656,-43.4753311640868));
#8110=CARTESIAN_POINT('Ctrl Pts',(104.958734125,29.1875000013656,-1.28537377788739E-14));
#8111=CARTESIAN_POINT('Ctrl Pts',(104.958734125,29.1250000013656,43.4753311640868));
#8112=CARTESIAN_POINT('Ctrl Pts',(74.2170326445434,29.0625000013656,74.2170326445434));
#8113=CARTESIAN_POINT('Ctrl Pts',(43.4753311640869,29.0000000013656,104.958734125));
#8114=CARTESIAN_POINT('Ctrl Pts',(1.92806066683109E-14,28.9375000013656,
104.958734125));
#8115=CARTESIAN_POINT('Ctrl Pts',(-43.4753311640868,28.8750000013656,104.958734125));
#8116=CARTESIAN_POINT('Ctrl Pts',(-74.2170326445434,28.8125000013656,74.2170326445434));
#8117=CARTESIAN_POINT('Ctrl Pts',(-104.958734125,28.7500000013656,43.4753311640869));
#8118=CARTESIAN_POINT('Ctrl Pts',(-104.958734125,28.6875000013656,0.));
#8119=CARTESIAN_POINT('Ctrl Pts',(-104.958734125,28.6250000013656,-43.4753311640868));
#8120=CARTESIAN_POINT('Ctrl Pts',(-74.2170326445434,28.5625000013656,-74.2170326445434));
#8121=CARTESIAN_POINT('Ctrl Pts',(-43.4753311640868,28.5000000013656,-104.958734125));
#8122=CARTESIAN_POINT('Ctrl Pts',(-6.42686888943697E-15,28.4375000013656,
-104.958734125));
#8123=CARTESIAN_POINT('Ctrl Pts',(43.4753311640868,28.3750000013656,-104.958734125));
#8124=CARTESIAN_POINT('Ctrl Pts',(74.2170326445434,28.3125000013656,-74.2170326445434));
#8125=CARTESIAN_POINT('Ctrl Pts',(104.958734125,28.2500000013656,-43.4753311640868));
#8126=CARTESIAN_POINT('Ctrl Pts',(104.958734125,28.1875000013656,-1.28537377788739E-14));
#8127=CARTESIAN_POINT('Ctrl Pts',(104.958734125,28.1250000013656,43.4753311640868));
#8128=CARTESIAN_POINT('Ctrl Pts',(74.2170326445434,28.0625000013656,74.2170326445434));
#8129=CARTESIAN_POINT('Ctrl Pts',(43.4753311640869,28.0000000013656,104.958734125));
#8130=CARTESIAN_POINT('Ctrl Pts',(1.92806066683109E-14,27.9375000013656,
104.958734125));
#8131=CARTESIAN_POINT('Ctrl Pts',(-43.4753311640868,27.8750000013656,104.958734125));
#8132=CARTESIAN_POINT('Ctrl Pts',(-74.2170326445434,27.8125000013656,74.2170326445434));
#8133=CARTESIAN_POINT('Ctrl Pts',(-104.958734125,27.7500000013656,43.4753311640869));
#8134=CARTESIAN_POINT('Ctrl Pts',(-104.958734125,27.6875000013656,0.));
#8135=CARTESIAN_POINT('Ctrl Pts',(-104.958734125,27.6250000013656,-43.4753311640868));
#8136=CARTESIAN_POINT('Ctrl Pts',(-74.2170326445434,27.5625000013656,-74.2170326445434));
#8137=CARTESIAN_POINT('Ctrl Pts',(-43.4753311640868,27.5000000013656,-104.958734125));
#8138=CARTESIAN_POINT('Ctrl Pts',(-6.42686888943697E-15,27.4375000013656,
-104.958734125));
#8139=CARTESIAN_POINT('Ctrl Pts',(43.4753311640868,27.3750000013656,-104.958734125));
#8140=CARTESIAN_POINT('Ctrl Pts',(74.2170326445434,27.3125000013656,-74.2170326445434));
#8141=CARTESIAN_POINT('Ctrl Pts',(104.958734125,27.2500000013656,-43.4753311640868));
#8142=CARTESIAN_POINT('Ctrl Pts',(104.958734125,27.1875000013656,-1.28537377788739E-14));
#8143=CARTESIAN_POINT('Ctrl Pts',(104.958734125,27.1250000013656,43.4753311640868));
#8144=CARTESIAN_POINT('Ctrl Pts',(74.2170326445434,27.0625000013656,74.2170326445434));
#8145=CARTESIAN_POINT('Ctrl Pts',(43.4753311640869,27.0000000013656,104.958734125));
#8146=CARTESIAN_POINT('Ctrl Pts',(1.92806066683109E-14,26.9375000013656,
104.958734125));
#8147=CARTESIAN_POINT('Ctrl Pts',(-43.4753311640868,26.8750000013656,104.958734125));
#8148=CARTESIAN_POINT('Ctrl Pts',(-74.2170326445434,26.8125000013656,74.2170326445434));
#8149=CARTESIAN_POINT('Ctrl Pts',(-104.958734125,26.7500000013656,43.4753311640869));
#8150=CARTESIAN_POINT('Ctrl Pts',(-104.958734125,26.6875000013656,0.));
#8151=CARTESIAN_POINT('Ctrl Pts',(-104.958734125,26.6250000013656,-43.4753311640868));
#8152=CARTESIAN_POINT('Ctrl Pts',(-74.2170326445434,26.5625000013656,-74.2170326445434));
#8153=CARTESIAN_POINT('Ctrl Pts',(-43.4753311640868,26.5000000013656,-104.958734125));
#8154=CARTESIAN_POINT('Ctrl Pts',(-6.42686888943697E-15,26.4375000013656,
-104.958734125));
#8155=CARTESIAN_POINT('Ctrl Pts',(43.4753311640868,26.3750000013656,-104.958734125));
#8156=CARTESIAN_POINT('Ctrl Pts',(74.2170326445434,26.3125000013656,-74.2170326445434));
#8157=CARTESIAN_POINT('Ctrl Pts',(104.958734125,26.2500000013656,-43.4753311640868));
#8158=CARTESIAN_POINT('Ctrl Pts',(104.958734125,26.1875000013656,-1.28537377788739E-14));
#8159=CARTESIAN_POINT('Ctrl Pts',(104.958734125,26.1250000013656,43.4753311640868));
#8160=CARTESIAN_POINT('Ctrl Pts',(74.2170326445434,26.0625000013656,74.2170326445434));
#8161=CARTESIAN_POINT('Ctrl Pts',(43.4753311640869,26.0000000013656,104.958734125));
#8162=CARTESIAN_POINT('Ctrl Pts',(1.92806066683109E-14,25.9375000013656,
104.958734125));
#8163=CARTESIAN_POINT('Ctrl Pts',(-43.4753311640868,25.8750000013656,104.958734125));
#8164=CARTESIAN_POINT('Ctrl Pts',(-74.2170326445434,25.8125000013656,74.2170326445434));
#8165=CARTESIAN_POINT('Ctrl Pts',(-104.958734125,25.7500000013656,43.4753311640869));
#8166=CARTESIAN_POINT('Ctrl Pts',(-104.958734125,25.6875000013656,0.));
#8167=CARTESIAN_POINT('Ctrl Pts',(-104.958734125,25.6250000013656,-43.4753311640868));
#8168=CARTESIAN_POINT('Ctrl Pts',(-74.2170326445434,25.5625000013656,-74.2170326445434));
#8169=CARTESIAN_POINT('Ctrl Pts',(-43.4753311640868,25.5000000013656,-104.958734125));
#8170=CARTESIAN_POINT('Ctrl Pts',(-6.42686888943697E-15,25.4375000013656,
-104.958734125));
#8171=CARTESIAN_POINT('Ctrl Pts',(43.4753311640868,25.3750000013656,-104.958734125));
#8172=CARTESIAN_POINT('Ctrl Pts',(74.2170326445434,25.3125000013656,-74.2170326445434));
#8173=CARTESIAN_POINT('Ctrl Pts',(104.958734125,25.2500000013656,-43.4753311640868));
#8174=CARTESIAN_POINT('Ctrl Pts',(104.958734125,25.1875000013656,-1.28537377788739E-14));
#8175=CARTESIAN_POINT('Ctrl Pts',(104.958734125,25.1250000013656,43.4753311640868));
#8176=CARTESIAN_POINT('Ctrl Pts',(74.2170326445434,25.0625000013656,74.2170326445434));
#8177=CARTESIAN_POINT('Ctrl Pts',(43.4753311640869,25.0000000013656,104.958734125));
#8178=CARTESIAN_POINT('Ctrl Pts',(1.92806066683109E-14,24.9375000013656,
104.958734125));
#8179=CARTESIAN_POINT('Ctrl Pts',(-43.4753311640868,24.8750000013656,104.958734125));
#8180=CARTESIAN_POINT('Ctrl Pts',(-74.2170326445434,24.8125000013656,74.2170326445434));
#8181=CARTESIAN_POINT('Ctrl Pts',(-104.958734125,24.7500000013656,43.4753311640869));
#8182=CARTESIAN_POINT('Ctrl Pts',(-104.958734125,24.6875000013656,0.));
#8183=CARTESIAN_POINT('Ctrl Pts',(-104.958734125,24.6250000013656,-43.4753311640868));
#8184=CARTESIAN_POINT('Ctrl Pts',(-74.2170326445434,24.5625000013656,-74.2170326445434));
#8185=CARTESIAN_POINT('Ctrl Pts',(-43.4753311640868,24.5000000013656,-104.958734125));
#8186=CARTESIAN_POINT('Ctrl Pts',(-6.42686888943697E-15,24.4375000013656,
-104.958734125));
#8187=CARTESIAN_POINT('Ctrl Pts',(43.4753311640868,24.3750000013656,-104.958734125));
#8188=CARTESIAN_POINT('Ctrl Pts',(74.2170326445434,24.3125000013656,-74.2170326445434));
#8189=CARTESIAN_POINT('Ctrl Pts',(104.958734125,24.2500000013656,-43.4753311640868));
#8190=CARTESIAN_POINT('Ctrl Pts',(104.958734125,24.1875000013656,-1.28537377788739E-14));
#8191=CARTESIAN_POINT('Ctrl Pts',(104.958734125,24.1250000013656,43.4753311640868));
#8192=CARTESIAN_POINT('Ctrl Pts',(74.2170326445434,24.0625000013656,74.2170326445434));
#8193=CARTESIAN_POINT('Ctrl Pts',(43.4753311640869,24.0000000013656,104.958734125));
#8194=CARTESIAN_POINT('Ctrl Pts',(1.92806066683109E-14,23.9375000013656,
104.958734125));
#8195=CARTESIAN_POINT('Ctrl Pts',(-43.4753311640868,23.8750000013656,104.958734125));
#8196=CARTESIAN_POINT('Ctrl Pts',(-74.2170326445434,23.8125000013656,74.2170326445434));
#8197=CARTESIAN_POINT('Ctrl Pts',(-104.958734125,23.7500000013656,43.4753311640869));
#8198=CARTESIAN_POINT('Ctrl Pts',(-104.958734125,23.6875000013656,0.));
#8199=CARTESIAN_POINT('Ctrl Pts',(-104.958734125,23.6250000013656,-43.4753311640868));
#8200=CARTESIAN_POINT('Ctrl Pts',(-74.2170326445434,23.5625000013656,-74.2170326445434));
#8201=CARTESIAN_POINT('Ctrl Pts',(-43.4753311640868,23.5000000013656,-104.958734125));
#8202=CARTESIAN_POINT('Ctrl Pts',(-6.42686888943697E-15,23.4375000013656,
-104.958734125));
#8203=CARTESIAN_POINT('Ctrl Pts',(43.4753311640868,23.3750000013656,-104.958734125));
#8204=CARTESIAN_POINT('Ctrl Pts',(74.2170326445434,23.3125000013656,-74.2170326445434));
#8205=CARTESIAN_POINT('Ctrl Pts',(104.958734125,23.2500000013656,-43.4753311640868));
#8206=CARTESIAN_POINT('Ctrl Pts',(104.958734125,23.1875000013656,-1.28537377788739E-14));
#8207=CARTESIAN_POINT('Ctrl Pts',(104.958734125,23.1250000013656,43.4753311640868));
#8208=CARTESIAN_POINT('Ctrl Pts',(74.2170326445434,23.0625000013656,74.2170326445434));
#8209=CARTESIAN_POINT('Ctrl Pts',(43.4753311640869,23.0000000013656,104.958734125));
#8210=CARTESIAN_POINT('Ctrl Pts',(1.92806066683109E-14,22.9375000013656,
104.958734125));
#8211=CARTESIAN_POINT('Ctrl Pts',(-43.4753311640868,22.8750000013656,104.958734125));
#8212=CARTESIAN_POINT('Ctrl Pts',(-74.2170326445434,22.8125000013656,74.2170326445434));
#8213=CARTESIAN_POINT('Ctrl Pts',(-104.958734125,22.7500000013656,43.4753311640869));
#8214=CARTESIAN_POINT('Ctrl Pts',(-104.958734125,22.6875000013656,0.));
#8215=CARTESIAN_POINT('Ctrl Pts',(-104.958734125,22.6250000013656,-43.4753311640868));
#8216=CARTESIAN_POINT('Ctrl Pts',(-74.2170326445434,22.5625000013656,-74.2170326445434));
#8217=CARTESIAN_POINT('Ctrl Pts',(-43.4753311640868,22.5000000013656,-104.958734125));
#8218=CARTESIAN_POINT('Ctrl Pts',(-6.42686888943697E-15,22.4375000013656,
-104.958734125));
#8219=CARTESIAN_POINT('Ctrl Pts',(43.4753311640868,22.3750000013656,-104.958734125));
#8220=CARTESIAN_POINT('Ctrl Pts',(74.2170326445434,22.3125000013656,-74.2170326445434));
#8221=CARTESIAN_POINT('Ctrl Pts',(104.958734125,22.2500000013656,-43.4753311640868));
#8222=CARTESIAN_POINT('Ctrl Pts',(104.958734125,22.1875000013656,-1.28537377788739E-14));
#8223=CARTESIAN_POINT('Ctrl Pts',(104.958734125,22.1250000013656,43.4753311640868));
#8224=CARTESIAN_POINT('Ctrl Pts',(74.2170326445434,22.0625000013656,74.2170326445434));
#8225=CARTESIAN_POINT('Ctrl Pts',(43.4753311640869,22.0000000013656,104.958734125));
#8226=CARTESIAN_POINT('Ctrl Pts',(1.92806066683109E-14,21.9375000013656,
104.958734125));
#8227=CARTESIAN_POINT('Ctrl Pts',(-43.4753311640868,21.8750000013656,104.958734125));
#8228=CARTESIAN_POINT('Ctrl Pts',(-74.2170326445434,21.8125000013656,74.2170326445434));
#8229=CARTESIAN_POINT('Ctrl Pts',(-104.958734125,21.7500000013656,43.4753311640869));
#8230=CARTESIAN_POINT('Ctrl Pts',(-104.958734125,21.6875000013656,0.));
#8231=CARTESIAN_POINT('Ctrl Pts',(-104.958734125,21.6250000013656,-43.4753311640868));
#8232=CARTESIAN_POINT('Ctrl Pts',(-74.2170326445434,21.5625000013656,-74.2170326445434));
#8233=CARTESIAN_POINT('Ctrl Pts',(-43.4753311640868,21.5000000013656,-104.958734125));
#8234=CARTESIAN_POINT('Ctrl Pts',(-6.42686888943697E-15,21.4375000013656,
-104.958734125));
#8235=CARTESIAN_POINT('Ctrl Pts',(43.4753311640868,21.3750000013656,-104.958734125));
#8236=CARTESIAN_POINT('Ctrl Pts',(74.2170326445434,21.3125000013656,-74.2170326445434));
#8237=CARTESIAN_POINT('Ctrl Pts',(104.958734125,21.2500000013656,-43.4753311640868));
#8238=CARTESIAN_POINT('Ctrl Pts',(104.958734125,21.1875000013656,-1.28537377788739E-14));
#8239=CARTESIAN_POINT('Ctrl Pts',(104.958734125,21.1250000013656,43.4753311640868));
#8240=CARTESIAN_POINT('Ctrl Pts',(74.2170326445434,21.0625000013656,74.2170326445434));
#8241=CARTESIAN_POINT('Ctrl Pts',(43.4753311640869,21.0000000013656,104.958734125));
#8242=CARTESIAN_POINT('Ctrl Pts',(1.92806066683109E-14,20.9375000013656,
104.958734125));
#8243=CARTESIAN_POINT('Ctrl Pts',(-43.4753311640868,20.8750000013656,104.958734125));
#8244=CARTESIAN_POINT('Ctrl Pts',(-74.2170326445434,20.8125000013656,74.2170326445434));
#8245=CARTESIAN_POINT('Ctrl Pts',(-104.958734125,20.7500000013656,43.4753311640869));
#8246=CARTESIAN_POINT('Ctrl Pts',(-104.958734125,20.6875000013656,0.));
#8247=CARTESIAN_POINT('Ctrl Pts',(-104.958734125,20.6250000013656,-43.4753311640868));
#8248=CARTESIAN_POINT('Ctrl Pts',(-74.2170326445434,20.5625000013656,-74.2170326445434));
#8249=CARTESIAN_POINT('Ctrl Pts',(-43.4753311640868,20.5000000013656,-104.958734125));
#8250=CARTESIAN_POINT('Ctrl Pts',(-6.42686888943697E-15,20.4375000013656,
-104.958734125));
#8251=CARTESIAN_POINT('Ctrl Pts',(43.4753311640868,20.3750000013656,-104.958734125));
#8252=CARTESIAN_POINT('Ctrl Pts',(74.2170326445434,20.3125000013656,-74.2170326445434));
#8253=CARTESIAN_POINT('Ctrl Pts',(104.958734125,20.2500000013656,-43.4753311640868));
#8254=CARTESIAN_POINT('Ctrl Pts',(104.958734125,20.1875000013656,-1.28537377788739E-14));
#8255=CARTESIAN_POINT('Ctrl Pts',(104.958734125,20.1250000013656,43.4753311640868));
#8256=CARTESIAN_POINT('Ctrl Pts',(74.2170326445434,20.0625000013656,74.2170326445434));
#8257=CARTESIAN_POINT('Ctrl Pts',(43.4753311640869,20.0000000013656,104.958734125));
#8258=CARTESIAN_POINT('Ctrl Pts',(1.92806066683109E-14,19.9375000013656,
104.958734125));
#8259=CARTESIAN_POINT('Ctrl Pts',(-43.4753311640868,19.8750000013656,104.958734125));
#8260=CARTESIAN_POINT('Ctrl Pts',(-74.2170326445434,19.8125000013656,74.2170326445434));
#8261=CARTESIAN_POINT('Ctrl Pts',(-104.958734125,19.7500000013656,43.4753311640869));
#8262=CARTESIAN_POINT('Ctrl Pts',(-104.958734125,19.6875000013656,0.));
#8263=CARTESIAN_POINT('Ctrl Pts',(-104.958734125,19.6250000013656,-43.4753311640868));
#8264=CARTESIAN_POINT('Ctrl Pts',(-74.2170326445434,19.5625000013656,-74.2170326445434));
#8265=CARTESIAN_POINT('Ctrl Pts',(-43.4753311640868,19.5000000013656,-104.958734125));
#8266=CARTESIAN_POINT('Ctrl Pts',(-6.42686888943697E-15,19.4375000013656,
-104.958734125));
#8267=CARTESIAN_POINT('Ctrl Pts',(43.4753311640868,19.3750000013656,-104.958734125));
#8268=CARTESIAN_POINT('Ctrl Pts',(74.2170326445434,19.3125000013656,-74.2170326445434));
#8269=CARTESIAN_POINT('Ctrl Pts',(104.958734125,19.2500000013656,-43.4753311640868));
#8270=CARTESIAN_POINT('Ctrl Pts',(104.958734125,19.1875000013656,-1.28537377788739E-14));
#8271=CARTESIAN_POINT('Ctrl Pts',(104.958734125,19.1250000013656,43.4753311640868));
#8272=CARTESIAN_POINT('Ctrl Pts',(74.2170326445434,19.0625000013656,74.2170326445434));
#8273=CARTESIAN_POINT('Ctrl Pts',(43.4753311640869,19.0000000013656,104.958734125));
#8274=CARTESIAN_POINT('Ctrl Pts',(1.92806066683109E-14,18.9375000013656,
104.958734125));
#8275=CARTESIAN_POINT('Ctrl Pts',(-43.4753311640868,18.8750000013656,104.958734125));
#8276=CARTESIAN_POINT('Ctrl Pts',(-74.2170326445434,18.8125000013656,74.2170326445434));
#8277=CARTESIAN_POINT('Ctrl Pts',(-104.958734125,18.7500000013656,43.4753311640869));
#8278=CARTESIAN_POINT('Ctrl Pts',(-104.958734125,18.6875000013656,0.));
#8279=CARTESIAN_POINT('Ctrl Pts',(-104.958734125,18.6250000013656,-43.4753311640868));
#8280=CARTESIAN_POINT('Ctrl Pts',(-74.2170326445434,18.5625000013656,-74.2170326445434));
#8281=CARTESIAN_POINT('Ctrl Pts',(-43.4753311640868,18.5000000013656,-104.958734125));
#8282=CARTESIAN_POINT('Ctrl Pts',(-6.42686888943697E-15,18.4375000013656,
-104.958734125));
#8283=CARTESIAN_POINT('Ctrl Pts',(43.4753311640868,18.3750000013656,-104.958734125));
#8284=CARTESIAN_POINT('Ctrl Pts',(74.2170326445434,18.3125000013656,-74.2170326445434));
#8285=CARTESIAN_POINT('Ctrl Pts',(104.958734125,18.2500000013656,-43.4753311640868));
#8286=CARTESIAN_POINT('Ctrl Pts',(104.958734125,18.1875000013656,-1.28537377788739E-14));
#8287=CARTESIAN_POINT('Ctrl Pts',(104.958734125,18.1250000013656,43.4753311640868));
#8288=CARTESIAN_POINT('Ctrl Pts',(74.2170326445434,18.0625000013656,74.2170326445434));
#8289=CARTESIAN_POINT('Ctrl Pts',(43.4753311640869,18.0000000013656,104.958734125));
#8290=CARTESIAN_POINT('Ctrl Pts',(1.92806066683109E-14,17.9375000013656,
104.958734125));
#8291=CARTESIAN_POINT('Ctrl Pts',(-43.4753311640868,17.8750000013656,104.958734125));
#8292=CARTESIAN_POINT('Ctrl Pts',(-74.2170326445434,17.8125000013656,74.2170326445434));
#8293=CARTESIAN_POINT('Ctrl Pts',(-104.958734125,17.7500000013656,43.4753311640869));
#8294=CARTESIAN_POINT('Ctrl Pts',(-104.958734125,17.6875000013656,0.));
#8295=CARTESIAN_POINT('Ctrl Pts',(-104.958734125,17.6250000013656,-43.4753311640868));
#8296=CARTESIAN_POINT('Ctrl Pts',(-74.2170326445434,17.5625000013656,-74.2170326445434));
#8297=CARTESIAN_POINT('Ctrl Pts',(-43.4753311640868,17.5000000013656,-104.958734125));
#8298=CARTESIAN_POINT('Ctrl Pts',(-6.42686888943697E-15,17.4375000013656,
-104.958734125));
#8299=CARTESIAN_POINT('Ctrl Pts',(43.4753311640868,17.3750000013656,-104.958734125));
#8300=CARTESIAN_POINT('Ctrl Pts',(74.2170326445434,17.3125000013656,-74.2170326445434));
#8301=CARTESIAN_POINT('Ctrl Pts',(104.958734125,17.2500000013656,-43.4753311640868));
#8302=CARTESIAN_POINT('Ctrl Pts',(104.958734125,17.1875000013656,-1.28537377788739E-14));
#8303=CARTESIAN_POINT('Ctrl Pts',(104.958734125,17.1250000013656,43.4753311640868));
#8304=CARTESIAN_POINT('Ctrl Pts',(74.2170326445434,17.0625000013656,74.2170326445434));
#8305=CARTESIAN_POINT('Ctrl Pts',(43.4753311640869,17.0000000013656,104.958734125));
#8306=CARTESIAN_POINT('Ctrl Pts',(1.92806066683109E-14,16.9375000013656,
104.958734125));
#8307=CARTESIAN_POINT('Ctrl Pts',(-43.4753311640868,16.8750000013656,104.958734125));
#8308=CARTESIAN_POINT('Ctrl Pts',(-74.2170326445434,16.8125000013656,74.2170326445434));
#8309=CARTESIAN_POINT('Ctrl Pts',(-104.958734125,16.7500000013656,43.4753311640869));
#8310=CARTESIAN_POINT('Ctrl Pts',(-104.958734125,16.6875000013656,0.));
#8311=CARTESIAN_POINT('Ctrl Pts',(-104.958734125,16.6250000013656,-43.4753311640868));
#8312=CARTESIAN_POINT('Ctrl Pts',(-74.2170326445434,16.5625000013656,-74.2170326445434));
#8313=CARTESIAN_POINT('Ctrl Pts',(-43.4753311640868,16.5000000013656,-104.958734125));
#8314=CARTESIAN_POINT('Ctrl Pts',(-6.42686888943697E-15,16.4375000013656,
-104.958734125));
#8315=CARTESIAN_POINT('Ctrl Pts',(43.4753311640868,16.3750000013656,-104.958734125));
#8316=CARTESIAN_POINT('Ctrl Pts',(74.2170326445434,16.3125000013656,-74.2170326445434));
#8317=CARTESIAN_POINT('Ctrl Pts',(104.958734125,16.2500000013656,-43.4753311640868));
#8318=CARTESIAN_POINT('Ctrl Pts',(104.958734125,16.1875000013656,-1.28537377788739E-14));
#8319=CARTESIAN_POINT('Ctrl Pts',(104.958734125,16.1250000013656,43.4753311640868));
#8320=CARTESIAN_POINT('Ctrl Pts',(74.2170326445434,16.0625000013656,74.2170326445434));
#8321=CARTESIAN_POINT('Ctrl Pts',(43.4753311640869,16.0000000013656,104.958734125));
#8322=CARTESIAN_POINT('Ctrl Pts',(1.92806066683109E-14,15.9375000013656,
104.958734125));
#8323=CARTESIAN_POINT('Ctrl Pts',(-43.4753311640868,15.8750000013656,104.958734125));
#8324=CARTESIAN_POINT('Ctrl Pts',(-74.2170326445434,15.8125000013656,74.2170326445434));
#8325=CARTESIAN_POINT('Ctrl Pts',(-104.958734125,15.7500000013656,43.4753311640869));
#8326=CARTESIAN_POINT('Ctrl Pts',(-104.958734125,15.6875000013656,0.));
#8327=CARTESIAN_POINT('Ctrl Pts',(-104.958734125,15.6250000013656,-43.4753311640868));
#8328=CARTESIAN_POINT('Ctrl Pts',(-74.2170326445434,15.5625000013656,-74.2170326445434));
#8329=CARTESIAN_POINT('Ctrl Pts',(-43.4753311640868,15.5000000013656,-104.958734125));
#8330=CARTESIAN_POINT('Ctrl Pts',(-6.42686888943697E-15,15.4375000013656,
-104.958734125));
#8331=CARTESIAN_POINT('Ctrl Pts',(43.4753311640868,15.3750000013656,-104.958734125));
#8332=CARTESIAN_POINT('Ctrl Pts',(74.2170326445434,15.3125000013656,-74.2170326445434));
#8333=CARTESIAN_POINT('Ctrl Pts',(104.958734125,15.2500000013656,-43.4753311640868));
#8334=CARTESIAN_POINT('Ctrl Pts',(104.958734125,15.1875000013656,-1.28537377788739E-14));
#8335=CARTESIAN_POINT('Ctrl Pts',(104.958734125,15.1250000013656,43.4753311640868));
#8336=CARTESIAN_POINT('Ctrl Pts',(74.2170326445434,15.0625000013656,74.2170326445434));
#8337=CARTESIAN_POINT('Ctrl Pts',(43.4753311640869,15.0000000013656,104.958734125));
#8338=CARTESIAN_POINT('Ctrl Pts',(1.92806066683109E-14,14.9375000013656,
104.958734125));
#8339=CARTESIAN_POINT('Ctrl Pts',(-43.4753311640868,14.8750000013656,104.958734125));
#8340=CARTESIAN_POINT('Ctrl Pts',(-74.2170326445434,14.8125000013656,74.2170326445434));
#8341=CARTESIAN_POINT('Ctrl Pts',(-104.958734125,14.7500000013656,43.4753311640869));
#8342=CARTESIAN_POINT('Ctrl Pts',(-104.958734125,14.6875000013656,0.));
#8343=CARTESIAN_POINT('Ctrl Pts',(-104.958734125,14.6250000013656,-43.4753311640868));
#8344=CARTESIAN_POINT('Ctrl Pts',(-74.2170326445434,14.5625000013656,-74.2170326445434));
#8345=CARTESIAN_POINT('Ctrl Pts',(-43.4753311640868,14.5000000013656,-104.958734125));
#8346=CARTESIAN_POINT('Ctrl Pts',(-6.42686888943697E-15,14.4375000013656,
-104.958734125));
#8347=CARTESIAN_POINT('Ctrl Pts',(43.4753311640868,14.3750000013656,-104.958734125));
#8348=CARTESIAN_POINT('Ctrl Pts',(74.2170326445434,14.3125000013656,-74.2170326445434));
#8349=CARTESIAN_POINT('Ctrl Pts',(104.958734125,14.2500000013656,-43.4753311640868));
#8350=CARTESIAN_POINT('Ctrl Pts',(104.958734125,14.1875000013656,-1.28537377788739E-14));
#8351=CARTESIAN_POINT('Ctrl Pts',(104.958734125,14.1250000013656,43.4753311640868));
#8352=CARTESIAN_POINT('Ctrl Pts',(74.2170326445434,14.0625000013656,74.2170326445434));
#8353=CARTESIAN_POINT('Ctrl Pts',(43.4753311640869,14.0000000013656,104.958734125));
#8354=CARTESIAN_POINT('Ctrl Pts',(1.92806066683109E-14,13.9375000013656,
104.958734125));
#8355=CARTESIAN_POINT('Ctrl Pts',(-43.4753311640868,13.8750000013656,104.958734125));
#8356=CARTESIAN_POINT('Ctrl Pts',(-74.2170326445434,13.8125000013656,74.2170326445434));
#8357=CARTESIAN_POINT('Ctrl Pts',(-104.958734125,13.7500000013656,43.4753311640869));
#8358=CARTESIAN_POINT('Ctrl Pts',(-104.958734125,13.6875000013656,0.));
#8359=CARTESIAN_POINT('Ctrl Pts',(-104.958734125,13.6250000013656,-43.4753311640868));
#8360=CARTESIAN_POINT('Ctrl Pts',(-74.2170326445434,13.5625000013656,-74.2170326445434));
#8361=CARTESIAN_POINT('Ctrl Pts',(-43.4753311640868,13.5000000013656,-104.958734125));
#8362=CARTESIAN_POINT('Ctrl Pts',(-6.42686888943697E-15,13.4375000013656,
-104.958734125));
#8363=CARTESIAN_POINT('Ctrl Pts',(43.4753311640868,13.3750000013656,-104.958734125));
#8364=CARTESIAN_POINT('Ctrl Pts',(74.2170326445434,13.3125000013656,-74.2170326445434));
#8365=CARTESIAN_POINT('Ctrl Pts',(104.958734125,13.2500000013656,-43.4753311640868));
#8366=CARTESIAN_POINT('Ctrl Pts',(104.958734125,13.1875000013656,-1.28537377788739E-14));
#8367=CARTESIAN_POINT('Ctrl Pts',(104.958734125,13.1250000013656,43.4753311640868));
#8368=CARTESIAN_POINT('Ctrl Pts',(74.2170326445434,13.0625000013656,74.2170326445434));
#8369=CARTESIAN_POINT('Ctrl Pts',(43.4753311640869,13.0000000013656,104.958734125));
#8370=CARTESIAN_POINT('Ctrl Pts',(1.92806066683109E-14,12.9375000013656,
104.958734125));
#8371=CARTESIAN_POINT('Ctrl Pts',(-43.4753311640868,12.8750000013656,104.958734125));
#8372=CARTESIAN_POINT('Ctrl Pts',(-74.2170326445434,12.8125000013656,74.2170326445434));
#8373=CARTESIAN_POINT('Ctrl Pts',(-104.958734125,12.7500000013656,43.4753311640869));
#8374=CARTESIAN_POINT('Ctrl Pts',(-104.958734125,12.6875000013656,0.));
#8375=CARTESIAN_POINT('Ctrl Pts',(-104.958734125,12.6250000013656,-43.4753311640868));
#8376=CARTESIAN_POINT('Ctrl Pts',(-74.2170326445434,12.5625000013656,-74.2170326445434));
#8377=CARTESIAN_POINT('Ctrl Pts',(-43.4753311640868,12.5000000013656,-104.958734125));
#8378=CARTESIAN_POINT('Ctrl Pts',(-6.42686888943697E-15,12.4375000013656,
-104.958734125));
#8379=CARTESIAN_POINT('Ctrl Pts',(43.4753311640868,12.3750000013656,-104.958734125));
#8380=CARTESIAN_POINT('Ctrl Pts',(74.2170326445434,12.3125000013656,-74.2170326445434));
#8381=CARTESIAN_POINT('Ctrl Pts',(104.958734125,12.2500000013656,-43.4753311640868));
#8382=CARTESIAN_POINT('Ctrl Pts',(104.958734125,12.1875000013656,-1.28537377788739E-14));
#8383=CARTESIAN_POINT('Ctrl Pts',(104.958734125,12.1250000013656,43.4753311640868));
#8384=CARTESIAN_POINT('Ctrl Pts',(74.2170326445434,12.0625000013656,74.2170326445434));
#8385=CARTESIAN_POINT('Ctrl Pts',(43.4753311640869,12.0000000013656,104.958734125));
#8386=CARTESIAN_POINT('Ctrl Pts',(1.92806066683109E-14,11.9375000013656,
104.958734125));
#8387=CARTESIAN_POINT('Ctrl Pts',(-43.4753311640868,11.8750000013656,104.958734125));
#8388=CARTESIAN_POINT('Ctrl Pts',(-74.2170326445434,11.8125000013656,74.2170326445434));
#8389=CARTESIAN_POINT('Ctrl Pts',(-104.958734125,11.7500000013656,43.4753311640869));
#8390=CARTESIAN_POINT('Ctrl Pts',(-104.958734125,11.6875000013656,0.));
#8391=CARTESIAN_POINT('Ctrl Pts',(-104.958734125,11.6250000013656,-43.4753311640868));
#8392=CARTESIAN_POINT('Ctrl Pts',(-74.2170326445434,11.5625000013656,-74.2170326445434));
#8393=CARTESIAN_POINT('Ctrl Pts',(-43.4753311640868,11.5000000013656,-104.958734125));
#8394=CARTESIAN_POINT('Ctrl Pts',(-6.42686888943697E-15,11.4375000013656,
-104.958734125));
#8395=CARTESIAN_POINT('Ctrl Pts',(43.4753311640868,11.3750000013656,-104.958734125));
#8396=CARTESIAN_POINT('Ctrl Pts',(74.2170326445434,11.3125000013656,-74.2170326445434));
#8397=CARTESIAN_POINT('Ctrl Pts',(104.958734125,11.2500000013656,-43.4753311640868));
#8398=CARTESIAN_POINT('Ctrl Pts',(104.958734125,11.1875000013656,-1.28537377788739E-14));
#8399=CARTESIAN_POINT('Ctrl Pts',(104.958734125,11.1250000013656,43.4753311640868));
#8400=CARTESIAN_POINT('Ctrl Pts',(74.2170326445434,11.0625000013656,74.2170326445434));
#8401=CARTESIAN_POINT('Ctrl Pts',(43.4753311640869,11.0000000013656,104.958734125));
#8402=CARTESIAN_POINT('Ctrl Pts',(1.92806066683109E-14,10.9375000013656,
104.958734125));
#8403=CARTESIAN_POINT('Ctrl Pts',(-43.4753311640868,10.8750000013656,104.958734125));
#8404=CARTESIAN_POINT('Ctrl Pts',(-74.2170326445434,10.8125000013656,74.2170326445434));
#8405=CARTESIAN_POINT('Ctrl Pts',(-104.958734125,10.7500000013656,43.4753311640869));
#8406=CARTESIAN_POINT('Ctrl Pts',(-104.958734125,10.6875000013656,0.));
#8407=CARTESIAN_POINT('Ctrl Pts',(-104.958734125,10.6250000013656,-43.4753311640868));
#8408=CARTESIAN_POINT('Ctrl Pts',(-74.2170326445434,10.5625000013656,-74.2170326445434));
#8409=CARTESIAN_POINT('Ctrl Pts',(-43.4753311640868,10.5000000013656,-104.958734125));
#8410=CARTESIAN_POINT('Ctrl Pts',(-6.42686888943697E-15,10.4375000013656,
-104.958734125));
#8411=CARTESIAN_POINT('Ctrl Pts',(43.4753311640868,10.3750000013656,-104.958734125));
#8412=CARTESIAN_POINT('Ctrl Pts',(74.2170326445434,10.3125000013656,-74.2170326445434));
#8413=CARTESIAN_POINT('Ctrl Pts',(104.958734125,10.2500000013656,-43.4753311640868));
#8414=CARTESIAN_POINT('Ctrl Pts',(104.958734125,10.1875000013656,-1.28537377788739E-14));
#8415=CARTESIAN_POINT('Ctrl Pts',(104.958734125,10.1250000013656,43.4753311640868));
#8416=CARTESIAN_POINT('Ctrl Pts',(74.2170326445434,10.0625000013656,74.2170326445434));
#8417=CARTESIAN_POINT('Ctrl Pts',(43.4753311640869,10.0000000013656,104.958734125));
#8418=CARTESIAN_POINT('Ctrl Pts',(1.92806066683109E-14,9.93750000136558,
104.958734125));
#8419=CARTESIAN_POINT('Ctrl Pts',(-43.4753311640868,9.87500000136558,104.958734125));
#8420=CARTESIAN_POINT('Ctrl Pts',(-74.2170326445434,9.81250000136558,74.2170326445434));
#8421=CARTESIAN_POINT('Ctrl Pts',(-104.958734125,9.75000000136558,43.4753311640869));
#8422=CARTESIAN_POINT('Ctrl Pts',(-104.958734125,9.68750000136558,0.));
#8423=CARTESIAN_POINT('Ctrl Pts',(-104.958734125,9.62500000136558,-43.4753311640868));
#8424=CARTESIAN_POINT('Ctrl Pts',(-74.2170326445434,9.56250000136558,-74.2170326445434));
#8425=CARTESIAN_POINT('Ctrl Pts',(-43.4753311640868,9.50000000136558,-104.958734125));
#8426=CARTESIAN_POINT('Ctrl Pts',(-6.42686888943697E-15,9.43750000136558,
-104.958734125));
#8427=CARTESIAN_POINT('Ctrl Pts',(43.4753311640868,9.37500000136558,-104.958734125));
#8428=CARTESIAN_POINT('Ctrl Pts',(74.2170326445434,9.31250000136558,-74.2170326445434));
#8429=CARTESIAN_POINT('Ctrl Pts',(104.958734125,9.25000000136558,-43.4753311640868));
#8430=CARTESIAN_POINT('Ctrl Pts',(104.958734125,9.18750000136558,-1.28537377788739E-14));
#8431=CARTESIAN_POINT('Ctrl Pts',(104.958734125,9.12500000136558,43.4753311640868));
#8432=CARTESIAN_POINT('Ctrl Pts',(74.2170326445434,9.06250000136558,74.2170326445434));
#8433=CARTESIAN_POINT('Ctrl Pts',(43.4753311640869,9.00000000136558,104.958734125));
#8434=CARTESIAN_POINT('Ctrl Pts',(1.92806066683109E-14,8.93750000136558,
104.958734125));
#8435=CARTESIAN_POINT('Ctrl Pts',(-43.4753311640868,8.87500000136558,104.958734125));
#8436=CARTESIAN_POINT('Ctrl Pts',(-74.2170326445434,8.81250000136558,74.2170326445434));
#8437=CARTESIAN_POINT('Ctrl Pts',(-104.958734125,8.75000000136558,43.4753311640869));
#8438=CARTESIAN_POINT('Ctrl Pts',(-104.958734125,8.68750000136558,0.));
#8439=CARTESIAN_POINT('Ctrl Pts',(-104.958734125,8.62500000136558,-43.4753311640868));
#8440=CARTESIAN_POINT('Ctrl Pts',(-74.2170326445434,8.56250000136558,-74.2170326445434));
#8441=CARTESIAN_POINT('Ctrl Pts',(-43.4753311640868,8.50000000136558,-104.958734125));
#8442=CARTESIAN_POINT('Ctrl Pts',(-6.42686888943697E-15,8.43750000136558,
-104.958734125));
#8443=CARTESIAN_POINT('Ctrl Pts',(43.4753311640868,8.37500000136558,-104.958734125));
#8444=CARTESIAN_POINT('Ctrl Pts',(74.2170326445434,8.31250000136558,-74.2170326445434));
#8445=CARTESIAN_POINT('Ctrl Pts',(104.958734125,8.25000000136558,-43.4753311640868));
#8446=CARTESIAN_POINT('Ctrl Pts',(104.958734125,8.18750000136558,-1.28537377788739E-14));
#8447=CARTESIAN_POINT('Ctrl Pts',(104.958734125,8.12500000136558,43.4753311640868));
#8448=CARTESIAN_POINT('Ctrl Pts',(74.2170326445434,8.06250000136558,74.2170326445434));
#8449=CARTESIAN_POINT('Ctrl Pts',(43.4753311640869,8.00000000136558,104.958734125));
#8450=CARTESIAN_POINT('Ctrl Pts',(1.92806066683109E-14,7.93750000136558,
104.958734125));
#8451=CARTESIAN_POINT('Ctrl Pts',(-43.4753311640868,7.87500000136558,104.958734125));
#8452=CARTESIAN_POINT('Ctrl Pts',(-74.2170326445434,7.81250000136558,74.2170326445434));
#8453=CARTESIAN_POINT('Ctrl Pts',(-104.958734125,7.75000000136558,43.4753311640869));
#8454=CARTESIAN_POINT('Ctrl Pts',(-104.958734125,7.68750000136558,0.));
#8455=CARTESIAN_POINT('Ctrl Pts',(-104.958734125,7.62500000136558,-43.4753311640868));
#8456=CARTESIAN_POINT('Ctrl Pts',(-74.2170326445434,7.56250000136558,-74.2170326445434));
#8457=CARTESIAN_POINT('Ctrl Pts',(-43.4753311640868,7.50000000136558,-104.958734125));
#8458=CARTESIAN_POINT('Ctrl Pts',(-6.42686888943697E-15,7.43750000136558,
-104.958734125));
#8459=CARTESIAN_POINT('Ctrl Pts',(43.4753311640868,7.37500000136558,-104.958734125));
#8460=CARTESIAN_POINT('Ctrl Pts',(74.2170326445434,7.31250000136558,-74.2170326445434));
#8461=CARTESIAN_POINT('Ctrl Pts',(104.958734125,7.25000000136558,-43.4753311640868));
#8462=CARTESIAN_POINT('Ctrl Pts',(104.958734125,7.18750000136558,-1.28537377788739E-14));
#8463=CARTESIAN_POINT('Ctrl Pts',(104.958734125,7.12500000136558,43.4753311640868));
#8464=CARTESIAN_POINT('Ctrl Pts',(74.2170326445434,7.06250000136558,74.2170326445434));
#8465=CARTESIAN_POINT('Ctrl Pts',(43.4753311640869,7.00000000136558,104.958734125));
#8466=CARTESIAN_POINT('Ctrl Pts',(1.92806066683109E-14,6.93750000136558,
104.958734125));
#8467=CARTESIAN_POINT('Ctrl Pts',(-43.4753311640868,6.87500000136558,104.958734125));
#8468=CARTESIAN_POINT('Ctrl Pts',(-74.2170326445434,6.81250000136558,74.2170326445434));
#8469=CARTESIAN_POINT('Ctrl Pts',(-104.958734125,6.75000000136558,43.4753311640869));
#8470=CARTESIAN_POINT('Ctrl Pts',(-104.958734125,6.68750000136558,0.));
#8471=CARTESIAN_POINT('Ctrl Pts',(-104.958734125,6.62500000136558,-43.4753311640868));
#8472=CARTESIAN_POINT('Ctrl Pts',(-74.2170326445434,6.56250000136558,-74.2170326445434));
#8473=CARTESIAN_POINT('Ctrl Pts',(-43.4753311640868,6.50000000136558,-104.958734125));
#8474=CARTESIAN_POINT('Ctrl Pts',(-6.42686888943697E-15,6.43750000136558,
-104.958734125));
#8475=CARTESIAN_POINT('Ctrl Pts',(43.4753311640868,6.37500000136558,-104.958734125));
#8476=CARTESIAN_POINT('Ctrl Pts',(74.2170326445434,6.31250000136558,-74.2170326445434));
#8477=CARTESIAN_POINT('Ctrl Pts',(104.958734125,6.25000000136558,-43.4753311640868));
#8478=CARTESIAN_POINT('Ctrl Pts',(104.958734125,6.18750000136558,-1.28537377788739E-14));
#8479=CARTESIAN_POINT('Ctrl Pts',(104.958734125,6.12500000136558,43.4753311640868));
#8480=CARTESIAN_POINT('Ctrl Pts',(74.2170326445434,6.06250000136558,74.2170326445434));
#8481=CARTESIAN_POINT('Ctrl Pts',(43.4753311640869,6.00000000136558,104.958734125));
#8482=CARTESIAN_POINT('Ctrl Pts',(1.92806066683109E-14,5.93750000136558,
104.958734125));
#8483=CARTESIAN_POINT('Ctrl Pts',(-43.4753311640868,5.87500000136558,104.958734125));
#8484=CARTESIAN_POINT('Ctrl Pts',(-74.2170326445434,5.81250000136558,74.2170326445434));
#8485=CARTESIAN_POINT('Ctrl Pts',(-104.958734125,5.75000000136558,43.4753311640869));
#8486=CARTESIAN_POINT('Ctrl Pts',(-104.958734125,5.68750000136559,0.));
#8487=CARTESIAN_POINT('Ctrl Pts',(-104.958734125,5.62500000136559,-43.4753311640868));
#8488=CARTESIAN_POINT('Ctrl Pts',(-74.2170326445434,5.56250000136559,-74.2170326445434));
#8489=CARTESIAN_POINT('Ctrl Pts',(-43.4753311640868,5.50000000136559,-104.958734125));
#8490=CARTESIAN_POINT('Ctrl Pts',(-6.42686888943697E-15,5.43750000136559,
-104.958734125));
#8491=CARTESIAN_POINT('Ctrl Pts',(43.4753311640868,5.37500000136559,-104.958734125));
#8492=CARTESIAN_POINT('Ctrl Pts',(74.2170326445434,5.31250000136558,-74.2170326445434));
#8493=CARTESIAN_POINT('Ctrl Pts',(104.958734125,5.25000000136559,-43.4753311640868));
#8494=CARTESIAN_POINT('Ctrl Pts',(104.958734125,5.18750000136559,-1.28537377788739E-14));
#8495=CARTESIAN_POINT('Ctrl Pts',(104.958734125,5.12500000136559,43.4753311640868));
#8496=CARTESIAN_POINT('Ctrl Pts',(74.2170326445434,5.06250000136559,74.2170326445434));
#8497=CARTESIAN_POINT('Ctrl Pts',(43.4753311640869,5.00000000136558,104.958734125));
#8498=CARTESIAN_POINT('Ctrl Pts',(1.92806066683109E-14,4.93750000136559,
104.958734125));
#8499=CARTESIAN_POINT('Ctrl Pts',(-43.4753311640868,4.87500000136559,104.958734125));
#8500=CARTESIAN_POINT('Ctrl Pts',(-74.2170326445434,4.81250000136559,74.2170326445434));
#8501=CARTESIAN_POINT('Ctrl Pts',(-104.958734125,4.75000000136558,43.4753311640869));
#8502=CARTESIAN_POINT('Ctrl Pts',(-104.958734125,4.68750000136558,0.));
#8503=CARTESIAN_POINT('Ctrl Pts',(-104.958734125,4.62500000136559,-43.4753311640868));
#8504=CARTESIAN_POINT('Ctrl Pts',(-74.2170326445434,4.56250000136558,-74.2170326445434));
#8505=CARTESIAN_POINT('Ctrl Pts',(-43.4753311640868,4.50000000136558,-104.958734125));
#8506=CARTESIAN_POINT('Ctrl Pts',(-6.42686888943697E-15,4.43750000136558,
-104.958734125));
#8507=CARTESIAN_POINT('Ctrl Pts',(43.4753311640868,4.37500000136558,-104.958734125));
#8508=CARTESIAN_POINT('Ctrl Pts',(74.2170326445434,4.31250000136558,-74.2170326445434));
#8509=CARTESIAN_POINT('Ctrl Pts',(104.958734125,4.25000000136558,-43.4753311640868));
#8510=CARTESIAN_POINT('Ctrl Pts',(104.958734125,4.18750000136558,-1.28537377788739E-14));
#8511=CARTESIAN_POINT('Ctrl Pts',(104.958734125,4.12500000136558,43.4753311640868));
#8512=CARTESIAN_POINT('Ctrl Pts',(74.2170326445434,4.06250000136558,74.2170326445434));
#8513=CARTESIAN_POINT('Ctrl Pts',(43.4753311640869,4.00000000136558,104.958734125));
#8514=CARTESIAN_POINT('Ctrl Pts',(1.92806066683109E-14,3.93750000136558,
104.958734125));
#8515=CARTESIAN_POINT('Ctrl Pts',(-43.4753311640868,3.87500000136558,104.958734125));
#8516=CARTESIAN_POINT('Ctrl Pts',(-74.2170326445434,3.81250000136558,74.2170326445434));
#8517=CARTESIAN_POINT('Ctrl Pts',(-104.958734125,3.75000000136558,43.4753311640869));
#8518=CARTESIAN_POINT('Ctrl Pts',(-104.958734125,3.68750000136558,0.));
#8519=CARTESIAN_POINT('Ctrl Pts',(-104.958734125,3.62500000136558,-43.4753311640868));
#8520=CARTESIAN_POINT('Ctrl Pts',(-74.2170326445434,3.56250000136558,-74.2170326445434));
#8521=CARTESIAN_POINT('Ctrl Pts',(-43.4753311640868,3.50000000136558,-104.958734125));
#8522=CARTESIAN_POINT('Ctrl Pts',(-6.42686888943697E-15,3.43750000136558,
-104.958734125));
#8523=CARTESIAN_POINT('Ctrl Pts',(43.4753311640868,3.37500000136558,-104.958734125));
#8524=CARTESIAN_POINT('Ctrl Pts',(74.2170326445434,3.31250000136558,-74.2170326445434));
#8525=CARTESIAN_POINT('Ctrl Pts',(104.958734125,3.25000000136558,-43.4753311640868));
#8526=CARTESIAN_POINT('Ctrl Pts',(104.958734125,3.18750000136558,-1.28537377788739E-14));
#8527=CARTESIAN_POINT('Ctrl Pts',(104.958734125,3.12500000136558,43.4753311640868));
#8528=CARTESIAN_POINT('Ctrl Pts',(74.2170326445434,3.06250000136558,74.2170326445434));
#8529=CARTESIAN_POINT('Ctrl Pts',(43.4753311640869,3.00000000136558,104.958734125));
#8530=CARTESIAN_POINT('Ctrl Pts',(1.92806066683109E-14,2.93750000136558,
104.958734125));
#8531=CARTESIAN_POINT('Ctrl Pts',(-43.4753311640868,2.87500000136558,104.958734125));
#8532=CARTESIAN_POINT('Ctrl Pts',(-74.2170326445434,2.81250000136558,74.2170326445434));
#8533=CARTESIAN_POINT('Ctrl Pts',(-104.958734125,2.75000000136558,43.4753311640869));
#8534=CARTESIAN_POINT('Ctrl Pts',(-104.958734125,2.68750000136558,0.));
#8535=CARTESIAN_POINT('Ctrl Pts',(-104.958734125,2.62500000136558,-43.4753311640868));
#8536=CARTESIAN_POINT('Ctrl Pts',(-74.2170326445434,2.56250000136558,-74.2170326445434));
#8537=CARTESIAN_POINT('Ctrl Pts',(-43.4753311640868,2.50000000136558,-104.958734125));
#8538=CARTESIAN_POINT('Ctrl Pts',(-6.42686888943697E-15,2.43750000136558,
-104.958734125));
#8539=CARTESIAN_POINT('Ctrl Pts',(43.4753311640868,2.37500000136558,-104.958734125));
#8540=CARTESIAN_POINT('Ctrl Pts',(74.2170326445434,2.31250000136558,-74.2170326445434));
#8541=CARTESIAN_POINT('Ctrl Pts',(104.958734125,2.25000000136558,-43.4753311640868));
#8542=CARTESIAN_POINT('Ctrl Pts',(104.958734125,2.18750000136558,-1.28537377788739E-14));
#8543=CARTESIAN_POINT('Ctrl Pts',(104.958734125,2.12500000136558,43.4753311640868));
#8544=CARTESIAN_POINT('Ctrl Pts',(74.2170326445434,2.06250000136558,74.2170326445434));
#8545=CARTESIAN_POINT('Ctrl Pts',(43.4753311640869,2.00000000136558,104.958734125));
#8546=CARTESIAN_POINT('Ctrl Pts',(1.92806066683109E-14,1.93750000136558,
104.958734125));
#8547=CARTESIAN_POINT('Ctrl Pts',(-43.4753311640868,1.87500000136558,104.958734125));
#8548=CARTESIAN_POINT('Ctrl Pts',(-74.2170326445434,1.81250000136558,74.2170326445434));
#8549=CARTESIAN_POINT('Ctrl Pts',(-104.958734125,1.75000000136558,43.4753311640869));
#8550=CARTESIAN_POINT('Ctrl Pts',(-104.958734125,1.68750000136558,0.));
#8551=CARTESIAN_POINT('Ctrl Pts',(-104.958734125,1.62500000136558,-43.4753311640868));
#8552=CARTESIAN_POINT('Ctrl Pts',(-74.2170326445434,1.56250000136558,-74.2170326445434));
#8553=CARTESIAN_POINT('Ctrl Pts',(-43.4753311640868,1.50000000136558,-104.958734125));
#8554=CARTESIAN_POINT('Ctrl Pts',(-6.42686888943697E-15,1.43750000136558,
-104.958734125));
#8555=CARTESIAN_POINT('Ctrl Pts',(43.4753311640868,1.37500000136558,-104.958734125));
#8556=CARTESIAN_POINT('Ctrl Pts',(74.2170326445434,1.31250000136558,-74.2170326445434));
#8557=CARTESIAN_POINT('Ctrl Pts',(104.958734125,1.25000000136558,-43.4753311640868));
#8558=CARTESIAN_POINT('Ctrl Pts',(104.958734125,1.18750000136558,-1.28537377788739E-14));
#8559=CARTESIAN_POINT('Ctrl Pts',(104.958734125,1.12500000136558,43.4753311640868));
#8560=CARTESIAN_POINT('Ctrl Pts',(74.2170326445434,1.06250000136558,74.2170326445434));
#8561=CARTESIAN_POINT('Ctrl Pts',(43.4753311640869,1.00000000136558,104.958734125));
#8562=CARTESIAN_POINT('Ctrl Pts',(1.92806066683109E-14,0.937500001365582,
104.958734125));
#8563=CARTESIAN_POINT('Ctrl Pts',(-43.4753311640868,0.875000001365582,104.958734125));
#8564=CARTESIAN_POINT('Ctrl Pts',(-74.2170326445434,0.812500001365582,74.2170326445434));
#8565=CARTESIAN_POINT('Ctrl Pts',(-104.958734125,0.750000001365582,43.4753311640869));
#8566=CARTESIAN_POINT('Ctrl Pts',(-104.958734125,0.687500001365582,0.));
#8567=CARTESIAN_POINT('Ctrl Pts',(-104.958734125,0.625000001365582,-43.4753311640868));
#8568=CARTESIAN_POINT('Ctrl Pts',(-74.2170326445434,0.562500001365582,-74.2170326445434));
#8569=CARTESIAN_POINT('Ctrl Pts',(-43.4753311640868,0.500000001365582,-104.958734125));
#8570=CARTESIAN_POINT('Ctrl Pts',(-6.42686888943697E-15,0.437500001365582,
-104.958734125));
#8571=CARTESIAN_POINT('Ctrl Pts',(43.4753311640868,0.375000001365582,-104.958734125));
#8572=CARTESIAN_POINT('Ctrl Pts',(74.2170326445434,0.312500001365582,-74.2170326445434));
#8573=CARTESIAN_POINT('Ctrl Pts',(104.958734125,0.250000001365581,-43.4753311640868));
#8574=CARTESIAN_POINT('Ctrl Pts',(104.958734125,0.187500001365581,-1.28537377788739E-14));
#8575=CARTESIAN_POINT('Ctrl Pts',(104.958734125,0.125000001365581,43.4753311640868));
#8576=CARTESIAN_POINT('Ctrl Pts',(74.2170326445434,0.0625000013655813,74.2170326445434));
#8577=CARTESIAN_POINT('Ctrl Pts',(43.4753311640869,1.36558125918285E-9,
104.958734125));
#8578=CARTESIAN_POINT('Ctrl Pts',(1.92806066683109E-14,-0.0624999986344188,
104.958734125));
#8579=CARTESIAN_POINT('Ctrl Pts',(-43.4753311640868,-0.124999998634419,
104.958734125));
#8580=CARTESIAN_POINT('Ctrl Pts',(-74.2170326445434,-0.187499998634419,
74.2170326445434));
#8581=CARTESIAN_POINT('Ctrl Pts',(-104.958734125,-0.249999998634419,43.4753311640869));
#8582=CARTESIAN_POINT('Ctrl Pts',(-104.958734125,-0.312499998634419,0.));
#8583=CARTESIAN_POINT('Ctrl Pts',(-105.5,50.,0.));
#8584=CARTESIAN_POINT('Ctrl Pts',(-105.5,49.9375,-43.6995308303615));
#8585=CARTESIAN_POINT('Ctrl Pts',(-74.5997654151808,49.875,-74.5997654151808));
#8586=CARTESIAN_POINT('Ctrl Pts',(-43.6995308303615,49.8125,-105.5));
#8587=CARTESIAN_POINT('Ctrl Pts',(-6.46001186550229E-15,49.75,-105.5));
#8588=CARTESIAN_POINT('Ctrl Pts',(43.6995308303615,49.6875,-105.5));
#8589=CARTESIAN_POINT('Ctrl Pts',(74.5997654151808,49.625,-74.5997654151808));
#8590=CARTESIAN_POINT('Ctrl Pts',(105.5,49.5625,-43.6995308303616));
#8591=CARTESIAN_POINT('Ctrl Pts',(105.5,49.5,-1.29200237310046E-14));
#8592=CARTESIAN_POINT('Ctrl Pts',(105.5,49.4375,43.6995308303615));
#8593=CARTESIAN_POINT('Ctrl Pts',(74.5997654151808,49.375,74.5997654151808));
#8594=CARTESIAN_POINT('Ctrl Pts',(43.6995308303616,49.3125,105.5));
#8595=CARTESIAN_POINT('Ctrl Pts',(1.93800355965069E-14,49.25,105.5));
#8596=CARTESIAN_POINT('Ctrl Pts',(-43.6995308303616,49.1875,105.5));
#8597=CARTESIAN_POINT('Ctrl Pts',(-74.5997654151808,49.125,74.5997654151808));
#8598=CARTESIAN_POINT('Ctrl Pts',(-105.5,49.0625,43.6995308303616));
#8599=CARTESIAN_POINT('Ctrl Pts',(-105.5,49.,0.));
#8600=CARTESIAN_POINT('Ctrl Pts',(-105.5,48.9375,-43.6995308303615));
#8601=CARTESIAN_POINT('Ctrl Pts',(-74.5997654151808,48.875,-74.5997654151808));
#8602=CARTESIAN_POINT('Ctrl Pts',(-43.6995308303615,48.8125,-105.5));
#8603=CARTESIAN_POINT('Ctrl Pts',(-6.46001186550229E-15,48.75,-105.5));
#8604=CARTESIAN_POINT('Ctrl Pts',(43.6995308303615,48.6875,-105.5));
#8605=CARTESIAN_POINT('Ctrl Pts',(74.5997654151808,48.625,-74.5997654151808));
#8606=CARTESIAN_POINT('Ctrl Pts',(105.5,48.5625,-43.6995308303616));
#8607=CARTESIAN_POINT('Ctrl Pts',(105.5,48.5,-1.29200237310046E-14));
#8608=CARTESIAN_POINT('Ctrl Pts',(105.5,48.4375,43.6995308303615));
#8609=CARTESIAN_POINT('Ctrl Pts',(74.5997654151808,48.375,74.5997654151808));
#8610=CARTESIAN_POINT('Ctrl Pts',(43.6995308303616,48.3125,105.5));
#8611=CARTESIAN_POINT('Ctrl Pts',(1.93800355965069E-14,48.25,105.5));
#8612=CARTESIAN_POINT('Ctrl Pts',(-43.6995308303616,48.1875,105.5));
#8613=CARTESIAN_POINT('Ctrl Pts',(-74.5997654151808,48.125,74.5997654151808));
#8614=CARTESIAN_POINT('Ctrl Pts',(-105.5,48.0625,43.6995308303616));
#8615=CARTESIAN_POINT('Ctrl Pts',(-105.5,48.,0.));
#8616=CARTESIAN_POINT('Ctrl Pts',(-105.5,47.9375,-43.6995308303615));
#8617=CARTESIAN_POINT('Ctrl Pts',(-74.5997654151808,47.875,-74.5997654151808));
#8618=CARTESIAN_POINT('Ctrl Pts',(-43.6995308303615,47.8125,-105.5));
#8619=CARTESIAN_POINT('Ctrl Pts',(-6.46001186550229E-15,47.75,-105.5));
#8620=CARTESIAN_POINT('Ctrl Pts',(43.6995308303615,47.6875,-105.5));
#8621=CARTESIAN_POINT('Ctrl Pts',(74.5997654151808,47.625,-74.5997654151808));
#8622=CARTESIAN_POINT('Ctrl Pts',(105.5,47.5625,-43.6995308303616));
#8623=CARTESIAN_POINT('Ctrl Pts',(105.5,47.5,-1.29200237310046E-14));
#8624=CARTESIAN_POINT('Ctrl Pts',(105.5,47.4375,43.6995308303615));
#8625=CARTESIAN_POINT('Ctrl Pts',(74.5997654151808,47.375,74.5997654151808));
#8626=CARTESIAN_POINT('Ctrl Pts',(43.6995308303616,47.3125,105.5));
#8627=CARTESIAN_POINT('Ctrl Pts',(1.93800355965069E-14,47.25,105.5));
#8628=CARTESIAN_POINT('Ctrl Pts',(-43.6995308303616,47.1875,105.5));
#8629=CARTESIAN_POINT('Ctrl Pts',(-74.5997654151808,47.125,74.5997654151808));
#8630=CARTESIAN_POINT('Ctrl Pts',(-105.5,47.0625,43.6995308303616));
#8631=CARTESIAN_POINT('Ctrl Pts',(-105.5,47.,0.));
#8632=CARTESIAN_POINT('Ctrl Pts',(-105.5,46.9375,-43.6995308303615));
#8633=CARTESIAN_POINT('Ctrl Pts',(-74.5997654151808,46.875,-74.5997654151808));
#8634=CARTESIAN_POINT('Ctrl Pts',(-43.6995308303615,46.8125,-105.5));
#8635=CARTESIAN_POINT('Ctrl Pts',(-6.46001186550229E-15,46.75,-105.5));
#8636=CARTESIAN_POINT('Ctrl Pts',(43.6995308303615,46.6875,-105.5));
#8637=CARTESIAN_POINT('Ctrl Pts',(74.5997654151808,46.625,-74.5997654151808));
#8638=CARTESIAN_POINT('Ctrl Pts',(105.5,46.5625,-43.6995308303616));
#8639=CARTESIAN_POINT('Ctrl Pts',(105.5,46.5,-1.29200237310046E-14));
#8640=CARTESIAN_POINT('Ctrl Pts',(105.5,46.4375,43.6995308303615));
#8641=CARTESIAN_POINT('Ctrl Pts',(74.5997654151808,46.375,74.5997654151808));
#8642=CARTESIAN_POINT('Ctrl Pts',(43.6995308303616,46.3125,105.5));
#8643=CARTESIAN_POINT('Ctrl Pts',(1.93800355965069E-14,46.25,105.5));
#8644=CARTESIAN_POINT('Ctrl Pts',(-43.6995308303616,46.1875,105.5));
#8645=CARTESIAN_POINT('Ctrl Pts',(-74.5997654151808,46.125,74.5997654151808));
#8646=CARTESIAN_POINT('Ctrl Pts',(-105.5,46.0625,43.6995308303616));
#8647=CARTESIAN_POINT('Ctrl Pts',(-105.5,46.,0.));
#8648=CARTESIAN_POINT('Ctrl Pts',(-105.5,45.9375,-43.6995308303615));
#8649=CARTESIAN_POINT('Ctrl Pts',(-74.5997654151808,45.875,-74.5997654151808));
#8650=CARTESIAN_POINT('Ctrl Pts',(-43.6995308303615,45.8125,-105.5));
#8651=CARTESIAN_POINT('Ctrl Pts',(-6.46001186550229E-15,45.75,-105.5));
#8652=CARTESIAN_POINT('Ctrl Pts',(43.6995308303615,45.6875,-105.5));
#8653=CARTESIAN_POINT('Ctrl Pts',(74.5997654151808,45.625,-74.5997654151808));
#8654=CARTESIAN_POINT('Ctrl Pts',(105.5,45.5625,-43.6995308303616));
#8655=CARTESIAN_POINT('Ctrl Pts',(105.5,45.5,-1.29200237310046E-14));
#8656=CARTESIAN_POINT('Ctrl Pts',(105.5,45.4375,43.6995308303615));
#8657=CARTESIAN_POINT('Ctrl Pts',(74.5997654151808,45.375,74.5997654151808));
#8658=CARTESIAN_POINT('Ctrl Pts',(43.6995308303616,45.3125,105.5));
#8659=CARTESIAN_POINT('Ctrl Pts',(1.93800355965069E-14,45.25,105.5));
#8660=CARTESIAN_POINT('Ctrl Pts',(-43.6995308303616,45.1875,105.5));
#8661=CARTESIAN_POINT('Ctrl Pts',(-74.5997654151808,45.125,74.5997654151808));
#8662=CARTESIAN_POINT('Ctrl Pts',(-105.5,45.0625,43.6995308303616));
#8663=CARTESIAN_POINT('Ctrl Pts',(-105.5,45.,0.));
#8664=CARTESIAN_POINT('Ctrl Pts',(-105.5,44.9375,-43.6995308303615));
#8665=CARTESIAN_POINT('Ctrl Pts',(-74.5997654151808,44.875,-74.5997654151808));
#8666=CARTESIAN_POINT('Ctrl Pts',(-43.6995308303615,44.8125,-105.5));
#8667=CARTESIAN_POINT('Ctrl Pts',(-6.46001186550229E-15,44.75,-105.5));
#8668=CARTESIAN_POINT('Ctrl Pts',(43.6995308303615,44.6875,-105.5));
#8669=CARTESIAN_POINT('Ctrl Pts',(74.5997654151808,44.625,-74.5997654151808));
#8670=CARTESIAN_POINT('Ctrl Pts',(105.5,44.5625,-43.6995308303616));
#8671=CARTESIAN_POINT('Ctrl Pts',(105.5,44.5,-1.29200237310046E-14));
#8672=CARTESIAN_POINT('Ctrl Pts',(105.5,44.4375,43.6995308303615));
#8673=CARTESIAN_POINT('Ctrl Pts',(74.5997654151808,44.375,74.5997654151808));
#8674=CARTESIAN_POINT('Ctrl Pts',(43.6995308303616,44.3125,105.5));
#8675=CARTESIAN_POINT('Ctrl Pts',(1.93800355965069E-14,44.25,105.5));
#8676=CARTESIAN_POINT('Ctrl Pts',(-43.6995308303616,44.1875,105.5));
#8677=CARTESIAN_POINT('Ctrl Pts',(-74.5997654151808,44.125,74.5997654151808));
#8678=CARTESIAN_POINT('Ctrl Pts',(-105.5,44.0625,43.6995308303616));
#8679=CARTESIAN_POINT('Ctrl Pts',(-105.5,44.,0.));
#8680=CARTESIAN_POINT('Ctrl Pts',(-105.5,43.9375,-43.6995308303615));
#8681=CARTESIAN_POINT('Ctrl Pts',(-74.5997654151808,43.875,-74.5997654151808));
#8682=CARTESIAN_POINT('Ctrl Pts',(-43.6995308303615,43.8125,-105.5));
#8683=CARTESIAN_POINT('Ctrl Pts',(-6.46001186550229E-15,43.75,-105.5));
#8684=CARTESIAN_POINT('Ctrl Pts',(43.6995308303615,43.6875,-105.5));
#8685=CARTESIAN_POINT('Ctrl Pts',(74.5997654151808,43.625,-74.5997654151808));
#8686=CARTESIAN_POINT('Ctrl Pts',(105.5,43.5625,-43.6995308303616));
#8687=CARTESIAN_POINT('Ctrl Pts',(105.5,43.5,-1.29200237310046E-14));
#8688=CARTESIAN_POINT('Ctrl Pts',(105.5,43.4375,43.6995308303615));
#8689=CARTESIAN_POINT('Ctrl Pts',(74.5997654151808,43.375,74.5997654151808));
#8690=CARTESIAN_POINT('Ctrl Pts',(43.6995308303616,43.3125,105.5));
#8691=CARTESIAN_POINT('Ctrl Pts',(1.93800355965069E-14,43.25,105.5));
#8692=CARTESIAN_POINT('Ctrl Pts',(-43.6995308303616,43.1875,105.5));
#8693=CARTESIAN_POINT('Ctrl Pts',(-74.5997654151808,43.125,74.5997654151808));
#8694=CARTESIAN_POINT('Ctrl Pts',(-105.5,43.0625,43.6995308303616));
#8695=CARTESIAN_POINT('Ctrl Pts',(-105.5,43.,0.));
#8696=CARTESIAN_POINT('Ctrl Pts',(-105.5,42.9375,-43.6995308303615));
#8697=CARTESIAN_POINT('Ctrl Pts',(-74.5997654151808,42.875,-74.5997654151808));
#8698=CARTESIAN_POINT('Ctrl Pts',(-43.6995308303615,42.8125,-105.5));
#8699=CARTESIAN_POINT('Ctrl Pts',(-6.46001186550229E-15,42.75,-105.5));
#8700=CARTESIAN_POINT('Ctrl Pts',(43.6995308303615,42.6875,-105.5));
#8701=CARTESIAN_POINT('Ctrl Pts',(74.5997654151808,42.625,-74.5997654151808));
#8702=CARTESIAN_POINT('Ctrl Pts',(105.5,42.5625,-43.6995308303616));
#8703=CARTESIAN_POINT('Ctrl Pts',(105.5,42.5,-1.29200237310046E-14));
#8704=CARTESIAN_POINT('Ctrl Pts',(105.5,42.4375,43.6995308303615));
#8705=CARTESIAN_POINT('Ctrl Pts',(74.5997654151808,42.375,74.5997654151808));
#8706=CARTESIAN_POINT('Ctrl Pts',(43.6995308303616,42.3125,105.5));
#8707=CARTESIAN_POINT('Ctrl Pts',(1.93800355965069E-14,42.25,105.5));
#8708=CARTESIAN_POINT('Ctrl Pts',(-43.6995308303616,42.1875,105.5));
#8709=CARTESIAN_POINT('Ctrl Pts',(-74.5997654151808,42.125,74.5997654151808));
#8710=CARTESIAN_POINT('Ctrl Pts',(-105.5,42.0625,43.6995308303616));
#8711=CARTESIAN_POINT('Ctrl Pts',(-105.5,42.,0.));
#8712=CARTESIAN_POINT('Ctrl Pts',(-105.5,41.9375,-43.6995308303615));
#8713=CARTESIAN_POINT('Ctrl Pts',(-74.5997654151808,41.875,-74.5997654151808));
#8714=CARTESIAN_POINT('Ctrl Pts',(-43.6995308303615,41.8125,-105.5));
#8715=CARTESIAN_POINT('Ctrl Pts',(-6.46001186550229E-15,41.75,-105.5));
#8716=CARTESIAN_POINT('Ctrl Pts',(43.6995308303615,41.6875,-105.5));
#8717=CARTESIAN_POINT('Ctrl Pts',(74.5997654151808,41.625,-74.5997654151808));
#8718=CARTESIAN_POINT('Ctrl Pts',(105.5,41.5625,-43.6995308303616));
#8719=CARTESIAN_POINT('Ctrl Pts',(105.5,41.5,-1.29200237310046E-14));
#8720=CARTESIAN_POINT('Ctrl Pts',(105.5,41.4375,43.6995308303615));
#8721=CARTESIAN_POINT('Ctrl Pts',(74.5997654151808,41.375,74.5997654151808));
#8722=CARTESIAN_POINT('Ctrl Pts',(43.6995308303616,41.3125,105.5));
#8723=CARTESIAN_POINT('Ctrl Pts',(1.93800355965069E-14,41.25,105.5));
#8724=CARTESIAN_POINT('Ctrl Pts',(-43.6995308303616,41.1875,105.5));
#8725=CARTESIAN_POINT('Ctrl Pts',(-74.5997654151808,41.125,74.5997654151808));
#8726=CARTESIAN_POINT('Ctrl Pts',(-105.5,41.0625,43.6995308303616));
#8727=CARTESIAN_POINT('Ctrl Pts',(-105.5,41.,0.));
#8728=CARTESIAN_POINT('Ctrl Pts',(-105.5,40.9375,-43.6995308303615));
#8729=CARTESIAN_POINT('Ctrl Pts',(-74.5997654151808,40.875,-74.5997654151808));
#8730=CARTESIAN_POINT('Ctrl Pts',(-43.6995308303615,40.8125,-105.5));
#8731=CARTESIAN_POINT('Ctrl Pts',(-6.46001186550229E-15,40.75,-105.5));
#8732=CARTESIAN_POINT('Ctrl Pts',(43.6995308303615,40.6875,-105.5));
#8733=CARTESIAN_POINT('Ctrl Pts',(74.5997654151808,40.625,-74.5997654151808));
#8734=CARTESIAN_POINT('Ctrl Pts',(105.5,40.5625,-43.6995308303616));
#8735=CARTESIAN_POINT('Ctrl Pts',(105.5,40.5,-1.29200237310046E-14));
#8736=CARTESIAN_POINT('Ctrl Pts',(105.5,40.4375,43.6995308303615));
#8737=CARTESIAN_POINT('Ctrl Pts',(74.5997654151808,40.375,74.5997654151808));
#8738=CARTESIAN_POINT('Ctrl Pts',(43.6995308303616,40.3125,105.5));
#8739=CARTESIAN_POINT('Ctrl Pts',(1.93800355965069E-14,40.25,105.5));
#8740=CARTESIAN_POINT('Ctrl Pts',(-43.6995308303616,40.1875,105.5));
#8741=CARTESIAN_POINT('Ctrl Pts',(-74.5997654151808,40.125,74.5997654151808));
#8742=CARTESIAN_POINT('Ctrl Pts',(-105.5,40.0625,43.6995308303616));
#8743=CARTESIAN_POINT('Ctrl Pts',(-105.5,40.,0.));
#8744=CARTESIAN_POINT('Ctrl Pts',(-105.5,39.9375,-43.6995308303615));
#8745=CARTESIAN_POINT('Ctrl Pts',(-74.5997654151808,39.875,-74.5997654151808));
#8746=CARTESIAN_POINT('Ctrl Pts',(-43.6995308303615,39.8125,-105.5));
#8747=CARTESIAN_POINT('Ctrl Pts',(-6.46001186550229E-15,39.75,-105.5));
#8748=CARTESIAN_POINT('Ctrl Pts',(43.6995308303615,39.6875,-105.5));
#8749=CARTESIAN_POINT('Ctrl Pts',(74.5997654151808,39.625,-74.5997654151808));
#8750=CARTESIAN_POINT('Ctrl Pts',(105.5,39.5625,-43.6995308303616));
#8751=CARTESIAN_POINT('Ctrl Pts',(105.5,39.5,-1.29200237310046E-14));
#8752=CARTESIAN_POINT('Ctrl Pts',(105.5,39.4375,43.6995308303615));
#8753=CARTESIAN_POINT('Ctrl Pts',(74.5997654151808,39.375,74.5997654151808));
#8754=CARTESIAN_POINT('Ctrl Pts',(43.6995308303616,39.3125,105.5));
#8755=CARTESIAN_POINT('Ctrl Pts',(1.93800355965069E-14,39.25,105.5));
#8756=CARTESIAN_POINT('Ctrl Pts',(-43.6995308303616,39.1875,105.5));
#8757=CARTESIAN_POINT('Ctrl Pts',(-74.5997654151808,39.125,74.5997654151808));
#8758=CARTESIAN_POINT('Ctrl Pts',(-105.5,39.0625,43.6995308303616));
#8759=CARTESIAN_POINT('Ctrl Pts',(-105.5,39.,0.));
#8760=CARTESIAN_POINT('Ctrl Pts',(-105.5,38.9375,-43.6995308303615));
#8761=CARTESIAN_POINT('Ctrl Pts',(-74.5997654151808,38.875,-74.5997654151808));
#8762=CARTESIAN_POINT('Ctrl Pts',(-43.6995308303615,38.8125,-105.5));
#8763=CARTESIAN_POINT('Ctrl Pts',(-6.46001186550229E-15,38.75,-105.5));
#8764=CARTESIAN_POINT('Ctrl Pts',(43.6995308303615,38.6875,-105.5));
#8765=CARTESIAN_POINT('Ctrl Pts',(74.5997654151808,38.625,-74.5997654151808));
#8766=CARTESIAN_POINT('Ctrl Pts',(105.5,38.5625,-43.6995308303616));
#8767=CARTESIAN_POINT('Ctrl Pts',(105.5,38.5,-1.29200237310046E-14));
#8768=CARTESIAN_POINT('Ctrl Pts',(105.5,38.4375,43.6995308303615));
#8769=CARTESIAN_POINT('Ctrl Pts',(74.5997654151808,38.375,74.5997654151808));
#8770=CARTESIAN_POINT('Ctrl Pts',(43.6995308303616,38.3125,105.5));
#8771=CARTESIAN_POINT('Ctrl Pts',(1.93800355965069E-14,38.25,105.5));
#8772=CARTESIAN_POINT('Ctrl Pts',(-43.6995308303616,38.1875,105.5));
#8773=CARTESIAN_POINT('Ctrl Pts',(-74.5997654151808,38.125,74.5997654151808));
#8774=CARTESIAN_POINT('Ctrl Pts',(-105.5,38.0625,43.6995308303616));
#8775=CARTESIAN_POINT('Ctrl Pts',(-105.5,38.,0.));
#8776=CARTESIAN_POINT('Ctrl Pts',(-105.5,37.9375,-43.6995308303615));
#8777=CARTESIAN_POINT('Ctrl Pts',(-74.5997654151808,37.875,-74.5997654151808));
#8778=CARTESIAN_POINT('Ctrl Pts',(-43.6995308303615,37.8125,-105.5));
#8779=CARTESIAN_POINT('Ctrl Pts',(-6.46001186550229E-15,37.75,-105.5));
#8780=CARTESIAN_POINT('Ctrl Pts',(43.6995308303615,37.6875,-105.5));
#8781=CARTESIAN_POINT('Ctrl Pts',(74.5997654151808,37.625,-74.5997654151808));
#8782=CARTESIAN_POINT('Ctrl Pts',(105.5,37.5625,-43.6995308303616));
#8783=CARTESIAN_POINT('Ctrl Pts',(105.5,37.5,-1.29200237310046E-14));
#8784=CARTESIAN_POINT('Ctrl Pts',(105.5,37.4375,43.6995308303615));
#8785=CARTESIAN_POINT('Ctrl Pts',(74.5997654151808,37.375,74.5997654151808));
#8786=CARTESIAN_POINT('Ctrl Pts',(43.6995308303616,37.3125,105.5));
#8787=CARTESIAN_POINT('Ctrl Pts',(1.93800355965069E-14,37.25,105.5));
#8788=CARTESIAN_POINT('Ctrl Pts',(-43.6995308303616,37.1875,105.5));
#8789=CARTESIAN_POINT('Ctrl Pts',(-74.5997654151808,37.125,74.5997654151808));
#8790=CARTESIAN_POINT('Ctrl Pts',(-105.5,37.0625,43.6995308303616));
#8791=CARTESIAN_POINT('Ctrl Pts',(-105.5,37.,0.));
#8792=CARTESIAN_POINT('Ctrl Pts',(-105.5,36.9375,-43.6995308303615));
#8793=CARTESIAN_POINT('Ctrl Pts',(-74.5997654151808,36.875,-74.5997654151808));
#8794=CARTESIAN_POINT('Ctrl Pts',(-43.6995308303615,36.8125,-105.5));
#8795=CARTESIAN_POINT('Ctrl Pts',(-6.46001186550229E-15,36.75,-105.5));
#8796=CARTESIAN_POINT('Ctrl Pts',(43.6995308303615,36.6875,-105.5));
#8797=CARTESIAN_POINT('Ctrl Pts',(74.5997654151808,36.625,-74.5997654151808));
#8798=CARTESIAN_POINT('Ctrl Pts',(105.5,36.5625,-43.6995308303616));
#8799=CARTESIAN_POINT('Ctrl Pts',(105.5,36.5,-1.29200237310046E-14));
#8800=CARTESIAN_POINT('Ctrl Pts',(105.5,36.4375,43.6995308303615));
#8801=CARTESIAN_POINT('Ctrl Pts',(74.5997654151808,36.375,74.5997654151808));
#8802=CARTESIAN_POINT('Ctrl Pts',(43.6995308303616,36.3125,105.5));
#8803=CARTESIAN_POINT('Ctrl Pts',(1.93800355965069E-14,36.25,105.5));
#8804=CARTESIAN_POINT('Ctrl Pts',(-43.6995308303616,36.1875,105.5));
#8805=CARTESIAN_POINT('Ctrl Pts',(-74.5997654151808,36.125,74.5997654151808));
#8806=CARTESIAN_POINT('Ctrl Pts',(-105.5,36.0625,43.6995308303616));
#8807=CARTESIAN_POINT('Ctrl Pts',(-105.5,36.,0.));
#8808=CARTESIAN_POINT('Ctrl Pts',(-105.5,35.9375,-43.6995308303615));
#8809=CARTESIAN_POINT('Ctrl Pts',(-74.5997654151808,35.875,-74.5997654151808));
#8810=CARTESIAN_POINT('Ctrl Pts',(-43.6995308303615,35.8125,-105.5));
#8811=CARTESIAN_POINT('Ctrl Pts',(-6.46001186550229E-15,35.75,-105.5));
#8812=CARTESIAN_POINT('Ctrl Pts',(43.6995308303615,35.6875,-105.5));
#8813=CARTESIAN_POINT('Ctrl Pts',(74.5997654151808,35.625,-74.5997654151808));
#8814=CARTESIAN_POINT('Ctrl Pts',(105.5,35.5625,-43.6995308303616));
#8815=CARTESIAN_POINT('Ctrl Pts',(105.5,35.5,-1.29200237310046E-14));
#8816=CARTESIAN_POINT('Ctrl Pts',(105.5,35.4375,43.6995308303615));
#8817=CARTESIAN_POINT('Ctrl Pts',(74.5997654151808,35.375,74.5997654151808));
#8818=CARTESIAN_POINT('Ctrl Pts',(43.6995308303616,35.3125,105.5));
#8819=CARTESIAN_POINT('Ctrl Pts',(1.93800355965069E-14,35.25,105.5));
#8820=CARTESIAN_POINT('Ctrl Pts',(-43.6995308303616,35.1875,105.5));
#8821=CARTESIAN_POINT('Ctrl Pts',(-74.5997654151808,35.125,74.5997654151808));
#8822=CARTESIAN_POINT('Ctrl Pts',(-105.5,35.0625,43.6995308303616));
#8823=CARTESIAN_POINT('Ctrl Pts',(-105.5,35.,0.));
#8824=CARTESIAN_POINT('Ctrl Pts',(-105.5,34.9375,-43.6995308303615));
#8825=CARTESIAN_POINT('Ctrl Pts',(-74.5997654151808,34.875,-74.5997654151808));
#8826=CARTESIAN_POINT('Ctrl Pts',(-43.6995308303615,34.8125,-105.5));
#8827=CARTESIAN_POINT('Ctrl Pts',(-6.46001186550229E-15,34.75,-105.5));
#8828=CARTESIAN_POINT('Ctrl Pts',(43.6995308303615,34.6875,-105.5));
#8829=CARTESIAN_POINT('Ctrl Pts',(74.5997654151808,34.625,-74.5997654151808));
#8830=CARTESIAN_POINT('Ctrl Pts',(105.5,34.5625,-43.6995308303616));
#8831=CARTESIAN_POINT('Ctrl Pts',(105.5,34.5,-1.29200237310046E-14));
#8832=CARTESIAN_POINT('Ctrl Pts',(105.5,34.4375,43.6995308303615));
#8833=CARTESIAN_POINT('Ctrl Pts',(74.5997654151808,34.375,74.5997654151808));
#8834=CARTESIAN_POINT('Ctrl Pts',(43.6995308303616,34.3125,105.5));
#8835=CARTESIAN_POINT('Ctrl Pts',(1.93800355965069E-14,34.25,105.5));
#8836=CARTESIAN_POINT('Ctrl Pts',(-43.6995308303616,34.1875,105.5));
#8837=CARTESIAN_POINT('Ctrl Pts',(-74.5997654151808,34.125,74.5997654151808));
#8838=CARTESIAN_POINT('Ctrl Pts',(-105.5,34.0625,43.6995308303616));
#8839=CARTESIAN_POINT('Ctrl Pts',(-105.5,34.,0.));
#8840=CARTESIAN_POINT('Ctrl Pts',(-105.5,33.9375,-43.6995308303615));
#8841=CARTESIAN_POINT('Ctrl Pts',(-74.5997654151808,33.875,-74.5997654151808));
#8842=CARTESIAN_POINT('Ctrl Pts',(-43.6995308303615,33.8125,-105.5));
#8843=CARTESIAN_POINT('Ctrl Pts',(-6.46001186550229E-15,33.75,-105.5));
#8844=CARTESIAN_POINT('Ctrl Pts',(43.6995308303615,33.6875,-105.5));
#8845=CARTESIAN_POINT('Ctrl Pts',(74.5997654151808,33.625,-74.5997654151808));
#8846=CARTESIAN_POINT('Ctrl Pts',(105.5,33.5625,-43.6995308303616));
#8847=CARTESIAN_POINT('Ctrl Pts',(105.5,33.5,-1.29200237310046E-14));
#8848=CARTESIAN_POINT('Ctrl Pts',(105.5,33.4375,43.6995308303615));
#8849=CARTESIAN_POINT('Ctrl Pts',(74.5997654151808,33.375,74.5997654151808));
#8850=CARTESIAN_POINT('Ctrl Pts',(43.6995308303616,33.3125,105.5));
#8851=CARTESIAN_POINT('Ctrl Pts',(1.93800355965069E-14,33.25,105.5));
#8852=CARTESIAN_POINT('Ctrl Pts',(-43.6995308303616,33.1875,105.5));
#8853=CARTESIAN_POINT('Ctrl Pts',(-74.5997654151808,33.125,74.5997654151808));
#8854=CARTESIAN_POINT('Ctrl Pts',(-105.5,33.0625,43.6995308303616));
#8855=CARTESIAN_POINT('Ctrl Pts',(-105.5,33.,0.));
#8856=CARTESIAN_POINT('Ctrl Pts',(-105.5,32.9375,-43.6995308303615));
#8857=CARTESIAN_POINT('Ctrl Pts',(-74.5997654151808,32.875,-74.5997654151808));
#8858=CARTESIAN_POINT('Ctrl Pts',(-43.6995308303615,32.8125,-105.5));
#8859=CARTESIAN_POINT('Ctrl Pts',(-6.46001186550229E-15,32.75,-105.5));
#8860=CARTESIAN_POINT('Ctrl Pts',(43.6995308303615,32.6875,-105.5));
#8861=CARTESIAN_POINT('Ctrl Pts',(74.5997654151808,32.625,-74.5997654151808));
#8862=CARTESIAN_POINT('Ctrl Pts',(105.5,32.5625,-43.6995308303616));
#8863=CARTESIAN_POINT('Ctrl Pts',(105.5,32.5,-1.29200237310046E-14));
#8864=CARTESIAN_POINT('Ctrl Pts',(105.5,32.4375,43.6995308303615));
#8865=CARTESIAN_POINT('Ctrl Pts',(74.5997654151808,32.375,74.5997654151808));
#8866=CARTESIAN_POINT('Ctrl Pts',(43.6995308303616,32.3125,105.5));
#8867=CARTESIAN_POINT('Ctrl Pts',(1.93800355965069E-14,32.25,105.5));
#8868=CARTESIAN_POINT('Ctrl Pts',(-43.6995308303616,32.1875,105.5));
#8869=CARTESIAN_POINT('Ctrl Pts',(-74.5997654151808,32.125,74.5997654151808));
#8870=CARTESIAN_POINT('Ctrl Pts',(-105.5,32.0625,43.6995308303616));
#8871=CARTESIAN_POINT('Ctrl Pts',(-105.5,32.,0.));
#8872=CARTESIAN_POINT('Ctrl Pts',(-105.5,31.9375,-43.6995308303615));
#8873=CARTESIAN_POINT('Ctrl Pts',(-74.5997654151808,31.875,-74.5997654151808));
#8874=CARTESIAN_POINT('Ctrl Pts',(-43.6995308303615,31.8125,-105.5));
#8875=CARTESIAN_POINT('Ctrl Pts',(-6.46001186550229E-15,31.75,-105.5));
#8876=CARTESIAN_POINT('Ctrl Pts',(43.6995308303615,31.6875,-105.5));
#8877=CARTESIAN_POINT('Ctrl Pts',(74.5997654151808,31.625,-74.5997654151808));
#8878=CARTESIAN_POINT('Ctrl Pts',(105.5,31.5625,-43.6995308303616));
#8879=CARTESIAN_POINT('Ctrl Pts',(105.5,31.5,-1.29200237310046E-14));
#8880=CARTESIAN_POINT('Ctrl Pts',(105.5,31.4375,43.6995308303615));
#8881=CARTESIAN_POINT('Ctrl Pts',(74.5997654151808,31.375,74.5997654151808));
#8882=CARTESIAN_POINT('Ctrl Pts',(43.6995308303616,31.3125,105.5));
#8883=CARTESIAN_POINT('Ctrl Pts',(1.93800355965069E-14,31.25,105.5));
#8884=CARTESIAN_POINT('Ctrl Pts',(-43.6995308303616,31.1875,105.5));
#8885=CARTESIAN_POINT('Ctrl Pts',(-74.5997654151808,31.125,74.5997654151808));
#8886=CARTESIAN_POINT('Ctrl Pts',(-105.5,31.0625,43.6995308303616));
#8887=CARTESIAN_POINT('Ctrl Pts',(-105.5,31.,0.));
#8888=CARTESIAN_POINT('Ctrl Pts',(-105.5,30.9375,-43.6995308303615));
#8889=CARTESIAN_POINT('Ctrl Pts',(-74.5997654151808,30.875,-74.5997654151808));
#8890=CARTESIAN_POINT('Ctrl Pts',(-43.6995308303615,30.8125,-105.5));
#8891=CARTESIAN_POINT('Ctrl Pts',(-6.46001186550229E-15,30.75,-105.5));
#8892=CARTESIAN_POINT('Ctrl Pts',(43.6995308303615,30.6875,-105.5));
#8893=CARTESIAN_POINT('Ctrl Pts',(74.5997654151808,30.625,-74.5997654151808));
#8894=CARTESIAN_POINT('Ctrl Pts',(105.5,30.5625,-43.6995308303616));
#8895=CARTESIAN_POINT('Ctrl Pts',(105.5,30.5,-1.29200237310046E-14));
#8896=CARTESIAN_POINT('Ctrl Pts',(105.5,30.4375,43.6995308303615));
#8897=CARTESIAN_POINT('Ctrl Pts',(74.5997654151808,30.375,74.5997654151808));
#8898=CARTESIAN_POINT('Ctrl Pts',(43.6995308303616,30.3125,105.5));
#8899=CARTESIAN_POINT('Ctrl Pts',(1.93800355965069E-14,30.25,105.5));
#8900=CARTESIAN_POINT('Ctrl Pts',(-43.6995308303616,30.1875,105.5));
#8901=CARTESIAN_POINT('Ctrl Pts',(-74.5997654151808,30.125,74.5997654151808));
#8902=CARTESIAN_POINT('Ctrl Pts',(-105.5,30.0625,43.6995308303616));
#8903=CARTESIAN_POINT('Ctrl Pts',(-105.5,30.,0.));
#8904=CARTESIAN_POINT('Ctrl Pts',(-105.5,29.9375,-43.6995308303615));
#8905=CARTESIAN_POINT('Ctrl Pts',(-74.5997654151808,29.875,-74.5997654151808));
#8906=CARTESIAN_POINT('Ctrl Pts',(-43.6995308303615,29.8125,-105.5));
#8907=CARTESIAN_POINT('Ctrl Pts',(-6.46001186550229E-15,29.75,-105.5));
#8908=CARTESIAN_POINT('Ctrl Pts',(43.6995308303615,29.6875,-105.5));
#8909=CARTESIAN_POINT('Ctrl Pts',(74.5997654151808,29.625,-74.5997654151808));
#8910=CARTESIAN_POINT('Ctrl Pts',(105.5,29.5625,-43.6995308303616));
#8911=CARTESIAN_POINT('Ctrl Pts',(105.5,29.5,-1.29200237310046E-14));
#8912=CARTESIAN_POINT('Ctrl Pts',(105.5,29.4375,43.6995308303615));
#8913=CARTESIAN_POINT('Ctrl Pts',(74.5997654151808,29.375,74.5997654151808));
#8914=CARTESIAN_POINT('Ctrl Pts',(43.6995308303616,29.3125,105.5));
#8915=CARTESIAN_POINT('Ctrl Pts',(1.93800355965069E-14,29.25,105.5));
#8916=CARTESIAN_POINT('Ctrl Pts',(-43.6995308303616,29.1875,105.5));
#8917=CARTESIAN_POINT('Ctrl Pts',(-74.5997654151808,29.125,74.5997654151808));
#8918=CARTESIAN_POINT('Ctrl Pts',(-105.5,29.0625,43.6995308303616));
#8919=CARTESIAN_POINT('Ctrl Pts',(-105.5,29.,0.));
#8920=CARTESIAN_POINT('Ctrl Pts',(-105.5,28.9375,-43.6995308303615));
#8921=CARTESIAN_POINT('Ctrl Pts',(-74.5997654151808,28.875,-74.5997654151808));
#8922=CARTESIAN_POINT('Ctrl Pts',(-43.6995308303615,28.8125,-105.5));
#8923=CARTESIAN_POINT('Ctrl Pts',(-6.46001186550229E-15,28.75,-105.5));
#8924=CARTESIAN_POINT('Ctrl Pts',(43.6995308303615,28.6875,-105.5));
#8925=CARTESIAN_POINT('Ctrl Pts',(74.5997654151808,28.625,-74.5997654151808));
#8926=CARTESIAN_POINT('Ctrl Pts',(105.5,28.5625,-43.6995308303616));
#8927=CARTESIAN_POINT('Ctrl Pts',(105.5,28.5,-1.29200237310046E-14));
#8928=CARTESIAN_POINT('Ctrl Pts',(105.5,28.4375,43.6995308303615));
#8929=CARTESIAN_POINT('Ctrl Pts',(74.5997654151808,28.375,74.5997654151808));
#8930=CARTESIAN_POINT('Ctrl Pts',(43.6995308303616,28.3125,105.5));
#8931=CARTESIAN_POINT('Ctrl Pts',(1.93800355965069E-14,28.25,105.5));
#8932=CARTESIAN_POINT('Ctrl Pts',(-43.6995308303616,28.1875,105.5));
#8933=CARTESIAN_POINT('Ctrl Pts',(-74.5997654151808,28.125,74.5997654151808));
#8934=CARTESIAN_POINT('Ctrl Pts',(-105.5,28.0625,43.6995308303616));
#8935=CARTESIAN_POINT('Ctrl Pts',(-105.5,28.,0.));
#8936=CARTESIAN_POINT('Ctrl Pts',(-105.5,27.9375,-43.6995308303615));
#8937=CARTESIAN_POINT('Ctrl Pts',(-74.5997654151808,27.875,-74.5997654151808));
#8938=CARTESIAN_POINT('Ctrl Pts',(-43.6995308303615,27.8125,-105.5));
#8939=CARTESIAN_POINT('Ctrl Pts',(-6.46001186550229E-15,27.75,-105.5));
#8940=CARTESIAN_POINT('Ctrl Pts',(43.6995308303615,27.6875,-105.5));
#8941=CARTESIAN_POINT('Ctrl Pts',(74.5997654151808,27.625,-74.5997654151808));
#8942=CARTESIAN_POINT('Ctrl Pts',(105.5,27.5625,-43.6995308303616));
#8943=CARTESIAN_POINT('Ctrl Pts',(105.5,27.5,-1.29200237310046E-14));
#8944=CARTESIAN_POINT('Ctrl Pts',(105.5,27.4375,43.6995308303615));
#8945=CARTESIAN_POINT('Ctrl Pts',(74.5997654151808,27.375,74.5997654151808));
#8946=CARTESIAN_POINT('Ctrl Pts',(43.6995308303616,27.3125,105.5));
#8947=CARTESIAN_POINT('Ctrl Pts',(1.93800355965069E-14,27.25,105.5));
#8948=CARTESIAN_POINT('Ctrl Pts',(-43.6995308303616,27.1875,105.5));
#8949=CARTESIAN_POINT('Ctrl Pts',(-74.5997654151808,27.125,74.5997654151808));
#8950=CARTESIAN_POINT('Ctrl Pts',(-105.5,27.0625,43.6995308303616));
#8951=CARTESIAN_POINT('Ctrl Pts',(-105.5,27.,0.));
#8952=CARTESIAN_POINT('Ctrl Pts',(-105.5,26.9375,-43.6995308303615));
#8953=CARTESIAN_POINT('Ctrl Pts',(-74.5997654151808,26.875,-74.5997654151808));
#8954=CARTESIAN_POINT('Ctrl Pts',(-43.6995308303615,26.8125,-105.5));
#8955=CARTESIAN_POINT('Ctrl Pts',(-6.46001186550229E-15,26.75,-105.5));
#8956=CARTESIAN_POINT('Ctrl Pts',(43.6995308303615,26.6875,-105.5));
#8957=CARTESIAN_POINT('Ctrl Pts',(74.5997654151808,26.625,-74.5997654151808));
#8958=CARTESIAN_POINT('Ctrl Pts',(105.5,26.5625,-43.6995308303616));
#8959=CARTESIAN_POINT('Ctrl Pts',(105.5,26.5,-1.29200237310046E-14));
#8960=CARTESIAN_POINT('Ctrl Pts',(105.5,26.4375,43.6995308303615));
#8961=CARTESIAN_POINT('Ctrl Pts',(74.5997654151808,26.375,74.5997654151808));
#8962=CARTESIAN_POINT('Ctrl Pts',(43.6995308303616,26.3125,105.5));
#8963=CARTESIAN_POINT('Ctrl Pts',(1.93800355965069E-14,26.25,105.5));
#8964=CARTESIAN_POINT('Ctrl Pts',(-43.6995308303616,26.1875,105.5));
#8965=CARTESIAN_POINT('Ctrl Pts',(-74.5997654151808,26.125,74.5997654151808));
#8966=CARTESIAN_POINT('Ctrl Pts',(-105.5,26.0625,43.6995308303616));
#8967=CARTESIAN_POINT('Ctrl Pts',(-105.5,26.,0.));
#8968=CARTESIAN_POINT('Ctrl Pts',(-105.5,25.9375,-43.6995308303615));
#8969=CARTESIAN_POINT('Ctrl Pts',(-74.5997654151808,25.875,-74.5997654151808));
#8970=CARTESIAN_POINT('Ctrl Pts',(-43.6995308303615,25.8125,-105.5));
#8971=CARTESIAN_POINT('Ctrl Pts',(-6.46001186550229E-15,25.75,-105.5));
#8972=CARTESIAN_POINT('Ctrl Pts',(43.6995308303615,25.6875,-105.5));
#8973=CARTESIAN_POINT('Ctrl Pts',(74.5997654151808,25.625,-74.5997654151808));
#8974=CARTESIAN_POINT('Ctrl Pts',(105.5,25.5625,-43.6995308303616));
#8975=CARTESIAN_POINT('Ctrl Pts',(105.5,25.5,-1.29200237310046E-14));
#8976=CARTESIAN_POINT('Ctrl Pts',(105.5,25.4375,43.6995308303615));
#8977=CARTESIAN_POINT('Ctrl Pts',(74.5997654151808,25.375,74.5997654151808));
#8978=CARTESIAN_POINT('Ctrl Pts',(43.6995308303616,25.3125,105.5));
#8979=CARTESIAN_POINT('Ctrl Pts',(1.93800355965069E-14,25.25,105.5));
#8980=CARTESIAN_POINT('Ctrl Pts',(-43.6995308303616,25.1875,105.5));
#8981=CARTESIAN_POINT('Ctrl Pts',(-74.5997654151808,25.125,74.5997654151808));
#8982=CARTESIAN_POINT('Ctrl Pts',(-105.5,25.0625,43.6995308303616));
#8983=CARTESIAN_POINT('Ctrl Pts',(-105.5,25.,0.));
#8984=CARTESIAN_POINT('Ctrl Pts',(-105.5,24.9375,-43.6995308303615));
#8985=CARTESIAN_POINT('Ctrl Pts',(-74.5997654151808,24.875,-74.5997654151808));
#8986=CARTESIAN_POINT('Ctrl Pts',(-43.6995308303615,24.8125,-105.5));
#8987=CARTESIAN_POINT('Ctrl Pts',(-6.46001186550229E-15,24.75,-105.5));
#8988=CARTESIAN_POINT('Ctrl Pts',(43.6995308303615,24.6875,-105.5));
#8989=CARTESIAN_POINT('Ctrl Pts',(74.5997654151808,24.625,-74.5997654151808));
#8990=CARTESIAN_POINT('Ctrl Pts',(105.5,24.5625,-43.6995308303616));
#8991=CARTESIAN_POINT('Ctrl Pts',(105.5,24.5,-1.29200237310046E-14));
#8992=CARTESIAN_POINT('Ctrl Pts',(105.5,24.4375,43.6995308303615));
#8993=CARTESIAN_POINT('Ctrl Pts',(74.5997654151808,24.375,74.5997654151808));
#8994=CARTESIAN_POINT('Ctrl Pts',(43.6995308303616,24.3125,105.5));
#8995=CARTESIAN_POINT('Ctrl Pts',(1.93800355965069E-14,24.25,105.5));
#8996=CARTESIAN_POINT('Ctrl Pts',(-43.6995308303616,24.1875,105.5));
#8997=CARTESIAN_POINT('Ctrl Pts',(-74.5997654151808,24.125,74.5997654151808));
#8998=CARTESIAN_POINT('Ctrl Pts',(-105.5,24.0625,43.6995308303616));
#8999=CARTESIAN_POINT('Ctrl Pts',(-105.5,24.,0.));
#9000=CARTESIAN_POINT('Ctrl Pts',(-105.5,23.9375,-43.6995308303615));
#9001=CARTESIAN_POINT('Ctrl Pts',(-74.5997654151808,23.875,-74.5997654151808));
#9002=CARTESIAN_POINT('Ctrl Pts',(-43.6995308303615,23.8125,-105.5));
#9003=CARTESIAN_POINT('Ctrl Pts',(-6.46001186550229E-15,23.75,-105.5));
#9004=CARTESIAN_POINT('Ctrl Pts',(43.6995308303615,23.6875,-105.5));
#9005=CARTESIAN_POINT('Ctrl Pts',(74.5997654151808,23.625,-74.5997654151808));
#9006=CARTESIAN_POINT('Ctrl Pts',(105.5,23.5625,-43.6995308303616));
#9007=CARTESIAN_POINT('Ctrl Pts',(105.5,23.5,-1.29200237310046E-14));
#9008=CARTESIAN_POINT('Ctrl Pts',(105.5,23.4375,43.6995308303615));
#9009=CARTESIAN_POINT('Ctrl Pts',(74.5997654151808,23.375,74.5997654151808));
#9010=CARTESIAN_POINT('Ctrl Pts',(43.6995308303616,23.3125,105.5));
#9011=CARTESIAN_POINT('Ctrl Pts',(1.93800355965069E-14,23.25,105.5));
#9012=CARTESIAN_POINT('Ctrl Pts',(-43.6995308303616,23.1875,105.5));
#9013=CARTESIAN_POINT('Ctrl Pts',(-74.5997654151808,23.125,74.5997654151808));
#9014=CARTESIAN_POINT('Ctrl Pts',(-105.5,23.0625,43.6995308303616));
#9015=CARTESIAN_POINT('Ctrl Pts',(-105.5,23.,0.));
#9016=CARTESIAN_POINT('Ctrl Pts',(-105.5,22.9375,-43.6995308303615));
#9017=CARTESIAN_POINT('Ctrl Pts',(-74.5997654151808,22.875,-74.5997654151808));
#9018=CARTESIAN_POINT('Ctrl Pts',(-43.6995308303615,22.8125,-105.5));
#9019=CARTESIAN_POINT('Ctrl Pts',(-6.46001186550229E-15,22.75,-105.5));
#9020=CARTESIAN_POINT('Ctrl Pts',(43.6995308303615,22.6875,-105.5));
#9021=CARTESIAN_POINT('Ctrl Pts',(74.5997654151808,22.625,-74.5997654151808));
#9022=CARTESIAN_POINT('Ctrl Pts',(105.5,22.5625,-43.6995308303616));
#9023=CARTESIAN_POINT('Ctrl Pts',(105.5,22.5,-1.29200237310046E-14));
#9024=CARTESIAN_POINT('Ctrl Pts',(105.5,22.4375,43.6995308303615));
#9025=CARTESIAN_POINT('Ctrl Pts',(74.5997654151808,22.375,74.5997654151808));
#9026=CARTESIAN_POINT('Ctrl Pts',(43.6995308303616,22.3125,105.5));
#9027=CARTESIAN_POINT('Ctrl Pts',(1.93800355965069E-14,22.25,105.5));
#9028=CARTESIAN_POINT('Ctrl Pts',(-43.6995308303616,22.1875,105.5));
#9029=CARTESIAN_POINT('Ctrl Pts',(-74.5997654151808,22.125,74.5997654151808));
#9030=CARTESIAN_POINT('Ctrl Pts',(-105.5,22.0625,43.6995308303616));
#9031=CARTESIAN_POINT('Ctrl Pts',(-105.5,22.,0.));
#9032=CARTESIAN_POINT('Ctrl Pts',(-105.5,21.9375,-43.6995308303615));
#9033=CARTESIAN_POINT('Ctrl Pts',(-74.5997654151808,21.875,-74.5997654151808));
#9034=CARTESIAN_POINT('Ctrl Pts',(-43.6995308303615,21.8125,-105.5));
#9035=CARTESIAN_POINT('Ctrl Pts',(-6.46001186550229E-15,21.75,-105.5));
#9036=CARTESIAN_POINT('Ctrl Pts',(43.6995308303615,21.6875,-105.5));
#9037=CARTESIAN_POINT('Ctrl Pts',(74.5997654151808,21.625,-74.5997654151808));
#9038=CARTESIAN_POINT('Ctrl Pts',(105.5,21.5625,-43.6995308303616));
#9039=CARTESIAN_POINT('Ctrl Pts',(105.5,21.5,-1.29200237310046E-14));
#9040=CARTESIAN_POINT('Ctrl Pts',(105.5,21.4375,43.6995308303615));
#9041=CARTESIAN_POINT('Ctrl Pts',(74.5997654151808,21.375,74.5997654151808));
#9042=CARTESIAN_POINT('Ctrl Pts',(43.6995308303616,21.3125,105.5));
#9043=CARTESIAN_POINT('Ctrl Pts',(1.93800355965069E-14,21.25,105.5));
#9044=CARTESIAN_POINT('Ctrl Pts',(-43.6995308303616,21.1875,105.5));
#9045=CARTESIAN_POINT('Ctrl Pts',(-74.5997654151808,21.125,74.5997654151808));
#9046=CARTESIAN_POINT('Ctrl Pts',(-105.5,21.0625,43.6995308303616));
#9047=CARTESIAN_POINT('Ctrl Pts',(-105.5,21.,0.));
#9048=CARTESIAN_POINT('Ctrl Pts',(-105.5,20.9375,-43.6995308303615));
#9049=CARTESIAN_POINT('Ctrl Pts',(-74.5997654151808,20.875,-74.5997654151808));
#9050=CARTESIAN_POINT('Ctrl Pts',(-43.6995308303615,20.8125,-105.5));
#9051=CARTESIAN_POINT('Ctrl Pts',(-6.46001186550229E-15,20.75,-105.5));
#9052=CARTESIAN_POINT('Ctrl Pts',(43.6995308303615,20.6875,-105.5));
#9053=CARTESIAN_POINT('Ctrl Pts',(74.5997654151808,20.625,-74.5997654151808));
#9054=CARTESIAN_POINT('Ctrl Pts',(105.5,20.5625,-43.6995308303616));
#9055=CARTESIAN_POINT('Ctrl Pts',(105.5,20.5,-1.29200237310046E-14));
#9056=CARTESIAN_POINT('Ctrl Pts',(105.5,20.4375,43.6995308303615));
#9057=CARTESIAN_POINT('Ctrl Pts',(74.5997654151808,20.375,74.5997654151808));
#9058=CARTESIAN_POINT('Ctrl Pts',(43.6995308303616,20.3125,105.5));
#9059=CARTESIAN_POINT('Ctrl Pts',(1.93800355965069E-14,20.25,105.5));
#9060=CARTESIAN_POINT('Ctrl Pts',(-43.6995308303616,20.1875,105.5));
#9061=CARTESIAN_POINT('Ctrl Pts',(-74.5997654151808,20.125,74.5997654151808));
#9062=CARTESIAN_POINT('Ctrl Pts',(-105.5,20.0625,43.6995308303616));
#9063=CARTESIAN_POINT('Ctrl Pts',(-105.5,20.,0.));
#9064=CARTESIAN_POINT('Ctrl Pts',(-105.5,19.9375,-43.6995308303615));
#9065=CARTESIAN_POINT('Ctrl Pts',(-74.5997654151808,19.875,-74.5997654151808));
#9066=CARTESIAN_POINT('Ctrl Pts',(-43.6995308303615,19.8125,-105.5));
#9067=CARTESIAN_POINT('Ctrl Pts',(-6.46001186550229E-15,19.75,-105.5));
#9068=CARTESIAN_POINT('Ctrl Pts',(43.6995308303615,19.6875,-105.5));
#9069=CARTESIAN_POINT('Ctrl Pts',(74.5997654151808,19.625,-74.5997654151808));
#9070=CARTESIAN_POINT('Ctrl Pts',(105.5,19.5625,-43.6995308303616));
#9071=CARTESIAN_POINT('Ctrl Pts',(105.5,19.5,-1.29200237310046E-14));
#9072=CARTESIAN_POINT('Ctrl Pts',(105.5,19.4375,43.6995308303615));
#9073=CARTESIAN_POINT('Ctrl Pts',(74.5997654151808,19.375,74.5997654151808));
#9074=CARTESIAN_POINT('Ctrl Pts',(43.6995308303616,19.3125,105.5));
#9075=CARTESIAN_POINT('Ctrl Pts',(1.93800355965069E-14,19.25,105.5));
#9076=CARTESIAN_POINT('Ctrl Pts',(-43.6995308303616,19.1875,105.5));
#9077=CARTESIAN_POINT('Ctrl Pts',(-74.5997654151808,19.125,74.5997654151808));
#9078=CARTESIAN_POINT('Ctrl Pts',(-105.5,19.0625,43.6995308303616));
#9079=CARTESIAN_POINT('Ctrl Pts',(-105.5,19.,0.));
#9080=CARTESIAN_POINT('Ctrl Pts',(-105.5,18.9375,-43.6995308303615));
#9081=CARTESIAN_POINT('Ctrl Pts',(-74.5997654151808,18.875,-74.5997654151808));
#9082=CARTESIAN_POINT('Ctrl Pts',(-43.6995308303615,18.8125,-105.5));
#9083=CARTESIAN_POINT('Ctrl Pts',(-6.46001186550229E-15,18.75,-105.5));
#9084=CARTESIAN_POINT('Ctrl Pts',(43.6995308303615,18.6875,-105.5));
#9085=CARTESIAN_POINT('Ctrl Pts',(74.5997654151808,18.625,-74.5997654151808));
#9086=CARTESIAN_POINT('Ctrl Pts',(105.5,18.5625,-43.6995308303616));
#9087=CARTESIAN_POINT('Ctrl Pts',(105.5,18.5,-1.29200237310046E-14));
#9088=CARTESIAN_POINT('Ctrl Pts',(105.5,18.4375,43.6995308303615));
#9089=CARTESIAN_POINT('Ctrl Pts',(74.5997654151808,18.375,74.5997654151808));
#9090=CARTESIAN_POINT('Ctrl Pts',(43.6995308303616,18.3125,105.5));
#9091=CARTESIAN_POINT('Ctrl Pts',(1.93800355965069E-14,18.25,105.5));
#9092=CARTESIAN_POINT('Ctrl Pts',(-43.6995308303616,18.1875,105.5));
#9093=CARTESIAN_POINT('Ctrl Pts',(-74.5997654151808,18.125,74.5997654151808));
#9094=CARTESIAN_POINT('Ctrl Pts',(-105.5,18.0625,43.6995308303616));
#9095=CARTESIAN_POINT('Ctrl Pts',(-105.5,18.,0.));
#9096=CARTESIAN_POINT('Ctrl Pts',(-105.5,17.9375,-43.6995308303615));
#9097=CARTESIAN_POINT('Ctrl Pts',(-74.5997654151808,17.875,-74.5997654151808));
#9098=CARTESIAN_POINT('Ctrl Pts',(-43.6995308303615,17.8125,-105.5));
#9099=CARTESIAN_POINT('Ctrl Pts',(-6.46001186550229E-15,17.75,-105.5));
#9100=CARTESIAN_POINT('Ctrl Pts',(43.6995308303615,17.6875,-105.5));
#9101=CARTESIAN_POINT('Ctrl Pts',(74.5997654151808,17.625,-74.5997654151808));
#9102=CARTESIAN_POINT('Ctrl Pts',(105.5,17.5625,-43.6995308303616));
#9103=CARTESIAN_POINT('Ctrl Pts',(105.5,17.5,-1.29200237310046E-14));
#9104=CARTESIAN_POINT('Ctrl Pts',(105.5,17.4375,43.6995308303615));
#9105=CARTESIAN_POINT('Ctrl Pts',(74.5997654151808,17.375,74.5997654151808));
#9106=CARTESIAN_POINT('Ctrl Pts',(43.6995308303616,17.3125,105.5));
#9107=CARTESIAN_POINT('Ctrl Pts',(1.93800355965069E-14,17.25,105.5));
#9108=CARTESIAN_POINT('Ctrl Pts',(-43.6995308303616,17.1875,105.5));
#9109=CARTESIAN_POINT('Ctrl Pts',(-74.5997654151808,17.125,74.5997654151808));
#9110=CARTESIAN_POINT('Ctrl Pts',(-105.5,17.0625,43.6995308303616));
#9111=CARTESIAN_POINT('Ctrl Pts',(-105.5,17.,0.));
#9112=CARTESIAN_POINT('Ctrl Pts',(-105.5,16.9375,-43.6995308303615));
#9113=CARTESIAN_POINT('Ctrl Pts',(-74.5997654151808,16.875,-74.5997654151808));
#9114=CARTESIAN_POINT('Ctrl Pts',(-43.6995308303615,16.8125,-105.5));
#9115=CARTESIAN_POINT('Ctrl Pts',(-6.46001186550229E-15,16.75,-105.5));
#9116=CARTESIAN_POINT('Ctrl Pts',(43.6995308303615,16.6875,-105.5));
#9117=CARTESIAN_POINT('Ctrl Pts',(74.5997654151808,16.625,-74.5997654151808));
#9118=CARTESIAN_POINT('Ctrl Pts',(105.5,16.5625,-43.6995308303616));
#9119=CARTESIAN_POINT('Ctrl Pts',(105.5,16.5,-1.29200237310046E-14));
#9120=CARTESIAN_POINT('Ctrl Pts',(105.5,16.4375,43.6995308303615));
#9121=CARTESIAN_POINT('Ctrl Pts',(74.5997654151808,16.375,74.5997654151808));
#9122=CARTESIAN_POINT('Ctrl Pts',(43.6995308303616,16.3125,105.5));
#9123=CARTESIAN_POINT('Ctrl Pts',(1.93800355965069E-14,16.25,105.5));
#9124=CARTESIAN_POINT('Ctrl Pts',(-43.6995308303616,16.1875,105.5));
#9125=CARTESIAN_POINT('Ctrl Pts',(-74.5997654151808,16.125,74.5997654151808));
#9126=CARTESIAN_POINT('Ctrl Pts',(-105.5,16.0625,43.6995308303616));
#9127=CARTESIAN_POINT('Ctrl Pts',(-105.5,16.,0.));
#9128=CARTESIAN_POINT('Ctrl Pts',(-105.5,15.9375,-43.6995308303615));
#9129=CARTESIAN_POINT('Ctrl Pts',(-74.5997654151808,15.875,-74.5997654151808));
#9130=CARTESIAN_POINT('Ctrl Pts',(-43.6995308303615,15.8125,-105.5));
#9131=CARTESIAN_POINT('Ctrl Pts',(-6.46001186550229E-15,15.75,-105.5));
#9132=CARTESIAN_POINT('Ctrl Pts',(43.6995308303615,15.6875,-105.5));
#9133=CARTESIAN_POINT('Ctrl Pts',(74.5997654151808,15.625,-74.5997654151808));
#9134=CARTESIAN_POINT('Ctrl Pts',(105.5,15.5625,-43.6995308303616));
#9135=CARTESIAN_POINT('Ctrl Pts',(105.5,15.5,-1.29200237310046E-14));
#9136=CARTESIAN_POINT('Ctrl Pts',(105.5,15.4375,43.6995308303615));
#9137=CARTESIAN_POINT('Ctrl Pts',(74.5997654151808,15.375,74.5997654151808));
#9138=CARTESIAN_POINT('Ctrl Pts',(43.6995308303616,15.3125,105.5));
#9139=CARTESIAN_POINT('Ctrl Pts',(1.93800355965069E-14,15.25,105.5));
#9140=CARTESIAN_POINT('Ctrl Pts',(-43.6995308303616,15.1875,105.5));
#9141=CARTESIAN_POINT('Ctrl Pts',(-74.5997654151808,15.125,74.5997654151808));
#9142=CARTESIAN_POINT('Ctrl Pts',(-105.5,15.0625,43.6995308303616));
#9143=CARTESIAN_POINT('Ctrl Pts',(-105.5,15.,0.));
#9144=CARTESIAN_POINT('Ctrl Pts',(-105.5,14.9375,-43.6995308303615));
#9145=CARTESIAN_POINT('Ctrl Pts',(-74.5997654151808,14.875,-74.5997654151808));
#9146=CARTESIAN_POINT('Ctrl Pts',(-43.6995308303615,14.8125,-105.5));
#9147=CARTESIAN_POINT('Ctrl Pts',(-6.46001186550229E-15,14.75,-105.5));
#9148=CARTESIAN_POINT('Ctrl Pts',(43.6995308303615,14.6875,-105.5));
#9149=CARTESIAN_POINT('Ctrl Pts',(74.5997654151808,14.625,-74.5997654151808));
#9150=CARTESIAN_POINT('Ctrl Pts',(105.5,14.5625,-43.6995308303616));
#9151=CARTESIAN_POINT('Ctrl Pts',(105.5,14.5,-1.29200237310046E-14));
#9152=CARTESIAN_POINT('Ctrl Pts',(105.5,14.4375,43.6995308303615));
#9153=CARTESIAN_POINT('Ctrl Pts',(74.5997654151808,14.375,74.5997654151808));
#9154=CARTESIAN_POINT('Ctrl Pts',(43.6995308303616,14.3125,105.5));
#9155=CARTESIAN_POINT('Ctrl Pts',(1.93800355965069E-14,14.25,105.5));
#9156=CARTESIAN_POINT('Ctrl Pts',(-43.6995308303616,14.1875,105.5));
#9157=CARTESIAN_POINT('Ctrl Pts',(-74.5997654151808,14.125,74.5997654151808));
#9158=CARTESIAN_POINT('Ctrl Pts',(-105.5,14.0625,43.6995308303616));
#9159=CARTESIAN_POINT('Ctrl Pts',(-105.5,14.,0.));
#9160=CARTESIAN_POINT('Ctrl Pts',(-105.5,13.9375,-43.6995308303615));
#9161=CARTESIAN_POINT('Ctrl Pts',(-74.5997654151808,13.875,-74.5997654151808));
#9162=CARTESIAN_POINT('Ctrl Pts',(-43.6995308303615,13.8125,-105.5));
#9163=CARTESIAN_POINT('Ctrl Pts',(-6.46001186550229E-15,13.75,-105.5));
#9164=CARTESIAN_POINT('Ctrl Pts',(43.6995308303615,13.6875,-105.5));
#9165=CARTESIAN_POINT('Ctrl Pts',(74.5997654151808,13.625,-74.5997654151808));
#9166=CARTESIAN_POINT('Ctrl Pts',(105.5,13.5625,-43.6995308303616));
#9167=CARTESIAN_POINT('Ctrl Pts',(105.5,13.5,-1.29200237310046E-14));
#9168=CARTESIAN_POINT('Ctrl Pts',(105.5,13.4375,43.6995308303615));
#9169=CARTESIAN_POINT('Ctrl Pts',(74.5997654151808,13.375,74.5997654151808));
#9170=CARTESIAN_POINT('Ctrl Pts',(43.6995308303616,13.3125,105.5));
#9171=CARTESIAN_POINT('Ctrl Pts',(1.93800355965069E-14,13.25,105.5));
#9172=CARTESIAN_POINT('Ctrl Pts',(-43.6995308303616,13.1875,105.5));
#9173=CARTESIAN_POINT('Ctrl Pts',(-74.5997654151808,13.125,74.5997654151808));
#9174=CARTESIAN_POINT('Ctrl Pts',(-105.5,13.0625,43.6995308303616));
#9175=CARTESIAN_POINT('Ctrl Pts',(-105.5,13.,0.));
#9176=CARTESIAN_POINT('Ctrl Pts',(-105.5,12.9375,-43.6995308303615));
#9177=CARTESIAN_POINT('Ctrl Pts',(-74.5997654151808,12.875,-74.5997654151808));
#9178=CARTESIAN_POINT('Ctrl Pts',(-43.6995308303615,12.8125,-105.5));
#9179=CARTESIAN_POINT('Ctrl Pts',(-6.46001186550229E-15,12.75,-105.5));
#9180=CARTESIAN_POINT('Ctrl Pts',(43.6995308303615,12.6875,-105.5));
#9181=CARTESIAN_POINT('Ctrl Pts',(74.5997654151808,12.625,-74.5997654151808));
#9182=CARTESIAN_POINT('Ctrl Pts',(105.5,12.5625,-43.6995308303616));
#9183=CARTESIAN_POINT('Ctrl Pts',(105.5,12.5,-1.29200237310046E-14));
#9184=CARTESIAN_POINT('Ctrl Pts',(105.5,12.4375,43.6995308303615));
#9185=CARTESIAN_POINT('Ctrl Pts',(74.5997654151808,12.375,74.5997654151808));
#9186=CARTESIAN_POINT('Ctrl Pts',(43.6995308303616,12.3125,105.5));
#9187=CARTESIAN_POINT('Ctrl Pts',(1.93800355965069E-14,12.25,105.5));
#9188=CARTESIAN_POINT('Ctrl Pts',(-43.6995308303616,12.1875,105.5));
#9189=CARTESIAN_POINT('Ctrl Pts',(-74.5997654151808,12.125,74.5997654151808));
#9190=CARTESIAN_POINT('Ctrl Pts',(-105.5,12.0625,43.6995308303616));
#9191=CARTESIAN_POINT('Ctrl Pts',(-105.5,12.,0.));
#9192=CARTESIAN_POINT('Ctrl Pts',(-105.5,11.9375,-43.6995308303615));
#9193=CARTESIAN_POINT('Ctrl Pts',(-74.5997654151808,11.875,-74.5997654151808));
#9194=CARTESIAN_POINT('Ctrl Pts',(-43.6995308303615,11.8125,-105.5));
#9195=CARTESIAN_POINT('Ctrl Pts',(-6.46001186550229E-15,11.75,-105.5));
#9196=CARTESIAN_POINT('Ctrl Pts',(43.6995308303615,11.6875,-105.5));
#9197=CARTESIAN_POINT('Ctrl Pts',(74.5997654151808,11.625,-74.5997654151808));
#9198=CARTESIAN_POINT('Ctrl Pts',(105.5,11.5625,-43.6995308303616));
#9199=CARTESIAN_POINT('Ctrl Pts',(105.5,11.5,-1.29200237310046E-14));
#9200=CARTESIAN_POINT('Ctrl Pts',(105.5,11.4375,43.6995308303615));
#9201=CARTESIAN_POINT('Ctrl Pts',(74.5997654151808,11.375,74.5997654151808));
#9202=CARTESIAN_POINT('Ctrl Pts',(43.6995308303616,11.3125,105.5));
#9203=CARTESIAN_POINT('Ctrl Pts',(1.93800355965069E-14,11.25,105.5));
#9204=CARTESIAN_POINT('Ctrl Pts',(-43.6995308303616,11.1875,105.5));
#9205=CARTESIAN_POINT('Ctrl Pts',(-74.5997654151808,11.125,74.5997654151808));
#9206=CARTESIAN_POINT('Ctrl Pts',(-105.5,11.0625,43.6995308303616));
#9207=CARTESIAN_POINT('Ctrl Pts',(-105.5,11.,0.));
#9208=CARTESIAN_POINT('Ctrl Pts',(-105.5,10.9375,-43.6995308303615));
#9209=CARTESIAN_POINT('Ctrl Pts',(-74.5997654151808,10.875,-74.5997654151808));
#9210=CARTESIAN_POINT('Ctrl Pts',(-43.6995308303615,10.8125,-105.5));
#9211=CARTESIAN_POINT('Ctrl Pts',(-6.46001186550229E-15,10.75,-105.5));
#9212=CARTESIAN_POINT('Ctrl Pts',(43.6995308303615,10.6875,-105.5));
#9213=CARTESIAN_POINT('Ctrl Pts',(74.5997654151808,10.625,-74.5997654151808));
#9214=CARTESIAN_POINT('Ctrl Pts',(105.5,10.5625,-43.6995308303616));
#9215=CARTESIAN_POINT('Ctrl Pts',(105.5,10.5,-1.29200237310046E-14));
#9216=CARTESIAN_POINT('Ctrl Pts',(105.5,10.4375,43.6995308303615));
#9217=CARTESIAN_POINT('Ctrl Pts',(74.5997654151808,10.375,74.5997654151808));
#9218=CARTESIAN_POINT('Ctrl Pts',(43.6995308303616,10.3125,105.5));
#9219=CARTESIAN_POINT('Ctrl Pts',(1.93800355965069E-14,10.25,105.5));
#9220=CARTESIAN_POINT('Ctrl Pts',(-43.6995308303616,10.1875,105.5));
#9221=CARTESIAN_POINT('Ctrl Pts',(-74.5997654151808,10.125,74.5997654151808));
#9222=CARTESIAN_POINT('Ctrl Pts',(-105.5,10.0625,43.6995308303616));
#9223=CARTESIAN_POINT('Ctrl Pts',(-105.5,9.99999999999999,0.));
#9224=CARTESIAN_POINT('Ctrl Pts',(-105.5,9.93749999999999,-43.6995308303615));
#9225=CARTESIAN_POINT('Ctrl Pts',(-74.5997654151808,9.87499999999999,-74.5997654151808));
#9226=CARTESIAN_POINT('Ctrl Pts',(-43.6995308303615,9.81249999999999,-105.5));
#9227=CARTESIAN_POINT('Ctrl Pts',(-6.46001186550229E-15,9.74999999999999,
-105.5));
#9228=CARTESIAN_POINT('Ctrl Pts',(43.6995308303615,9.68749999999999,-105.5));
#9229=CARTESIAN_POINT('Ctrl Pts',(74.5997654151808,9.62499999999999,-74.5997654151808));
#9230=CARTESIAN_POINT('Ctrl Pts',(105.5,9.56249999999999,-43.6995308303616));
#9231=CARTESIAN_POINT('Ctrl Pts',(105.5,9.49999999999999,-1.29200237310046E-14));
#9232=CARTESIAN_POINT('Ctrl Pts',(105.5,9.43749999999999,43.6995308303615));
#9233=CARTESIAN_POINT('Ctrl Pts',(74.5997654151808,9.37499999999999,74.5997654151808));
#9234=CARTESIAN_POINT('Ctrl Pts',(43.6995308303616,9.31249999999999,105.5));
#9235=CARTESIAN_POINT('Ctrl Pts',(1.93800355965069E-14,9.24999999999999,
105.5));
#9236=CARTESIAN_POINT('Ctrl Pts',(-43.6995308303616,9.18749999999999,105.5));
#9237=CARTESIAN_POINT('Ctrl Pts',(-74.5997654151808,9.12499999999999,74.5997654151808));
#9238=CARTESIAN_POINT('Ctrl Pts',(-105.5,9.06249999999999,43.6995308303616));
#9239=CARTESIAN_POINT('Ctrl Pts',(-105.5,8.99999999999999,0.));
#9240=CARTESIAN_POINT('Ctrl Pts',(-105.5,8.93749999999999,-43.6995308303615));
#9241=CARTESIAN_POINT('Ctrl Pts',(-74.5997654151808,8.87499999999999,-74.5997654151808));
#9242=CARTESIAN_POINT('Ctrl Pts',(-43.6995308303615,8.81249999999999,-105.5));
#9243=CARTESIAN_POINT('Ctrl Pts',(-6.46001186550229E-15,8.74999999999999,
-105.5));
#9244=CARTESIAN_POINT('Ctrl Pts',(43.6995308303615,8.68749999999999,-105.5));
#9245=CARTESIAN_POINT('Ctrl Pts',(74.5997654151808,8.62499999999999,-74.5997654151808));
#9246=CARTESIAN_POINT('Ctrl Pts',(105.5,8.56249999999999,-43.6995308303616));
#9247=CARTESIAN_POINT('Ctrl Pts',(105.5,8.49999999999999,-1.29200237310046E-14));
#9248=CARTESIAN_POINT('Ctrl Pts',(105.5,8.43749999999999,43.6995308303615));
#9249=CARTESIAN_POINT('Ctrl Pts',(74.5997654151808,8.37499999999999,74.5997654151808));
#9250=CARTESIAN_POINT('Ctrl Pts',(43.6995308303616,8.31249999999999,105.5));
#9251=CARTESIAN_POINT('Ctrl Pts',(1.93800355965069E-14,8.24999999999999,
105.5));
#9252=CARTESIAN_POINT('Ctrl Pts',(-43.6995308303616,8.18749999999999,105.5));
#9253=CARTESIAN_POINT('Ctrl Pts',(-74.5997654151808,8.12499999999999,74.5997654151808));
#9254=CARTESIAN_POINT('Ctrl Pts',(-105.5,8.06249999999999,43.6995308303616));
#9255=CARTESIAN_POINT('Ctrl Pts',(-105.5,7.99999999999999,0.));
#9256=CARTESIAN_POINT('Ctrl Pts',(-105.5,7.93749999999999,-43.6995308303615));
#9257=CARTESIAN_POINT('Ctrl Pts',(-74.5997654151808,7.87499999999999,-74.5997654151808));
#9258=CARTESIAN_POINT('Ctrl Pts',(-43.6995308303615,7.81249999999999,-105.5));
#9259=CARTESIAN_POINT('Ctrl Pts',(-6.46001186550229E-15,7.74999999999999,
-105.5));
#9260=CARTESIAN_POINT('Ctrl Pts',(43.6995308303615,7.68749999999999,-105.5));
#9261=CARTESIAN_POINT('Ctrl Pts',(74.5997654151808,7.62499999999999,-74.5997654151808));
#9262=CARTESIAN_POINT('Ctrl Pts',(105.5,7.56249999999999,-43.6995308303616));
#9263=CARTESIAN_POINT('Ctrl Pts',(105.5,7.49999999999999,-1.29200237310046E-14));
#9264=CARTESIAN_POINT('Ctrl Pts',(105.5,7.43749999999999,43.6995308303615));
#9265=CARTESIAN_POINT('Ctrl Pts',(74.5997654151808,7.37499999999999,74.5997654151808));
#9266=CARTESIAN_POINT('Ctrl Pts',(43.6995308303616,7.31249999999999,105.5));
#9267=CARTESIAN_POINT('Ctrl Pts',(1.93800355965069E-14,7.24999999999999,
105.5));
#9268=CARTESIAN_POINT('Ctrl Pts',(-43.6995308303616,7.18749999999999,105.5));
#9269=CARTESIAN_POINT('Ctrl Pts',(-74.5997654151808,7.12499999999999,74.5997654151808));
#9270=CARTESIAN_POINT('Ctrl Pts',(-105.5,7.06249999999998,43.6995308303616));
#9271=CARTESIAN_POINT('Ctrl Pts',(-105.5,6.99999999999998,0.));
#9272=CARTESIAN_POINT('Ctrl Pts',(-105.5,6.93749999999999,-43.6995308303615));
#9273=CARTESIAN_POINT('Ctrl Pts',(-74.5997654151808,6.87499999999999,-74.5997654151808));
#9274=CARTESIAN_POINT('Ctrl Pts',(-43.6995308303615,6.81249999999999,-105.5));
#9275=CARTESIAN_POINT('Ctrl Pts',(-6.46001186550229E-15,6.74999999999998,
-105.5));
#9276=CARTESIAN_POINT('Ctrl Pts',(43.6995308303615,6.68749999999998,-105.5));
#9277=CARTESIAN_POINT('Ctrl Pts',(74.5997654151808,6.62499999999999,-74.5997654151808));
#9278=CARTESIAN_POINT('Ctrl Pts',(105.5,6.56249999999998,-43.6995308303616));
#9279=CARTESIAN_POINT('Ctrl Pts',(105.5,6.49999999999998,-1.29200237310046E-14));
#9280=CARTESIAN_POINT('Ctrl Pts',(105.5,6.43749999999998,43.6995308303615));
#9281=CARTESIAN_POINT('Ctrl Pts',(74.5997654151808,6.37499999999998,74.5997654151808));
#9282=CARTESIAN_POINT('Ctrl Pts',(43.6995308303616,6.31249999999999,105.5));
#9283=CARTESIAN_POINT('Ctrl Pts',(1.93800355965069E-14,6.24999999999998,
105.5));
#9284=CARTESIAN_POINT('Ctrl Pts',(-43.6995308303616,6.18749999999998,105.5));
#9285=CARTESIAN_POINT('Ctrl Pts',(-74.5997654151808,6.12499999999998,74.5997654151808));
#9286=CARTESIAN_POINT('Ctrl Pts',(-105.5,6.06249999999998,43.6995308303616));
#9287=CARTESIAN_POINT('Ctrl Pts',(-105.5,5.99999999999999,0.));
#9288=CARTESIAN_POINT('Ctrl Pts',(-105.5,5.93749999999999,-43.6995308303615));
#9289=CARTESIAN_POINT('Ctrl Pts',(-74.5997654151808,5.87499999999999,-74.5997654151808));
#9290=CARTESIAN_POINT('Ctrl Pts',(-43.6995308303615,5.81249999999999,-105.5));
#9291=CARTESIAN_POINT('Ctrl Pts',(-6.46001186550229E-15,5.74999999999999,
-105.5));
#9292=CARTESIAN_POINT('Ctrl Pts',(43.6995308303615,5.68749999999999,-105.5));
#9293=CARTESIAN_POINT('Ctrl Pts',(74.5997654151808,5.62499999999999,-74.5997654151808));
#9294=CARTESIAN_POINT('Ctrl Pts',(105.5,5.56249999999999,-43.6995308303616));
#9295=CARTESIAN_POINT('Ctrl Pts',(105.5,5.49999999999999,-1.29200237310046E-14));
#9296=CARTESIAN_POINT('Ctrl Pts',(105.5,5.43749999999999,43.6995308303615));
#9297=CARTESIAN_POINT('Ctrl Pts',(74.5997654151808,5.37499999999999,74.5997654151808));
#9298=CARTESIAN_POINT('Ctrl Pts',(43.6995308303616,5.31249999999999,105.5));
#9299=CARTESIAN_POINT('Ctrl Pts',(1.93800355965069E-14,5.24999999999999,
105.5));
#9300=CARTESIAN_POINT('Ctrl Pts',(-43.6995308303616,5.18749999999999,105.5));
#9301=CARTESIAN_POINT('Ctrl Pts',(-74.5997654151808,5.12499999999999,74.5997654151808));
#9302=CARTESIAN_POINT('Ctrl Pts',(-105.5,5.06249999999999,43.6995308303616));
#9303=CARTESIAN_POINT('Ctrl Pts',(-105.5,4.99999999999999,0.));
#9304=CARTESIAN_POINT('Ctrl Pts',(-105.5,4.93749999999999,-43.6995308303615));
#9305=CARTESIAN_POINT('Ctrl Pts',(-74.5997654151808,4.87499999999999,-74.5997654151808));
#9306=CARTESIAN_POINT('Ctrl Pts',(-43.6995308303615,4.81249999999999,-105.5));
#9307=CARTESIAN_POINT('Ctrl Pts',(-6.46001186550229E-15,4.74999999999999,
-105.5));
#9308=CARTESIAN_POINT('Ctrl Pts',(43.6995308303615,4.68749999999999,-105.5));
#9309=CARTESIAN_POINT('Ctrl Pts',(74.5997654151808,4.62499999999999,-74.5997654151808));
#9310=CARTESIAN_POINT('Ctrl Pts',(105.5,4.56249999999999,-43.6995308303616));
#9311=CARTESIAN_POINT('Ctrl Pts',(105.5,4.49999999999999,-1.29200237310046E-14));
#9312=CARTESIAN_POINT('Ctrl Pts',(105.5,4.43749999999999,43.6995308303615));
#9313=CARTESIAN_POINT('Ctrl Pts',(74.5997654151808,4.37499999999999,74.5997654151808));
#9314=CARTESIAN_POINT('Ctrl Pts',(43.6995308303616,4.31249999999999,105.5));
#9315=CARTESIAN_POINT('Ctrl Pts',(1.93800355965069E-14,4.24999999999999,
105.5));
#9316=CARTESIAN_POINT('Ctrl Pts',(-43.6995308303616,4.18749999999999,105.5));
#9317=CARTESIAN_POINT('Ctrl Pts',(-74.5997654151808,4.12499999999999,74.5997654151808));
#9318=CARTESIAN_POINT('Ctrl Pts',(-105.5,4.06249999999999,43.6995308303616));
#9319=CARTESIAN_POINT('Ctrl Pts',(-105.5,3.99999999999999,0.));
#9320=CARTESIAN_POINT('Ctrl Pts',(-105.5,3.93749999999999,-43.6995308303615));
#9321=CARTESIAN_POINT('Ctrl Pts',(-74.5997654151808,3.87499999999999,-74.5997654151808));
#9322=CARTESIAN_POINT('Ctrl Pts',(-43.6995308303615,3.81249999999999,-105.5));
#9323=CARTESIAN_POINT('Ctrl Pts',(-6.46001186550229E-15,3.74999999999999,
-105.5));
#9324=CARTESIAN_POINT('Ctrl Pts',(43.6995308303615,3.68749999999999,-105.5));
#9325=CARTESIAN_POINT('Ctrl Pts',(74.5997654151808,3.62499999999999,-74.5997654151808));
#9326=CARTESIAN_POINT('Ctrl Pts',(105.5,3.56249999999999,-43.6995308303616));
#9327=CARTESIAN_POINT('Ctrl Pts',(105.5,3.49999999999999,-1.29200237310046E-14));
#9328=CARTESIAN_POINT('Ctrl Pts',(105.5,3.43749999999999,43.6995308303615));
#9329=CARTESIAN_POINT('Ctrl Pts',(74.5997654151808,3.37499999999999,74.5997654151808));
#9330=CARTESIAN_POINT('Ctrl Pts',(43.6995308303616,3.31249999999999,105.5));
#9331=CARTESIAN_POINT('Ctrl Pts',(1.93800355965069E-14,3.24999999999999,
105.5));
#9332=CARTESIAN_POINT('Ctrl Pts',(-43.6995308303616,3.18749999999999,105.5));
#9333=CARTESIAN_POINT('Ctrl Pts',(-74.5997654151808,3.12499999999999,74.5997654151808));
#9334=CARTESIAN_POINT('Ctrl Pts',(-105.5,3.06249999999999,43.6995308303616));
#9335=CARTESIAN_POINT('Ctrl Pts',(-105.5,2.99999999999999,0.));
#9336=CARTESIAN_POINT('Ctrl Pts',(-105.5,2.93749999999999,-43.6995308303615));
#9337=CARTESIAN_POINT('Ctrl Pts',(-74.5997654151808,2.87499999999999,-74.5997654151808));
#9338=CARTESIAN_POINT('Ctrl Pts',(-43.6995308303615,2.81249999999999,-105.5));
#9339=CARTESIAN_POINT('Ctrl Pts',(-6.46001186550229E-15,2.74999999999999,
-105.5));
#9340=CARTESIAN_POINT('Ctrl Pts',(43.6995308303615,2.68749999999999,-105.5));
#9341=CARTESIAN_POINT('Ctrl Pts',(74.5997654151808,2.62499999999999,-74.5997654151808));
#9342=CARTESIAN_POINT('Ctrl Pts',(105.5,2.56249999999999,-43.6995308303616));
#9343=CARTESIAN_POINT('Ctrl Pts',(105.5,2.49999999999999,-1.29200237310046E-14));
#9344=CARTESIAN_POINT('Ctrl Pts',(105.5,2.43749999999999,43.6995308303615));
#9345=CARTESIAN_POINT('Ctrl Pts',(74.5997654151808,2.37499999999999,74.5997654151808));
#9346=CARTESIAN_POINT('Ctrl Pts',(43.6995308303616,2.31249999999999,105.5));
#9347=CARTESIAN_POINT('Ctrl Pts',(1.93800355965069E-14,2.24999999999999,
105.5));
#9348=CARTESIAN_POINT('Ctrl Pts',(-43.6995308303616,2.18749999999999,105.5));
#9349=CARTESIAN_POINT('Ctrl Pts',(-74.5997654151808,2.12499999999999,74.5997654151808));
#9350=CARTESIAN_POINT('Ctrl Pts',(-105.5,2.06249999999999,43.6995308303616));
#9351=CARTESIAN_POINT('Ctrl Pts',(-105.5,1.99999999999999,0.));
#9352=CARTESIAN_POINT('Ctrl Pts',(-105.5,1.93749999999999,-43.6995308303615));
#9353=CARTESIAN_POINT('Ctrl Pts',(-74.5997654151808,1.87499999999999,-74.5997654151808));
#9354=CARTESIAN_POINT('Ctrl Pts',(-43.6995308303615,1.81249999999999,-105.5));
#9355=CARTESIAN_POINT('Ctrl Pts',(-6.46001186550229E-15,1.74999999999999,
-105.5));
#9356=CARTESIAN_POINT('Ctrl Pts',(43.6995308303615,1.68749999999999,-105.5));
#9357=CARTESIAN_POINT('Ctrl Pts',(74.5997654151808,1.62499999999999,-74.5997654151808));
#9358=CARTESIAN_POINT('Ctrl Pts',(105.5,1.56249999999999,-43.6995308303616));
#9359=CARTESIAN_POINT('Ctrl Pts',(105.5,1.49999999999999,-1.29200237310046E-14));
#9360=CARTESIAN_POINT('Ctrl Pts',(105.5,1.43749999999999,43.6995308303615));
#9361=CARTESIAN_POINT('Ctrl Pts',(74.5997654151808,1.37499999999999,74.5997654151808));
#9362=CARTESIAN_POINT('Ctrl Pts',(43.6995308303616,1.31249999999999,105.5));
#9363=CARTESIAN_POINT('Ctrl Pts',(1.93800355965069E-14,1.24999999999999,
105.5));
#9364=CARTESIAN_POINT('Ctrl Pts',(-43.6995308303616,1.18749999999999,105.5));
#9365=CARTESIAN_POINT('Ctrl Pts',(-74.5997654151808,1.12499999999999,74.5997654151808));
#9366=CARTESIAN_POINT('Ctrl Pts',(-105.5,1.06249999999999,43.6995308303616));
#9367=CARTESIAN_POINT('Ctrl Pts',(-105.5,0.999999999999987,0.));
#9368=CARTESIAN_POINT('Ctrl Pts',(-105.5,0.937499999999987,-43.6995308303615));
#9369=CARTESIAN_POINT('Ctrl Pts',(-74.5997654151808,0.874999999999987,-74.5997654151808));
#9370=CARTESIAN_POINT('Ctrl Pts',(-43.6995308303615,0.812499999999987,-105.5));
#9371=CARTESIAN_POINT('Ctrl Pts',(-6.46001186550229E-15,0.749999999999987,
-105.5));
#9372=CARTESIAN_POINT('Ctrl Pts',(43.6995308303615,0.687499999999987,-105.5));
#9373=CARTESIAN_POINT('Ctrl Pts',(74.5997654151808,0.624999999999987,-74.5997654151808));
#9374=CARTESIAN_POINT('Ctrl Pts',(105.5,0.562499999999987,-43.6995308303616));
#9375=CARTESIAN_POINT('Ctrl Pts',(105.5,0.499999999999987,-1.29200237310046E-14));
#9376=CARTESIAN_POINT('Ctrl Pts',(105.5,0.437499999999987,43.6995308303615));
#9377=CARTESIAN_POINT('Ctrl Pts',(74.5997654151808,0.374999999999986,74.5997654151808));
#9378=CARTESIAN_POINT('Ctrl Pts',(43.6995308303616,0.312499999999986,105.5));
#9379=CARTESIAN_POINT('Ctrl Pts',(1.93800355965069E-14,0.249999999999986,
105.5));
#9380=CARTESIAN_POINT('Ctrl Pts',(-43.6995308303616,0.187499999999986,105.5));
#9381=CARTESIAN_POINT('Ctrl Pts',(-74.5997654151808,0.124999999999986,74.5997654151808));
#9382=CARTESIAN_POINT('Ctrl Pts',(-105.5,0.0624999999999862,43.6995308303616));
#9383=CARTESIAN_POINT('Ctrl Pts',(-105.5,-1.38777878078145E-14,0.));
#9384=CARTESIAN_POINT('Ctrl Pts',(104.958734125,49.1875000013656,-1.28537377788739E-14));
#9385=CARTESIAN_POINT('Ctrl Pts',(104.958734125,49.1250000013656,43.4753311640868));
#9386=CARTESIAN_POINT('Ctrl Pts',(74.2170326445434,49.0625000013656,74.2170326445434));
#9387=CARTESIAN_POINT('Ctrl Pts',(43.4753311640869,49.0000000013656,104.958734125));
#9388=CARTESIAN_POINT('Ctrl Pts',(1.92806066683109E-14,48.9375000013656,
104.958734125));
#9389=CARTESIAN_POINT('Ctrl Pts',(-43.4753311640868,48.8750000013656,104.958734125));
#9390=CARTESIAN_POINT('Ctrl Pts',(-74.2170326445434,48.8125000013656,74.2170326445434));
#9391=CARTESIAN_POINT('Ctrl Pts',(-104.958734125,48.7500000013656,43.4753311640869));
#9392=CARTESIAN_POINT('Ctrl Pts',(-104.958734125,48.6875000013656,0.));
#9393=CARTESIAN_POINT('Ctrl Pts',(-104.958734125,48.6250000013656,-43.4753311640868));
#9394=CARTESIAN_POINT('Ctrl Pts',(-74.2170326445434,48.5625000013656,-74.2170326445434));
#9395=CARTESIAN_POINT('Ctrl Pts',(-43.4753311640868,48.5000000013656,-104.958734125));
#9396=CARTESIAN_POINT('Ctrl Pts',(-6.42686888943697E-15,48.4375000013656,
-104.958734125));
#9397=CARTESIAN_POINT('Ctrl Pts',(43.4753311640868,48.3750000013656,-104.958734125));
#9398=CARTESIAN_POINT('Ctrl Pts',(74.2170326445434,48.3125000013656,-74.2170326445434));
#9399=CARTESIAN_POINT('Ctrl Pts',(104.958734125,48.2500000013656,-43.4753311640868));
#9400=CARTESIAN_POINT('Ctrl Pts',(104.958734125,48.1875000013656,-1.28537377788739E-14));
#9401=CARTESIAN_POINT('Origin',(-7.105427357601E-14,49.5625000013656,-6.0924204042587E-14));
#9402=CARTESIAN_POINT('Ctrl Pts',(104.958734125,48.9375000013656,-1.28537377788739E-14));
#9403=CARTESIAN_POINT('Ctrl Pts',(104.958734125,48.8750000013656,43.4753311640868));
#9404=CARTESIAN_POINT('Ctrl Pts',(74.2170326445434,48.8125000013656,74.2170326445434));
#9405=CARTESIAN_POINT('Ctrl Pts',(43.4753311640869,48.7500000013656,104.958734125));
#9406=CARTESIAN_POINT('Ctrl Pts',(1.92806066683109E-14,48.6875000013656,
104.958734125));
#9407=CARTESIAN_POINT('Ctrl Pts',(-43.4753311640868,48.6250000013656,104.958734125));
#9408=CARTESIAN_POINT('Ctrl Pts',(-74.2170326445434,48.5625000013656,74.2170326445434));
#9409=CARTESIAN_POINT('Ctrl Pts',(-104.958734125,48.5000000013656,43.4753311640869));
#9410=CARTESIAN_POINT('Ctrl Pts',(-104.958734125,48.4375000013656,0.));
#9411=CARTESIAN_POINT('Ctrl Pts',(-104.958734125,48.3750000013656,-43.4753311640868));
#9412=CARTESIAN_POINT('Ctrl Pts',(-74.2170326445434,48.3125000013656,-74.2170326445434));
#9413=CARTESIAN_POINT('Ctrl Pts',(-43.4753311640868,48.2500000013656,-104.958734125));
#9414=CARTESIAN_POINT('Ctrl Pts',(-6.42686888943697E-15,48.1875000013656,
-104.958734125));
#9415=CARTESIAN_POINT('Ctrl Pts',(43.4753311640868,48.1250000013656,-104.958734125));
#9416=CARTESIAN_POINT('Ctrl Pts',(74.2170326445434,48.0625000013656,-74.2170326445434));
#9417=CARTESIAN_POINT('Ctrl Pts',(104.958734125,48.0000000013656,-43.4753311640868));
#9418=CARTESIAN_POINT('Ctrl Pts',(104.958734125,47.9375000013656,-1.28537377788739E-14));
#9419=CARTESIAN_POINT('Ctrl Pts',(-105.5,49.1250000027312,0.));
#9420=CARTESIAN_POINT('Ctrl Pts',(-105.5,49.0625000027312,-43.6995308303615));
#9421=CARTESIAN_POINT('Ctrl Pts',(-74.5997654151808,49.0000000027312,-74.5997654151808));
#9422=CARTESIAN_POINT('Ctrl Pts',(-43.6995308303615,48.9375000027312,-105.5));
#9423=CARTESIAN_POINT('Ctrl Pts',(-6.46001186550229E-15,48.8750000027312,
-105.5));
#9424=CARTESIAN_POINT('Ctrl Pts',(43.6995308303615,48.8125000027312,-105.5));
#9425=CARTESIAN_POINT('Ctrl Pts',(74.5997654151808,48.7500000027312,-74.5997654151808));
#9426=CARTESIAN_POINT('Ctrl Pts',(105.5,48.6875000027312,-43.6995308303616));
#9427=CARTESIAN_POINT('Ctrl Pts',(105.5,48.6250000027312,-1.29200237310046E-14));
#9428=CARTESIAN_POINT('Ctrl Pts',(105.5,48.5625000027312,43.6995308303615));
#9429=CARTESIAN_POINT('Ctrl Pts',(74.5997654151808,48.5000000027312,74.5997654151808));
#9430=CARTESIAN_POINT('Ctrl Pts',(43.6995308303616,48.4375000027312,105.5));
#9431=CARTESIAN_POINT('Ctrl Pts',(1.93800355965069E-14,48.3750000027312,
105.5));
#9432=CARTESIAN_POINT('Ctrl Pts',(-43.6995308303616,48.3125000027312,105.5));
#9433=CARTESIAN_POINT('Ctrl Pts',(-74.5997654151808,48.2500000027312,74.5997654151808));
#9434=CARTESIAN_POINT('Ctrl Pts',(-105.5,48.1875000027312,43.6995308303616));
#9435=CARTESIAN_POINT('Ctrl Pts',(-105.5,48.1250000027312,0.));
#9436=CARTESIAN_POINT('Ctrl Pts',(-105.5,48.0625000027312,-43.6995308303615));
#9437=CARTESIAN_POINT('Ctrl Pts',(-74.5997654151808,48.0000000027312,-74.5997654151808));
#9438=CARTESIAN_POINT('Ctrl Pts',(-43.6995308303615,47.9375000027312,-105.5));
#9439=CARTESIAN_POINT('Ctrl Pts',(-6.46001186550229E-15,47.8750000027312,
-105.5));
#9440=CARTESIAN_POINT('Ctrl Pts',(43.6995308303615,47.8125000027312,-105.5));
#9441=CARTESIAN_POINT('Ctrl Pts',(74.5997654151808,47.7500000027312,-74.5997654151808));
#9442=CARTESIAN_POINT('Ctrl Pts',(105.5,47.6875000027312,-43.6995308303616));
#9443=CARTESIAN_POINT('Ctrl Pts',(105.5,47.6250000027312,-1.29200237310046E-14));
#9444=CARTESIAN_POINT('Ctrl Pts',(105.5,47.5625000027312,43.6995308303615));
#9445=CARTESIAN_POINT('Ctrl Pts',(74.5997654151808,47.5000000027312,74.5997654151808));
#9446=CARTESIAN_POINT('Ctrl Pts',(43.6995308303616,47.4375000027312,105.5));
#9447=CARTESIAN_POINT('Ctrl Pts',(1.93800355965069E-14,47.3750000027312,
105.5));
#9448=CARTESIAN_POINT('Ctrl Pts',(-43.6995308303616,47.3125000027312,105.5));
#9449=CARTESIAN_POINT('Ctrl Pts',(-74.5997654151808,47.2500000027312,74.5997654151808));
#9450=CARTESIAN_POINT('Ctrl Pts',(-105.5,47.1875000027312,43.6995308303616));
#9451=CARTESIAN_POINT('Ctrl Pts',(-105.5,47.1250000027312,0.));
#9452=CARTESIAN_POINT('Ctrl Pts',(-105.5,47.0625000027312,-43.6995308303615));
#9453=CARTESIAN_POINT('Ctrl Pts',(-74.5997654151808,47.0000000027312,-74.5997654151808));
#9454=CARTESIAN_POINT('Ctrl Pts',(-43.6995308303615,46.9375000027312,-105.5));
#9455=CARTESIAN_POINT('Ctrl Pts',(-6.46001186550229E-15,46.8750000027312,
-105.5));
#9456=CARTESIAN_POINT('Ctrl Pts',(43.6995308303615,46.8125000027312,-105.5));
#9457=CARTESIAN_POINT('Ctrl Pts',(74.5997654151808,46.7500000027312,-74.5997654151808));
#9458=CARTESIAN_POINT('Ctrl Pts',(105.5,46.6875000027312,-43.6995308303616));
#9459=CARTESIAN_POINT('Ctrl Pts',(105.5,46.6250000027312,-1.29200237310046E-14));
#9460=CARTESIAN_POINT('Ctrl Pts',(105.5,46.5625000027312,43.6995308303615));
#9461=CARTESIAN_POINT('Ctrl Pts',(74.5997654151808,46.5000000027312,74.5997654151808));
#9462=CARTESIAN_POINT('Ctrl Pts',(43.6995308303616,46.4375000027312,105.5));
#9463=CARTESIAN_POINT('Ctrl Pts',(1.93800355965069E-14,46.3750000027312,
105.5));
#9464=CARTESIAN_POINT('Ctrl Pts',(-43.6995308303616,46.3125000027312,105.5));
#9465=CARTESIAN_POINT('Ctrl Pts',(-74.5997654151808,46.2500000027312,74.5997654151808));
#9466=CARTESIAN_POINT('Ctrl Pts',(-105.5,46.1875000027312,43.6995308303616));
#9467=CARTESIAN_POINT('Ctrl Pts',(-105.5,46.1250000027312,0.));
#9468=CARTESIAN_POINT('Ctrl Pts',(-105.5,46.0625000027312,-43.6995308303615));
#9469=CARTESIAN_POINT('Ctrl Pts',(-74.5997654151808,46.0000000027312,-74.5997654151808));
#9470=CARTESIAN_POINT('Ctrl Pts',(-43.6995308303615,45.9375000027312,-105.5));
#9471=CARTESIAN_POINT('Ctrl Pts',(-6.46001186550229E-15,45.8750000027312,
-105.5));
#9472=CARTESIAN_POINT('Ctrl Pts',(43.6995308303615,45.8125000027312,-105.5));
#9473=CARTESIAN_POINT('Ctrl Pts',(74.5997654151808,45.7500000027312,-74.5997654151808));
#9474=CARTESIAN_POINT('Ctrl Pts',(105.5,45.6875000027312,-43.6995308303616));
#9475=CARTESIAN_POINT('Ctrl Pts',(105.5,45.6250000027312,-1.29200237310046E-14));
#9476=CARTESIAN_POINT('Ctrl Pts',(105.5,45.5625000027312,43.6995308303615));
#9477=CARTESIAN_POINT('Ctrl Pts',(74.5997654151808,45.5000000027312,74.5997654151808));
#9478=CARTESIAN_POINT('Ctrl Pts',(43.6995308303616,45.4375000027312,105.5));
#9479=CARTESIAN_POINT('Ctrl Pts',(1.93800355965069E-14,45.3750000027312,
105.5));
#9480=CARTESIAN_POINT('Ctrl Pts',(-43.6995308303616,45.3125000027312,105.5));
#9481=CARTESIAN_POINT('Ctrl Pts',(-74.5997654151808,45.2500000027312,74.5997654151808));
#9482=CARTESIAN_POINT('Ctrl Pts',(-105.5,45.1875000027312,43.6995308303616));
#9483=CARTESIAN_POINT('Ctrl Pts',(-105.5,45.1250000027312,0.));
#9484=CARTESIAN_POINT('Ctrl Pts',(-105.5,45.0625000027312,-43.6995308303615));
#9485=CARTESIAN_POINT('Ctrl Pts',(-74.5997654151808,45.0000000027312,-74.5997654151808));
#9486=CARTESIAN_POINT('Ctrl Pts',(-43.6995308303615,44.9375000027312,-105.5));
#9487=CARTESIAN_POINT('Ctrl Pts',(-6.46001186550229E-15,44.8750000027312,
-105.5));
#9488=CARTESIAN_POINT('Ctrl Pts',(43.6995308303615,44.8125000027312,-105.5));
#9489=CARTESIAN_POINT('Ctrl Pts',(74.5997654151808,44.7500000027312,-74.5997654151808));
#9490=CARTESIAN_POINT('Ctrl Pts',(105.5,44.6875000027312,-43.6995308303616));
#9491=CARTESIAN_POINT('Ctrl Pts',(105.5,44.6250000027312,-1.29200237310046E-14));
#9492=CARTESIAN_POINT('Ctrl Pts',(105.5,44.5625000027312,43.6995308303615));
#9493=CARTESIAN_POINT('Ctrl Pts',(74.5997654151808,44.5000000027312,74.5997654151808));
#9494=CARTESIAN_POINT('Ctrl Pts',(43.6995308303616,44.4375000027312,105.5));
#9495=CARTESIAN_POINT('Ctrl Pts',(1.93800355965069E-14,44.3750000027312,
105.5));
#9496=CARTESIAN_POINT('Ctrl Pts',(-43.6995308303616,44.3125000027312,105.5));
#9497=CARTESIAN_POINT('Ctrl Pts',(-74.5997654151808,44.2500000027312,74.5997654151808));
#9498=CARTESIAN_POINT('Ctrl Pts',(-105.5,44.1875000027312,43.6995308303616));
#9499=CARTESIAN_POINT('Ctrl Pts',(-105.5,44.1250000027312,0.));
#9500=CARTESIAN_POINT('Ctrl Pts',(-105.5,44.0625000027312,-43.6995308303615));
#9501=CARTESIAN_POINT('Ctrl Pts',(-74.5997654151808,44.0000000027312,-74.5997654151808));
#9502=CARTESIAN_POINT('Ctrl Pts',(-43.6995308303615,43.9375000027312,-105.5));
#9503=CARTESIAN_POINT('Ctrl Pts',(-6.46001186550229E-15,43.8750000027312,
-105.5));
#9504=CARTESIAN_POINT('Ctrl Pts',(43.6995308303615,43.8125000027312,-105.5));
#9505=CARTESIAN_POINT('Ctrl Pts',(74.5997654151808,43.7500000027312,-74.5997654151808));
#9506=CARTESIAN_POINT('Ctrl Pts',(105.5,43.6875000027312,-43.6995308303616));
#9507=CARTESIAN_POINT('Ctrl Pts',(105.5,43.6250000027312,-1.29200237310046E-14));
#9508=CARTESIAN_POINT('Ctrl Pts',(105.5,43.5625000027312,43.6995308303615));
#9509=CARTESIAN_POINT('Ctrl Pts',(74.5997654151808,43.5000000027312,74.5997654151808));
#9510=CARTESIAN_POINT('Ctrl Pts',(43.6995308303616,43.4375000027312,105.5));
#9511=CARTESIAN_POINT('Ctrl Pts',(1.93800355965069E-14,43.3750000027312,
105.5));
#9512=CARTESIAN_POINT('Ctrl Pts',(-43.6995308303616,43.3125000027312,105.5));
#9513=CARTESIAN_POINT('Ctrl Pts',(-74.5997654151808,43.2500000027312,74.5997654151808));
#9514=CARTESIAN_POINT('Ctrl Pts',(-105.5,43.1875000027312,43.6995308303616));
#9515=CARTESIAN_POINT('Ctrl Pts',(-105.5,43.1250000027312,0.));
#9516=CARTESIAN_POINT('Ctrl Pts',(-105.5,43.0625000027312,-43.6995308303615));
#9517=CARTESIAN_POINT('Ctrl Pts',(-74.5997654151808,43.0000000027312,-74.5997654151808));
#9518=CARTESIAN_POINT('Ctrl Pts',(-43.6995308303615,42.9375000027312,-105.5));
#9519=CARTESIAN_POINT('Ctrl Pts',(-6.46001186550229E-15,42.8750000027312,
-105.5));
#9520=CARTESIAN_POINT('Ctrl Pts',(43.6995308303615,42.8125000027312,-105.5));
#9521=CARTESIAN_POINT('Ctrl Pts',(74.5997654151808,42.7500000027312,-74.5997654151808));
#9522=CARTESIAN_POINT('Ctrl Pts',(105.5,42.6875000027312,-43.6995308303616));
#9523=CARTESIAN_POINT('Ctrl Pts',(105.5,42.6250000027312,-1.29200237310046E-14));
#9524=CARTESIAN_POINT('Ctrl Pts',(105.5,42.5625000027312,43.6995308303615));
#9525=CARTESIAN_POINT('Ctrl Pts',(74.5997654151808,42.5000000027312,74.5997654151808));
#9526=CARTESIAN_POINT('Ctrl Pts',(43.6995308303616,42.4375000027312,105.5));
#9527=CARTESIAN_POINT('Ctrl Pts',(1.93800355965069E-14,42.3750000027312,
105.5));
#9528=CARTESIAN_POINT('Ctrl Pts',(-43.6995308303616,42.3125000027312,105.5));
#9529=CARTESIAN_POINT('Ctrl Pts',(-74.5997654151808,42.2500000027312,74.5997654151808));
#9530=CARTESIAN_POINT('Ctrl Pts',(-105.5,42.1875000027312,43.6995308303616));
#9531=CARTESIAN_POINT('Ctrl Pts',(-105.5,42.1250000027312,0.));
#9532=CARTESIAN_POINT('Ctrl Pts',(-105.5,42.0625000027312,-43.6995308303615));
#9533=CARTESIAN_POINT('Ctrl Pts',(-74.5997654151808,42.0000000027312,-74.5997654151808));
#9534=CARTESIAN_POINT('Ctrl Pts',(-43.6995308303615,41.9375000027312,-105.5));
#9535=CARTESIAN_POINT('Ctrl Pts',(-6.46001186550229E-15,41.8750000027312,
-105.5));
#9536=CARTESIAN_POINT('Ctrl Pts',(43.6995308303615,41.8125000027312,-105.5));
#9537=CARTESIAN_POINT('Ctrl Pts',(74.5997654151808,41.7500000027312,-74.5997654151808));
#9538=CARTESIAN_POINT('Ctrl Pts',(105.5,41.6875000027312,-43.6995308303616));
#9539=CARTESIAN_POINT('Ctrl Pts',(105.5,41.6250000027312,-1.29200237310046E-14));
#9540=CARTESIAN_POINT('Ctrl Pts',(105.5,41.5625000027312,43.6995308303615));
#9541=CARTESIAN_POINT('Ctrl Pts',(74.5997654151808,41.5000000027312,74.5997654151808));
#9542=CARTESIAN_POINT('Ctrl Pts',(43.6995308303616,41.4375000027312,105.5));
#9543=CARTESIAN_POINT('Ctrl Pts',(1.93800355965069E-14,41.3750000027312,
105.5));
#9544=CARTESIAN_POINT('Ctrl Pts',(-43.6995308303616,41.3125000027312,105.5));
#9545=CARTESIAN_POINT('Ctrl Pts',(-74.5997654151808,41.2500000027312,74.5997654151808));
#9546=CARTESIAN_POINT('Ctrl Pts',(-105.5,41.1875000027312,43.6995308303616));
#9547=CARTESIAN_POINT('Ctrl Pts',(-105.5,41.1250000027312,0.));
#9548=CARTESIAN_POINT('Ctrl Pts',(-105.5,41.0625000027312,-43.6995308303615));
#9549=CARTESIAN_POINT('Ctrl Pts',(-74.5997654151808,41.0000000027312,-74.5997654151808));
#9550=CARTESIAN_POINT('Ctrl Pts',(-43.6995308303615,40.9375000027312,-105.5));
#9551=CARTESIAN_POINT('Ctrl Pts',(-6.46001186550229E-15,40.8750000027312,
-105.5));
#9552=CARTESIAN_POINT('Ctrl Pts',(43.6995308303615,40.8125000027312,-105.5));
#9553=CARTESIAN_POINT('Ctrl Pts',(74.5997654151808,40.7500000027312,-74.5997654151808));
#9554=CARTESIAN_POINT('Ctrl Pts',(105.5,40.6875000027312,-43.6995308303616));
#9555=CARTESIAN_POINT('Ctrl Pts',(105.5,40.6250000027312,-1.29200237310046E-14));
#9556=CARTESIAN_POINT('Ctrl Pts',(105.5,40.5625000027312,43.6995308303615));
#9557=CARTESIAN_POINT('Ctrl Pts',(74.5997654151808,40.5000000027312,74.5997654151808));
#9558=CARTESIAN_POINT('Ctrl Pts',(43.6995308303616,40.4375000027312,105.5));
#9559=CARTESIAN_POINT('Ctrl Pts',(1.93800355965069E-14,40.3750000027312,
105.5));
#9560=CARTESIAN_POINT('Ctrl Pts',(-43.6995308303616,40.3125000027312,105.5));
#9561=CARTESIAN_POINT('Ctrl Pts',(-74.5997654151808,40.2500000027312,74.5997654151808));
#9562=CARTESIAN_POINT('Ctrl Pts',(-105.5,40.1875000027312,43.6995308303616));
#9563=CARTESIAN_POINT('Ctrl Pts',(-105.5,40.1250000027312,0.));
#9564=CARTESIAN_POINT('Ctrl Pts',(-105.5,40.0625000027312,-43.6995308303615));
#9565=CARTESIAN_POINT('Ctrl Pts',(-74.5997654151808,40.0000000027312,-74.5997654151808));
#9566=CARTESIAN_POINT('Ctrl Pts',(-43.6995308303615,39.9375000027312,-105.5));
#9567=CARTESIAN_POINT('Ctrl Pts',(-6.46001186550229E-15,39.8750000027312,
-105.5));
#9568=CARTESIAN_POINT('Ctrl Pts',(43.6995308303615,39.8125000027312,-105.5));
#9569=CARTESIAN_POINT('Ctrl Pts',(74.5997654151808,39.7500000027312,-74.5997654151808));
#9570=CARTESIAN_POINT('Ctrl Pts',(105.5,39.6875000027312,-43.6995308303616));
#9571=CARTESIAN_POINT('Ctrl Pts',(105.5,39.6250000027312,-1.29200237310046E-14));
#9572=CARTESIAN_POINT('Ctrl Pts',(105.5,39.5625000027312,43.6995308303615));
#9573=CARTESIAN_POINT('Ctrl Pts',(74.5997654151808,39.5000000027312,74.5997654151808));
#9574=CARTESIAN_POINT('Ctrl Pts',(43.6995308303616,39.4375000027312,105.5));
#9575=CARTESIAN_POINT('Ctrl Pts',(1.93800355965069E-14,39.3750000027312,
105.5));
#9576=CARTESIAN_POINT('Ctrl Pts',(-43.6995308303616,39.3125000027312,105.5));
#9577=CARTESIAN_POINT('Ctrl Pts',(-74.5997654151808,39.2500000027312,74.5997654151808));
#9578=CARTESIAN_POINT('Ctrl Pts',(-105.5,39.1875000027312,43.6995308303616));
#9579=CARTESIAN_POINT('Ctrl Pts',(-105.5,39.1250000027312,0.));
#9580=CARTESIAN_POINT('Ctrl Pts',(-105.5,39.0625000027312,-43.6995308303615));
#9581=CARTESIAN_POINT('Ctrl Pts',(-74.5997654151808,39.0000000027312,-74.5997654151808));
#9582=CARTESIAN_POINT('Ctrl Pts',(-43.6995308303615,38.9375000027312,-105.5));
#9583=CARTESIAN_POINT('Ctrl Pts',(-6.46001186550229E-15,38.8750000027312,
-105.5));
#9584=CARTESIAN_POINT('Ctrl Pts',(43.6995308303615,38.8125000027312,-105.5));
#9585=CARTESIAN_POINT('Ctrl Pts',(74.5997654151808,38.7500000027312,-74.5997654151808));
#9586=CARTESIAN_POINT('Ctrl Pts',(105.5,38.6875000027312,-43.6995308303616));
#9587=CARTESIAN_POINT('Ctrl Pts',(105.5,38.6250000027312,-1.29200237310046E-14));
#9588=CARTESIAN_POINT('Ctrl Pts',(105.5,38.5625000027312,43.6995308303615));
#9589=CARTESIAN_POINT('Ctrl Pts',(74.5997654151808,38.5000000027312,74.5997654151808));
#9590=CARTESIAN_POINT('Ctrl Pts',(43.6995308303616,38.4375000027312,105.5));
#9591=CARTESIAN_POINT('Ctrl Pts',(1.93800355965069E-14,38.3750000027312,
105.5));
#9592=CARTESIAN_POINT('Ctrl Pts',(-43.6995308303616,38.3125000027312,105.5));
#9593=CARTESIAN_POINT('Ctrl Pts',(-74.5997654151808,38.2500000027312,74.5997654151808));
#9594=CARTESIAN_POINT('Ctrl Pts',(-105.5,38.1875000027312,43.6995308303616));
#9595=CARTESIAN_POINT('Ctrl Pts',(-105.5,38.1250000027312,0.));
#9596=CARTESIAN_POINT('Ctrl Pts',(-105.5,38.0625000027312,-43.6995308303615));
#9597=CARTESIAN_POINT('Ctrl Pts',(-74.5997654151808,38.0000000027312,-74.5997654151808));
#9598=CARTESIAN_POINT('Ctrl Pts',(-43.6995308303615,37.9375000027312,-105.5));
#9599=CARTESIAN_POINT('Ctrl Pts',(-6.46001186550229E-15,37.8750000027312,
-105.5));
#9600=CARTESIAN_POINT('Ctrl Pts',(43.6995308303615,37.8125000027312,-105.5));
#9601=CARTESIAN_POINT('Ctrl Pts',(74.5997654151808,37.7500000027312,-74.5997654151808));
#9602=CARTESIAN_POINT('Ctrl Pts',(105.5,37.6875000027312,-43.6995308303616));
#9603=CARTESIAN_POINT('Ctrl Pts',(105.5,37.6250000027312,-1.29200237310046E-14));
#9604=CARTESIAN_POINT('Ctrl Pts',(105.5,37.5625000027312,43.6995308303615));
#9605=CARTESIAN_POINT('Ctrl Pts',(74.5997654151808,37.5000000027312,74.5997654151808));
#9606=CARTESIAN_POINT('Ctrl Pts',(43.6995308303616,37.4375000027312,105.5));
#9607=CARTESIAN_POINT('Ctrl Pts',(1.93800355965069E-14,37.3750000027312,
105.5));
#9608=CARTESIAN_POINT('Ctrl Pts',(-43.6995308303616,37.3125000027312,105.5));
#9609=CARTESIAN_POINT('Ctrl Pts',(-74.5997654151808,37.2500000027312,74.5997654151808));
#9610=CARTESIAN_POINT('Ctrl Pts',(-105.5,37.1875000027312,43.6995308303616));
#9611=CARTESIAN_POINT('Ctrl Pts',(-105.5,37.1250000027312,0.));
#9612=CARTESIAN_POINT('Ctrl Pts',(-105.5,37.0625000027312,-43.6995308303615));
#9613=CARTESIAN_POINT('Ctrl Pts',(-74.5997654151808,37.0000000027312,-74.5997654151808));
#9614=CARTESIAN_POINT('Ctrl Pts',(-43.6995308303615,36.9375000027312,-105.5));
#9615=CARTESIAN_POINT('Ctrl Pts',(-6.46001186550229E-15,36.8750000027312,
-105.5));
#9616=CARTESIAN_POINT('Ctrl Pts',(43.6995308303615,36.8125000027312,-105.5));
#9617=CARTESIAN_POINT('Ctrl Pts',(74.5997654151808,36.7500000027312,-74.5997654151808));
#9618=CARTESIAN_POINT('Ctrl Pts',(105.5,36.6875000027312,-43.6995308303616));
#9619=CARTESIAN_POINT('Ctrl Pts',(105.5,36.6250000027312,-1.29200237310046E-14));
#9620=CARTESIAN_POINT('Ctrl Pts',(105.5,36.5625000027312,43.6995308303615));
#9621=CARTESIAN_POINT('Ctrl Pts',(74.5997654151808,36.5000000027312,74.5997654151808));
#9622=CARTESIAN_POINT('Ctrl Pts',(43.6995308303616,36.4375000027312,105.5));
#9623=CARTESIAN_POINT('Ctrl Pts',(1.93800355965069E-14,36.3750000027312,
105.5));
#9624=CARTESIAN_POINT('Ctrl Pts',(-43.6995308303616,36.3125000027312,105.5));
#9625=CARTESIAN_POINT('Ctrl Pts',(-74.5997654151808,36.2500000027312,74.5997654151808));
#9626=CARTESIAN_POINT('Ctrl Pts',(-105.5,36.1875000027312,43.6995308303616));
#9627=CARTESIAN_POINT('Ctrl Pts',(-105.5,36.1250000027312,0.));
#9628=CARTESIAN_POINT('Ctrl Pts',(-105.5,36.0625000027312,-43.6995308303615));
#9629=CARTESIAN_POINT('Ctrl Pts',(-74.5997654151808,36.0000000027312,-74.5997654151808));
#9630=CARTESIAN_POINT('Ctrl Pts',(-43.6995308303615,35.9375000027312,-105.5));
#9631=CARTESIAN_POINT('Ctrl Pts',(-6.46001186550229E-15,35.8750000027312,
-105.5));
#9632=CARTESIAN_POINT('Ctrl Pts',(43.6995308303615,35.8125000027312,-105.5));
#9633=CARTESIAN_POINT('Ctrl Pts',(74.5997654151808,35.7500000027312,-74.5997654151808));
#9634=CARTESIAN_POINT('Ctrl Pts',(105.5,35.6875000027312,-43.6995308303616));
#9635=CARTESIAN_POINT('Ctrl Pts',(105.5,35.6250000027312,-1.29200237310046E-14));
#9636=CARTESIAN_POINT('Ctrl Pts',(105.5,35.5625000027312,43.6995308303615));
#9637=CARTESIAN_POINT('Ctrl Pts',(74.5997654151808,35.5000000027312,74.5997654151808));
#9638=CARTESIAN_POINT('Ctrl Pts',(43.6995308303616,35.4375000027312,105.5));
#9639=CARTESIAN_POINT('Ctrl Pts',(1.93800355965069E-14,35.3750000027312,
105.5));
#9640=CARTESIAN_POINT('Ctrl Pts',(-43.6995308303616,35.3125000027312,105.5));
#9641=CARTESIAN_POINT('Ctrl Pts',(-74.5997654151808,35.2500000027312,74.5997654151808));
#9642=CARTESIAN_POINT('Ctrl Pts',(-105.5,35.1875000027312,43.6995308303616));
#9643=CARTESIAN_POINT('Ctrl Pts',(-105.5,35.1250000027312,0.));
#9644=CARTESIAN_POINT('Ctrl Pts',(-105.5,35.0625000027312,-43.6995308303615));
#9645=CARTESIAN_POINT('Ctrl Pts',(-74.5997654151808,35.0000000027312,-74.5997654151808));
#9646=CARTESIAN_POINT('Ctrl Pts',(-43.6995308303615,34.9375000027312,-105.5));
#9647=CARTESIAN_POINT('Ctrl Pts',(-6.46001186550229E-15,34.8750000027312,
-105.5));
#9648=CARTESIAN_POINT('Ctrl Pts',(43.6995308303615,34.8125000027312,-105.5));
#9649=CARTESIAN_POINT('Ctrl Pts',(74.5997654151808,34.7500000027312,-74.5997654151808));
#9650=CARTESIAN_POINT('Ctrl Pts',(105.5,34.6875000027312,-43.6995308303616));
#9651=CARTESIAN_POINT('Ctrl Pts',(105.5,34.6250000027312,-1.29200237310046E-14));
#9652=CARTESIAN_POINT('Ctrl Pts',(105.5,34.5625000027312,43.6995308303615));
#9653=CARTESIAN_POINT('Ctrl Pts',(74.5997654151808,34.5000000027312,74.5997654151808));
#9654=CARTESIAN_POINT('Ctrl Pts',(43.6995308303616,34.4375000027312,105.5));
#9655=CARTESIAN_POINT('Ctrl Pts',(1.93800355965069E-14,34.3750000027312,
105.5));
#9656=CARTESIAN_POINT('Ctrl Pts',(-43.6995308303616,34.3125000027312,105.5));
#9657=CARTESIAN_POINT('Ctrl Pts',(-74.5997654151808,34.2500000027312,74.5997654151808));
#9658=CARTESIAN_POINT('Ctrl Pts',(-105.5,34.1875000027312,43.6995308303616));
#9659=CARTESIAN_POINT('Ctrl Pts',(-105.5,34.1250000027312,0.));
#9660=CARTESIAN_POINT('Ctrl Pts',(-105.5,34.0625000027312,-43.6995308303615));
#9661=CARTESIAN_POINT('Ctrl Pts',(-74.5997654151808,34.0000000027312,-74.5997654151808));
#9662=CARTESIAN_POINT('Ctrl Pts',(-43.6995308303615,33.9375000027312,-105.5));
#9663=CARTESIAN_POINT('Ctrl Pts',(-6.46001186550229E-15,33.8750000027312,
-105.5));
#9664=CARTESIAN_POINT('Ctrl Pts',(43.6995308303615,33.8125000027312,-105.5));
#9665=CARTESIAN_POINT('Ctrl Pts',(74.5997654151808,33.7500000027312,-74.5997654151808));
#9666=CARTESIAN_POINT('Ctrl Pts',(105.5,33.6875000027312,-43.6995308303616));
#9667=CARTESIAN_POINT('Ctrl Pts',(105.5,33.6250000027312,-1.29200237310046E-14));
#9668=CARTESIAN_POINT('Ctrl Pts',(105.5,33.5625000027312,43.6995308303615));
#9669=CARTESIAN_POINT('Ctrl Pts',(74.5997654151808,33.5000000027312,74.5997654151808));
#9670=CARTESIAN_POINT('Ctrl Pts',(43.6995308303616,33.4375000027312,105.5));
#9671=CARTESIAN_POINT('Ctrl Pts',(1.93800355965069E-14,33.3750000027312,
105.5));
#9672=CARTESIAN_POINT('Ctrl Pts',(-43.6995308303616,33.3125000027312,105.5));
#9673=CARTESIAN_POINT('Ctrl Pts',(-74.5997654151808,33.2500000027312,74.5997654151808));
#9674=CARTESIAN_POINT('Ctrl Pts',(-105.5,33.1875000027312,43.6995308303616));
#9675=CARTESIAN_POINT('Ctrl Pts',(-105.5,33.1250000027312,0.));
#9676=CARTESIAN_POINT('Ctrl Pts',(-105.5,33.0625000027312,-43.6995308303615));
#9677=CARTESIAN_POINT('Ctrl Pts',(-74.5997654151808,33.0000000027312,-74.5997654151808));
#9678=CARTESIAN_POINT('Ctrl Pts',(-43.6995308303615,32.9375000027312,-105.5));
#9679=CARTESIAN_POINT('Ctrl Pts',(-6.46001186550229E-15,32.8750000027312,
-105.5));
#9680=CARTESIAN_POINT('Ctrl Pts',(43.6995308303615,32.8125000027312,-105.5));
#9681=CARTESIAN_POINT('Ctrl Pts',(74.5997654151808,32.7500000027312,-74.5997654151808));
#9682=CARTESIAN_POINT('Ctrl Pts',(105.5,32.6875000027312,-43.6995308303616));
#9683=CARTESIAN_POINT('Ctrl Pts',(105.5,32.6250000027312,-1.29200237310046E-14));
#9684=CARTESIAN_POINT('Ctrl Pts',(105.5,32.5625000027312,43.6995308303615));
#9685=CARTESIAN_POINT('Ctrl Pts',(74.5997654151808,32.5000000027312,74.5997654151808));
#9686=CARTESIAN_POINT('Ctrl Pts',(43.6995308303616,32.4375000027312,105.5));
#9687=CARTESIAN_POINT('Ctrl Pts',(1.93800355965069E-14,32.3750000027312,
105.5));
#9688=CARTESIAN_POINT('Ctrl Pts',(-43.6995308303616,32.3125000027312,105.5));
#9689=CARTESIAN_POINT('Ctrl Pts',(-74.5997654151808,32.2500000027312,74.5997654151808));
#9690=CARTESIAN_POINT('Ctrl Pts',(-105.5,32.1875000027312,43.6995308303616));
#9691=CARTESIAN_POINT('Ctrl Pts',(-105.5,32.1250000027312,0.));
#9692=CARTESIAN_POINT('Ctrl Pts',(-105.5,32.0625000027312,-43.6995308303615));
#9693=CARTESIAN_POINT('Ctrl Pts',(-74.5997654151808,32.0000000027312,-74.5997654151808));
#9694=CARTESIAN_POINT('Ctrl Pts',(-43.6995308303615,31.9375000027312,-105.5));
#9695=CARTESIAN_POINT('Ctrl Pts',(-6.46001186550229E-15,31.8750000027312,
-105.5));
#9696=CARTESIAN_POINT('Ctrl Pts',(43.6995308303615,31.8125000027312,-105.5));
#9697=CARTESIAN_POINT('Ctrl Pts',(74.5997654151808,31.7500000027312,-74.5997654151808));
#9698=CARTESIAN_POINT('Ctrl Pts',(105.5,31.6875000027312,-43.6995308303616));
#9699=CARTESIAN_POINT('Ctrl Pts',(105.5,31.6250000027312,-1.29200237310046E-14));
#9700=CARTESIAN_POINT('Ctrl Pts',(105.5,31.5625000027312,43.6995308303615));
#9701=CARTESIAN_POINT('Ctrl Pts',(74.5997654151808,31.5000000027312,74.5997654151808));
#9702=CARTESIAN_POINT('Ctrl Pts',(43.6995308303616,31.4375000027312,105.5));
#9703=CARTESIAN_POINT('Ctrl Pts',(1.93800355965069E-14,31.3750000027312,
105.5));
#9704=CARTESIAN_POINT('Ctrl Pts',(-43.6995308303616,31.3125000027312,105.5));
#9705=CARTESIAN_POINT('Ctrl Pts',(-74.5997654151808,31.2500000027312,74.5997654151808));
#9706=CARTESIAN_POINT('Ctrl Pts',(-105.5,31.1875000027312,43.6995308303616));
#9707=CARTESIAN_POINT('Ctrl Pts',(-105.5,31.1250000027312,0.));
#9708=CARTESIAN_POINT('Ctrl Pts',(-105.5,31.0625000027312,-43.6995308303615));
#9709=CARTESIAN_POINT('Ctrl Pts',(-74.5997654151808,31.0000000027312,-74.5997654151808));
#9710=CARTESIAN_POINT('Ctrl Pts',(-43.6995308303615,30.9375000027312,-105.5));
#9711=CARTESIAN_POINT('Ctrl Pts',(-6.46001186550229E-15,30.8750000027312,
-105.5));
#9712=CARTESIAN_POINT('Ctrl Pts',(43.6995308303615,30.8125000027312,-105.5));
#9713=CARTESIAN_POINT('Ctrl Pts',(74.5997654151808,30.7500000027312,-74.5997654151808));
#9714=CARTESIAN_POINT('Ctrl Pts',(105.5,30.6875000027312,-43.6995308303616));
#9715=CARTESIAN_POINT('Ctrl Pts',(105.5,30.6250000027312,-1.29200237310046E-14));
#9716=CARTESIAN_POINT('Ctrl Pts',(105.5,30.5625000027312,43.6995308303615));
#9717=CARTESIAN_POINT('Ctrl Pts',(74.5997654151808,30.5000000027312,74.5997654151808));
#9718=CARTESIAN_POINT('Ctrl Pts',(43.6995308303616,30.4375000027312,105.5));
#9719=CARTESIAN_POINT('Ctrl Pts',(1.93800355965069E-14,30.3750000027312,
105.5));
#9720=CARTESIAN_POINT('Ctrl Pts',(-43.6995308303616,30.3125000027312,105.5));
#9721=CARTESIAN_POINT('Ctrl Pts',(-74.5997654151808,30.2500000027312,74.5997654151808));
#9722=CARTESIAN_POINT('Ctrl Pts',(-105.5,30.1875000027312,43.6995308303616));
#9723=CARTESIAN_POINT('Ctrl Pts',(-105.5,30.1250000027312,0.));
#9724=CARTESIAN_POINT('Ctrl Pts',(-105.5,30.0625000027312,-43.6995308303615));
#9725=CARTESIAN_POINT('Ctrl Pts',(-74.5997654151808,30.0000000027312,-74.5997654151808));
#9726=CARTESIAN_POINT('Ctrl Pts',(-43.6995308303615,29.9375000027312,-105.5));
#9727=CARTESIAN_POINT('Ctrl Pts',(-6.46001186550229E-15,29.8750000027312,
-105.5));
#9728=CARTESIAN_POINT('Ctrl Pts',(43.6995308303615,29.8125000027312,-105.5));
#9729=CARTESIAN_POINT('Ctrl Pts',(74.5997654151808,29.7500000027312,-74.5997654151808));
#9730=CARTESIAN_POINT('Ctrl Pts',(105.5,29.6875000027312,-43.6995308303616));
#9731=CARTESIAN_POINT('Ctrl Pts',(105.5,29.6250000027312,-1.29200237310046E-14));
#9732=CARTESIAN_POINT('Ctrl Pts',(105.5,29.5625000027312,43.6995308303615));
#9733=CARTESIAN_POINT('Ctrl Pts',(74.5997654151808,29.5000000027312,74.5997654151808));
#9734=CARTESIAN_POINT('Ctrl Pts',(43.6995308303616,29.4375000027312,105.5));
#9735=CARTESIAN_POINT('Ctrl Pts',(1.93800355965069E-14,29.3750000027312,
105.5));
#9736=CARTESIAN_POINT('Ctrl Pts',(-43.6995308303616,29.3125000027312,105.5));
#9737=CARTESIAN_POINT('Ctrl Pts',(-74.5997654151808,29.2500000027312,74.5997654151808));
#9738=CARTESIAN_POINT('Ctrl Pts',(-105.5,29.1875000027312,43.6995308303616));
#9739=CARTESIAN_POINT('Ctrl Pts',(-105.5,29.1250000027312,0.));
#9740=CARTESIAN_POINT('Ctrl Pts',(-105.5,29.0625000027312,-43.6995308303615));
#9741=CARTESIAN_POINT('Ctrl Pts',(-74.5997654151808,29.0000000027312,-74.5997654151808));
#9742=CARTESIAN_POINT('Ctrl Pts',(-43.6995308303615,28.9375000027312,-105.5));
#9743=CARTESIAN_POINT('Ctrl Pts',(-6.46001186550229E-15,28.8750000027312,
-105.5));
#9744=CARTESIAN_POINT('Ctrl Pts',(43.6995308303615,28.8125000027312,-105.5));
#9745=CARTESIAN_POINT('Ctrl Pts',(74.5997654151808,28.7500000027312,-74.5997654151808));
#9746=CARTESIAN_POINT('Ctrl Pts',(105.5,28.6875000027312,-43.6995308303616));
#9747=CARTESIAN_POINT('Ctrl Pts',(105.5,28.6250000027312,-1.29200237310046E-14));
#9748=CARTESIAN_POINT('Ctrl Pts',(105.5,28.5625000027312,43.6995308303615));
#9749=CARTESIAN_POINT('Ctrl Pts',(74.5997654151808,28.5000000027312,74.5997654151808));
#9750=CARTESIAN_POINT('Ctrl Pts',(43.6995308303616,28.4375000027312,105.5));
#9751=CARTESIAN_POINT('Ctrl Pts',(1.93800355965069E-14,28.3750000027312,
105.5));
#9752=CARTESIAN_POINT('Ctrl Pts',(-43.6995308303616,28.3125000027312,105.5));
#9753=CARTESIAN_POINT('Ctrl Pts',(-74.5997654151808,28.2500000027312,74.5997654151808));
#9754=CARTESIAN_POINT('Ctrl Pts',(-105.5,28.1875000027312,43.6995308303616));
#9755=CARTESIAN_POINT('Ctrl Pts',(-105.5,28.1250000027312,0.));
#9756=CARTESIAN_POINT('Ctrl Pts',(-105.5,28.0625000027312,-43.6995308303615));
#9757=CARTESIAN_POINT('Ctrl Pts',(-74.5997654151808,28.0000000027312,-74.5997654151808));
#9758=CARTESIAN_POINT('Ctrl Pts',(-43.6995308303615,27.9375000027312,-105.5));
#9759=CARTESIAN_POINT('Ctrl Pts',(-6.46001186550229E-15,27.8750000027312,
-105.5));
#9760=CARTESIAN_POINT('Ctrl Pts',(43.6995308303615,27.8125000027312,-105.5));
#9761=CARTESIAN_POINT('Ctrl Pts',(74.5997654151808,27.7500000027312,-74.5997654151808));
#9762=CARTESIAN_POINT('Ctrl Pts',(105.5,27.6875000027312,-43.6995308303616));
#9763=CARTESIAN_POINT('Ctrl Pts',(105.5,27.6250000027312,-1.29200237310046E-14));
#9764=CARTESIAN_POINT('Ctrl Pts',(105.5,27.5625000027312,43.6995308303615));
#9765=CARTESIAN_POINT('Ctrl Pts',(74.5997654151808,27.5000000027312,74.5997654151808));
#9766=CARTESIAN_POINT('Ctrl Pts',(43.6995308303616,27.4375000027312,105.5));
#9767=CARTESIAN_POINT('Ctrl Pts',(1.93800355965069E-14,27.3750000027312,
105.5));
#9768=CARTESIAN_POINT('Ctrl Pts',(-43.6995308303616,27.3125000027312,105.5));
#9769=CARTESIAN_POINT('Ctrl Pts',(-74.5997654151808,27.2500000027312,74.5997654151808));
#9770=CARTESIAN_POINT('Ctrl Pts',(-105.5,27.1875000027312,43.6995308303616));
#9771=CARTESIAN_POINT('Ctrl Pts',(-105.5,27.1250000027312,0.));
#9772=CARTESIAN_POINT('Ctrl Pts',(-105.5,27.0625000027312,-43.6995308303615));
#9773=CARTESIAN_POINT('Ctrl Pts',(-74.5997654151808,27.0000000027312,-74.5997654151808));
#9774=CARTESIAN_POINT('Ctrl Pts',(-43.6995308303615,26.9375000027312,-105.5));
#9775=CARTESIAN_POINT('Ctrl Pts',(-6.46001186550229E-15,26.8750000027312,
-105.5));
#9776=CARTESIAN_POINT('Ctrl Pts',(43.6995308303615,26.8125000027312,-105.5));
#9777=CARTESIAN_POINT('Ctrl Pts',(74.5997654151808,26.7500000027312,-74.5997654151808));
#9778=CARTESIAN_POINT('Ctrl Pts',(105.5,26.6875000027312,-43.6995308303616));
#9779=CARTESIAN_POINT('Ctrl Pts',(105.5,26.6250000027312,-1.29200237310046E-14));
#9780=CARTESIAN_POINT('Ctrl Pts',(105.5,26.5625000027312,43.6995308303615));
#9781=CARTESIAN_POINT('Ctrl Pts',(74.5997654151808,26.5000000027312,74.5997654151808));
#9782=CARTESIAN_POINT('Ctrl Pts',(43.6995308303616,26.4375000027312,105.5));
#9783=CARTESIAN_POINT('Ctrl Pts',(1.93800355965069E-14,26.3750000027312,
105.5));
#9784=CARTESIAN_POINT('Ctrl Pts',(-43.6995308303616,26.3125000027312,105.5));
#9785=CARTESIAN_POINT('Ctrl Pts',(-74.5997654151808,26.2500000027312,74.5997654151808));
#9786=CARTESIAN_POINT('Ctrl Pts',(-105.5,26.1875000027312,43.6995308303616));
#9787=CARTESIAN_POINT('Ctrl Pts',(-105.5,26.1250000027312,0.));
#9788=CARTESIAN_POINT('Ctrl Pts',(-105.5,26.0625000027312,-43.6995308303615));
#9789=CARTESIAN_POINT('Ctrl Pts',(-74.5997654151808,26.0000000027312,-74.5997654151808));
#9790=CARTESIAN_POINT('Ctrl Pts',(-43.6995308303615,25.9375000027312,-105.5));
#9791=CARTESIAN_POINT('Ctrl Pts',(-6.46001186550229E-15,25.8750000027312,
-105.5));
#9792=CARTESIAN_POINT('Ctrl Pts',(43.6995308303615,25.8125000027312,-105.5));
#9793=CARTESIAN_POINT('Ctrl Pts',(74.5997654151808,25.7500000027312,-74.5997654151808));
#9794=CARTESIAN_POINT('Ctrl Pts',(105.5,25.6875000027312,-43.6995308303616));
#9795=CARTESIAN_POINT('Ctrl Pts',(105.5,25.6250000027312,-1.29200237310046E-14));
#9796=CARTESIAN_POINT('Ctrl Pts',(105.5,25.5625000027312,43.6995308303615));
#9797=CARTESIAN_POINT('Ctrl Pts',(74.5997654151808,25.5000000027312,74.5997654151808));
#9798=CARTESIAN_POINT('Ctrl Pts',(43.6995308303616,25.4375000027312,105.5));
#9799=CARTESIAN_POINT('Ctrl Pts',(1.93800355965069E-14,25.3750000027312,
105.5));
#9800=CARTESIAN_POINT('Ctrl Pts',(-43.6995308303616,25.3125000027312,105.5));
#9801=CARTESIAN_POINT('Ctrl Pts',(-74.5997654151808,25.2500000027312,74.5997654151808));
#9802=CARTESIAN_POINT('Ctrl Pts',(-105.5,25.1875000027312,43.6995308303616));
#9803=CARTESIAN_POINT('Ctrl Pts',(-105.5,25.1250000027312,0.));
#9804=CARTESIAN_POINT('Ctrl Pts',(-105.5,25.0625000027312,-43.6995308303615));
#9805=CARTESIAN_POINT('Ctrl Pts',(-74.5997654151808,25.0000000027312,-74.5997654151808));
#9806=CARTESIAN_POINT('Ctrl Pts',(-43.6995308303615,24.9375000027312,-105.5));
#9807=CARTESIAN_POINT('Ctrl Pts',(-6.46001186550229E-15,24.8750000027312,
-105.5));
#9808=CARTESIAN_POINT('Ctrl Pts',(43.6995308303615,24.8125000027312,-105.5));
#9809=CARTESIAN_POINT('Ctrl Pts',(74.5997654151808,24.7500000027312,-74.5997654151808));
#9810=CARTESIAN_POINT('Ctrl Pts',(105.5,24.6875000027312,-43.6995308303616));
#9811=CARTESIAN_POINT('Ctrl Pts',(105.5,24.6250000027312,-1.29200237310046E-14));
#9812=CARTESIAN_POINT('Ctrl Pts',(105.5,24.5625000027312,43.6995308303615));
#9813=CARTESIAN_POINT('Ctrl Pts',(74.5997654151808,24.5000000027312,74.5997654151808));
#9814=CARTESIAN_POINT('Ctrl Pts',(43.6995308303616,24.4375000027312,105.5));
#9815=CARTESIAN_POINT('Ctrl Pts',(1.93800355965069E-14,24.3750000027312,
105.5));
#9816=CARTESIAN_POINT('Ctrl Pts',(-43.6995308303616,24.3125000027312,105.5));
#9817=CARTESIAN_POINT('Ctrl Pts',(-74.5997654151808,24.2500000027312,74.5997654151808));
#9818=CARTESIAN_POINT('Ctrl Pts',(-105.5,24.1875000027312,43.6995308303616));
#9819=CARTESIAN_POINT('Ctrl Pts',(-105.5,24.1250000027312,0.));
#9820=CARTESIAN_POINT('Ctrl Pts',(-105.5,24.0625000027312,-43.6995308303615));
#9821=CARTESIAN_POINT('Ctrl Pts',(-74.5997654151808,24.0000000027312,-74.5997654151808));
#9822=CARTESIAN_POINT('Ctrl Pts',(-43.6995308303615,23.9375000027312,-105.5));
#9823=CARTESIAN_POINT('Ctrl Pts',(-6.46001186550229E-15,23.8750000027312,
-105.5));
#9824=CARTESIAN_POINT('Ctrl Pts',(43.6995308303615,23.8125000027312,-105.5));
#9825=CARTESIAN_POINT('Ctrl Pts',(74.5997654151808,23.7500000027312,-74.5997654151808));
#9826=CARTESIAN_POINT('Ctrl Pts',(105.5,23.6875000027312,-43.6995308303616));
#9827=CARTESIAN_POINT('Ctrl Pts',(105.5,23.6250000027312,-1.29200237310046E-14));
#9828=CARTESIAN_POINT('Ctrl Pts',(105.5,23.5625000027312,43.6995308303615));
#9829=CARTESIAN_POINT('Ctrl Pts',(74.5997654151808,23.5000000027312,74.5997654151808));
#9830=CARTESIAN_POINT('Ctrl Pts',(43.6995308303616,23.4375000027312,105.5));
#9831=CARTESIAN_POINT('Ctrl Pts',(1.93800355965069E-14,23.3750000027312,
105.5));
#9832=CARTESIAN_POINT('Ctrl Pts',(-43.6995308303616,23.3125000027312,105.5));
#9833=CARTESIAN_POINT('Ctrl Pts',(-74.5997654151808,23.2500000027312,74.5997654151808));
#9834=CARTESIAN_POINT('Ctrl Pts',(-105.5,23.1875000027312,43.6995308303616));
#9835=CARTESIAN_POINT('Ctrl Pts',(-105.5,23.1250000027312,0.));
#9836=CARTESIAN_POINT('Ctrl Pts',(-105.5,23.0625000027312,-43.6995308303615));
#9837=CARTESIAN_POINT('Ctrl Pts',(-74.5997654151808,23.0000000027312,-74.5997654151808));
#9838=CARTESIAN_POINT('Ctrl Pts',(-43.6995308303615,22.9375000027312,-105.5));
#9839=CARTESIAN_POINT('Ctrl Pts',(-6.46001186550229E-15,22.8750000027312,
-105.5));
#9840=CARTESIAN_POINT('Ctrl Pts',(43.6995308303615,22.8125000027312,-105.5));
#9841=CARTESIAN_POINT('Ctrl Pts',(74.5997654151808,22.7500000027312,-74.5997654151808));
#9842=CARTESIAN_POINT('Ctrl Pts',(105.5,22.6875000027312,-43.6995308303616));
#9843=CARTESIAN_POINT('Ctrl Pts',(105.5,22.6250000027312,-1.29200237310046E-14));
#9844=CARTESIAN_POINT('Ctrl Pts',(105.5,22.5625000027312,43.6995308303615));
#9845=CARTESIAN_POINT('Ctrl Pts',(74.5997654151808,22.5000000027312,74.5997654151808));
#9846=CARTESIAN_POINT('Ctrl Pts',(43.6995308303616,22.4375000027312,105.5));
#9847=CARTESIAN_POINT('Ctrl Pts',(1.93800355965069E-14,22.3750000027312,
105.5));
#9848=CARTESIAN_POINT('Ctrl Pts',(-43.6995308303616,22.3125000027312,105.5));
#9849=CARTESIAN_POINT('Ctrl Pts',(-74.5997654151808,22.2500000027312,74.5997654151808));
#9850=CARTESIAN_POINT('Ctrl Pts',(-105.5,22.1875000027312,43.6995308303616));
#9851=CARTESIAN_POINT('Ctrl Pts',(-105.5,22.1250000027312,0.));
#9852=CARTESIAN_POINT('Ctrl Pts',(-105.5,22.0625000027312,-43.6995308303615));
#9853=CARTESIAN_POINT('Ctrl Pts',(-74.5997654151808,22.0000000027312,-74.5997654151808));
#9854=CARTESIAN_POINT('Ctrl Pts',(-43.6995308303615,21.9375000027312,-105.5));
#9855=CARTESIAN_POINT('Ctrl Pts',(-6.46001186550229E-15,21.8750000027312,
-105.5));
#9856=CARTESIAN_POINT('Ctrl Pts',(43.6995308303615,21.8125000027312,-105.5));
#9857=CARTESIAN_POINT('Ctrl Pts',(74.5997654151808,21.7500000027312,-74.5997654151808));
#9858=CARTESIAN_POINT('Ctrl Pts',(105.5,21.6875000027312,-43.6995308303616));
#9859=CARTESIAN_POINT('Ctrl Pts',(105.5,21.6250000027312,-1.29200237310046E-14));
#9860=CARTESIAN_POINT('Ctrl Pts',(105.5,21.5625000027312,43.6995308303615));
#9861=CARTESIAN_POINT('Ctrl Pts',(74.5997654151808,21.5000000027312,74.5997654151808));
#9862=CARTESIAN_POINT('Ctrl Pts',(43.6995308303616,21.4375000027312,105.5));
#9863=CARTESIAN_POINT('Ctrl Pts',(1.93800355965069E-14,21.3750000027312,
105.5));
#9864=CARTESIAN_POINT('Ctrl Pts',(-43.6995308303616,21.3125000027312,105.5));
#9865=CARTESIAN_POINT('Ctrl Pts',(-74.5997654151808,21.2500000027312,74.5997654151808));
#9866=CARTESIAN_POINT('Ctrl Pts',(-105.5,21.1875000027312,43.6995308303616));
#9867=CARTESIAN_POINT('Ctrl Pts',(-105.5,21.1250000027312,0.));
#9868=CARTESIAN_POINT('Ctrl Pts',(-105.5,21.0625000027312,-43.6995308303615));
#9869=CARTESIAN_POINT('Ctrl Pts',(-74.5997654151808,21.0000000027312,-74.5997654151808));
#9870=CARTESIAN_POINT('Ctrl Pts',(-43.6995308303615,20.9375000027312,-105.5));
#9871=CARTESIAN_POINT('Ctrl Pts',(-6.46001186550229E-15,20.8750000027312,
-105.5));
#9872=CARTESIAN_POINT('Ctrl Pts',(43.6995308303615,20.8125000027312,-105.5));
#9873=CARTESIAN_POINT('Ctrl Pts',(74.5997654151808,20.7500000027312,-74.5997654151808));
#9874=CARTESIAN_POINT('Ctrl Pts',(105.5,20.6875000027312,-43.6995308303616));
#9875=CARTESIAN_POINT('Ctrl Pts',(105.5,20.6250000027312,-1.29200237310046E-14));
#9876=CARTESIAN_POINT('Ctrl Pts',(105.5,20.5625000027312,43.6995308303615));
#9877=CARTESIAN_POINT('Ctrl Pts',(74.5997654151808,20.5000000027312,74.5997654151808));
#9878=CARTESIAN_POINT('Ctrl Pts',(43.6995308303616,20.4375000027312,105.5));
#9879=CARTESIAN_POINT('Ctrl Pts',(1.93800355965069E-14,20.3750000027312,
105.5));
#9880=CARTESIAN_POINT('Ctrl Pts',(-43.6995308303616,20.3125000027312,105.5));
#9881=CARTESIAN_POINT('Ctrl Pts',(-74.5997654151808,20.2500000027312,74.5997654151808));
#9882=CARTESIAN_POINT('Ctrl Pts',(-105.5,20.1875000027312,43.6995308303616));
#9883=CARTESIAN_POINT('Ctrl Pts',(-105.5,20.1250000027312,0.));
#9884=CARTESIAN_POINT('Ctrl Pts',(-105.5,20.0625000027312,-43.6995308303615));
#9885=CARTESIAN_POINT('Ctrl Pts',(-74.5997654151808,20.0000000027312,-74.5997654151808));
#9886=CARTESIAN_POINT('Ctrl Pts',(-43.6995308303615,19.9375000027312,-105.5));
#9887=CARTESIAN_POINT('Ctrl Pts',(-6.46001186550229E-15,19.8750000027312,
-105.5));
#9888=CARTESIAN_POINT('Ctrl Pts',(43.6995308303615,19.8125000027312,-105.5));
#9889=CARTESIAN_POINT('Ctrl Pts',(74.5997654151808,19.7500000027312,-74.5997654151808));
#9890=CARTESIAN_POINT('Ctrl Pts',(105.5,19.6875000027312,-43.6995308303616));
#9891=CARTESIAN_POINT('Ctrl Pts',(105.5,19.6250000027312,-1.29200237310046E-14));
#9892=CARTESIAN_POINT('Ctrl Pts',(105.5,19.5625000027312,43.6995308303615));
#9893=CARTESIAN_POINT('Ctrl Pts',(74.5997654151808,19.5000000027312,74.5997654151808));
#9894=CARTESIAN_POINT('Ctrl Pts',(43.6995308303616,19.4375000027312,105.5));
#9895=CARTESIAN_POINT('Ctrl Pts',(1.93800355965069E-14,19.3750000027312,
105.5));
#9896=CARTESIAN_POINT('Ctrl Pts',(-43.6995308303616,19.3125000027312,105.5));
#9897=CARTESIAN_POINT('Ctrl Pts',(-74.5997654151808,19.2500000027312,74.5997654151808));
#9898=CARTESIAN_POINT('Ctrl Pts',(-105.5,19.1875000027312,43.6995308303616));
#9899=CARTESIAN_POINT('Ctrl Pts',(-105.5,19.1250000027312,0.));
#9900=CARTESIAN_POINT('Ctrl Pts',(-105.5,19.0625000027312,-43.6995308303615));
#9901=CARTESIAN_POINT('Ctrl Pts',(-74.5997654151808,19.0000000027312,-74.5997654151808));
#9902=CARTESIAN_POINT('Ctrl Pts',(-43.6995308303615,18.9375000027312,-105.5));
#9903=CARTESIAN_POINT('Ctrl Pts',(-6.46001186550229E-15,18.8750000027312,
-105.5));
#9904=CARTESIAN_POINT('Ctrl Pts',(43.6995308303615,18.8125000027312,-105.5));
#9905=CARTESIAN_POINT('Ctrl Pts',(74.5997654151808,18.7500000027312,-74.5997654151808));
#9906=CARTESIAN_POINT('Ctrl Pts',(105.5,18.6875000027312,-43.6995308303616));
#9907=CARTESIAN_POINT('Ctrl Pts',(105.5,18.6250000027312,-1.29200237310046E-14));
#9908=CARTESIAN_POINT('Ctrl Pts',(105.5,18.5625000027312,43.6995308303615));
#9909=CARTESIAN_POINT('Ctrl Pts',(74.5997654151808,18.5000000027312,74.5997654151808));
#9910=CARTESIAN_POINT('Ctrl Pts',(43.6995308303616,18.4375000027312,105.5));
#9911=CARTESIAN_POINT('Ctrl Pts',(1.93800355965069E-14,18.3750000027312,
105.5));
#9912=CARTESIAN_POINT('Ctrl Pts',(-43.6995308303616,18.3125000027312,105.5));
#9913=CARTESIAN_POINT('Ctrl Pts',(-74.5997654151808,18.2500000027312,74.5997654151808));
#9914=CARTESIAN_POINT('Ctrl Pts',(-105.5,18.1875000027312,43.6995308303616));
#9915=CARTESIAN_POINT('Ctrl Pts',(-105.5,18.1250000027312,0.));
#9916=CARTESIAN_POINT('Ctrl Pts',(-105.5,18.0625000027312,-43.6995308303615));
#9917=CARTESIAN_POINT('Ctrl Pts',(-74.5997654151808,18.0000000027312,-74.5997654151808));
#9918=CARTESIAN_POINT('Ctrl Pts',(-43.6995308303615,17.9375000027312,-105.5));
#9919=CARTESIAN_POINT('Ctrl Pts',(-6.46001186550229E-15,17.8750000027312,
-105.5));
#9920=CARTESIAN_POINT('Ctrl Pts',(43.6995308303615,17.8125000027312,-105.5));
#9921=CARTESIAN_POINT('Ctrl Pts',(74.5997654151808,17.7500000027312,-74.5997654151808));
#9922=CARTESIAN_POINT('Ctrl Pts',(105.5,17.6875000027312,-43.6995308303616));
#9923=CARTESIAN_POINT('Ctrl Pts',(105.5,17.6250000027312,-1.29200237310046E-14));
#9924=CARTESIAN_POINT('Ctrl Pts',(105.5,17.5625000027312,43.6995308303615));
#9925=CARTESIAN_POINT('Ctrl Pts',(74.5997654151808,17.5000000027312,74.5997654151808));
#9926=CARTESIAN_POINT('Ctrl Pts',(43.6995308303616,17.4375000027312,105.5));
#9927=CARTESIAN_POINT('Ctrl Pts',(1.93800355965069E-14,17.3750000027312,
105.5));
#9928=CARTESIAN_POINT('Ctrl Pts',(-43.6995308303616,17.3125000027312,105.5));
#9929=CARTESIAN_POINT('Ctrl Pts',(-74.5997654151808,17.2500000027312,74.5997654151808));
#9930=CARTESIAN_POINT('Ctrl Pts',(-105.5,17.1875000027312,43.6995308303616));
#9931=CARTESIAN_POINT('Ctrl Pts',(-105.5,17.1250000027312,0.));
#9932=CARTESIAN_POINT('Ctrl Pts',(-105.5,17.0625000027312,-43.6995308303615));
#9933=CARTESIAN_POINT('Ctrl Pts',(-74.5997654151808,17.0000000027312,-74.5997654151808));
#9934=CARTESIAN_POINT('Ctrl Pts',(-43.6995308303615,16.9375000027312,-105.5));
#9935=CARTESIAN_POINT('Ctrl Pts',(-6.46001186550229E-15,16.8750000027312,
-105.5));
#9936=CARTESIAN_POINT('Ctrl Pts',(43.6995308303615,16.8125000027312,-105.5));
#9937=CARTESIAN_POINT('Ctrl Pts',(74.5997654151808,16.7500000027312,-74.5997654151808));
#9938=CARTESIAN_POINT('Ctrl Pts',(105.5,16.6875000027312,-43.6995308303616));
#9939=CARTESIAN_POINT('Ctrl Pts',(105.5,16.6250000027312,-1.29200237310046E-14));
#9940=CARTESIAN_POINT('Ctrl Pts',(105.5,16.5625000027312,43.6995308303615));
#9941=CARTESIAN_POINT('Ctrl Pts',(74.5997654151808,16.5000000027312,74.5997654151808));
#9942=CARTESIAN_POINT('Ctrl Pts',(43.6995308303616,16.4375000027312,105.5));
#9943=CARTESIAN_POINT('Ctrl Pts',(1.93800355965069E-14,16.3750000027312,
105.5));
#9944=CARTESIAN_POINT('Ctrl Pts',(-43.6995308303616,16.3125000027312,105.5));
#9945=CARTESIAN_POINT('Ctrl Pts',(-74.5997654151808,16.2500000027312,74.5997654151808));
#9946=CARTESIAN_POINT('Ctrl Pts',(-105.5,16.1875000027312,43.6995308303616));
#9947=CARTESIAN_POINT('Ctrl Pts',(-105.5,16.1250000027312,0.));
#9948=CARTESIAN_POINT('Ctrl Pts',(-105.5,16.0625000027312,-43.6995308303615));
#9949=CARTESIAN_POINT('Ctrl Pts',(-74.5997654151808,16.0000000027312,-74.5997654151808));
#9950=CARTESIAN_POINT('Ctrl Pts',(-43.6995308303615,15.9375000027312,-105.5));
#9951=CARTESIAN_POINT('Ctrl Pts',(-6.46001186550229E-15,15.8750000027312,
-105.5));
#9952=CARTESIAN_POINT('Ctrl Pts',(43.6995308303615,15.8125000027312,-105.5));
#9953=CARTESIAN_POINT('Ctrl Pts',(74.5997654151808,15.7500000027312,-74.5997654151808));
#9954=CARTESIAN_POINT('Ctrl Pts',(105.5,15.6875000027312,-43.6995308303616));
#9955=CARTESIAN_POINT('Ctrl Pts',(105.5,15.6250000027312,-1.29200237310046E-14));
#9956=CARTESIAN_POINT('Ctrl Pts',(105.5,15.5625000027312,43.6995308303615));
#9957=CARTESIAN_POINT('Ctrl Pts',(74.5997654151808,15.5000000027312,74.5997654151808));
#9958=CARTESIAN_POINT('Ctrl Pts',(43.6995308303616,15.4375000027312,105.5));
#9959=CARTESIAN_POINT('Ctrl Pts',(1.93800355965069E-14,15.3750000027312,
105.5));
#9960=CARTESIAN_POINT('Ctrl Pts',(-43.6995308303616,15.3125000027312,105.5));
#9961=CARTESIAN_POINT('Ctrl Pts',(-74.5997654151808,15.2500000027312,74.5997654151808));
#9962=CARTESIAN_POINT('Ctrl Pts',(-105.5,15.1875000027312,43.6995308303616));
#9963=CARTESIAN_POINT('Ctrl Pts',(-105.5,15.1250000027312,0.));
#9964=CARTESIAN_POINT('Ctrl Pts',(-105.5,15.0625000027312,-43.6995308303615));
#9965=CARTESIAN_POINT('Ctrl Pts',(-74.5997654151808,15.0000000027312,-74.5997654151808));
#9966=CARTESIAN_POINT('Ctrl Pts',(-43.6995308303615,14.9375000027312,-105.5));
#9967=CARTESIAN_POINT('Ctrl Pts',(-6.46001186550229E-15,14.8750000027312,
-105.5));
#9968=CARTESIAN_POINT('Ctrl Pts',(43.6995308303615,14.8125000027312,-105.5));
#9969=CARTESIAN_POINT('Ctrl Pts',(74.5997654151808,14.7500000027312,-74.5997654151808));
#9970=CARTESIAN_POINT('Ctrl Pts',(105.5,14.6875000027312,-43.6995308303616));
#9971=CARTESIAN_POINT('Ctrl Pts',(105.5,14.6250000027312,-1.29200237310046E-14));
#9972=CARTESIAN_POINT('Ctrl Pts',(105.5,14.5625000027312,43.6995308303615));
#9973=CARTESIAN_POINT('Ctrl Pts',(74.5997654151808,14.5000000027312,74.5997654151808));
#9974=CARTESIAN_POINT('Ctrl Pts',(43.6995308303616,14.4375000027312,105.5));
#9975=CARTESIAN_POINT('Ctrl Pts',(1.93800355965069E-14,14.3750000027312,
105.5));
#9976=CARTESIAN_POINT('Ctrl Pts',(-43.6995308303616,14.3125000027312,105.5));
#9977=CARTESIAN_POINT('Ctrl Pts',(-74.5997654151808,14.2500000027312,74.5997654151808));
#9978=CARTESIAN_POINT('Ctrl Pts',(-105.5,14.1875000027312,43.6995308303616));
#9979=CARTESIAN_POINT('Ctrl Pts',(-105.5,14.1250000027312,0.));
#9980=CARTESIAN_POINT('Ctrl Pts',(-105.5,14.0625000027312,-43.6995308303615));
#9981=CARTESIAN_POINT('Ctrl Pts',(-74.5997654151808,14.0000000027312,-74.5997654151808));
#9982=CARTESIAN_POINT('Ctrl Pts',(-43.6995308303615,13.9375000027312,-105.5));
#9983=CARTESIAN_POINT('Ctrl Pts',(-6.46001186550229E-15,13.8750000027312,
-105.5));
#9984=CARTESIAN_POINT('Ctrl Pts',(43.6995308303615,13.8125000027312,-105.5));
#9985=CARTESIAN_POINT('Ctrl Pts',(74.5997654151808,13.7500000027312,-74.5997654151808));
#9986=CARTESIAN_POINT('Ctrl Pts',(105.5,13.6875000027312,-43.6995308303616));
#9987=CARTESIAN_POINT('Ctrl Pts',(105.5,13.6250000027312,-1.29200237310046E-14));
#9988=CARTESIAN_POINT('Ctrl Pts',(105.5,13.5625000027312,43.6995308303615));
#9989=CARTESIAN_POINT('Ctrl Pts',(74.5997654151808,13.5000000027312,74.5997654151808));
#9990=CARTESIAN_POINT('Ctrl Pts',(43.6995308303616,13.4375000027312,105.5));
#9991=CARTESIAN_POINT('Ctrl Pts',(1.93800355965069E-14,13.3750000027312,
105.5));
#9992=CARTESIAN_POINT('Ctrl Pts',(-43.6995308303616,13.3125000027312,105.5));
#9993=CARTESIAN_POINT('Ctrl Pts',(-74.5997654151808,13.2500000027312,74.5997654151808));
#9994=CARTESIAN_POINT('Ctrl Pts',(-105.5,13.1875000027312,43.6995308303616));
#9995=CARTESIAN_POINT('Ctrl Pts',(-105.5,13.1250000027312,0.));
#9996=CARTESIAN_POINT('Ctrl Pts',(-105.5,13.0625000027312,-43.6995308303615));
#9997=CARTESIAN_POINT('Ctrl Pts',(-74.5997654151808,13.0000000027312,-74.5997654151808));
#9998=CARTESIAN_POINT('Ctrl Pts',(-43.6995308303615,12.9375000027312,-105.5));
#9999=CARTESIAN_POINT('Ctrl Pts',(-6.46001186550229E-15,12.8750000027312,
-105.5));
#10000=CARTESIAN_POINT('Ctrl Pts',(43.6995308303615,12.8125000027312,-105.5));
#10001=CARTESIAN_POINT('Ctrl Pts',(74.5997654151808,12.7500000027312,-74.5997654151808));
#10002=CARTESIAN_POINT('Ctrl Pts',(105.5,12.6875000027312,-43.6995308303616));
#10003=CARTESIAN_POINT('Ctrl Pts',(105.5,12.6250000027312,-1.29200237310046E-14));
#10004=CARTESIAN_POINT('Ctrl Pts',(105.5,12.5625000027312,43.6995308303615));
#10005=CARTESIAN_POINT('Ctrl Pts',(74.5997654151808,12.5000000027312,74.5997654151808));
#10006=CARTESIAN_POINT('Ctrl Pts',(43.6995308303616,12.4375000027312,105.5));
#10007=CARTESIAN_POINT('Ctrl Pts',(1.93800355965069E-14,12.3750000027312,
105.5));
#10008=CARTESIAN_POINT('Ctrl Pts',(-43.6995308303616,12.3125000027312,105.5));
#10009=CARTESIAN_POINT('Ctrl Pts',(-74.5997654151808,12.2500000027312,74.5997654151808));
#10010=CARTESIAN_POINT('Ctrl Pts',(-105.5,12.1875000027312,43.6995308303616));
#10011=CARTESIAN_POINT('Ctrl Pts',(-105.5,12.1250000027312,0.));
#10012=CARTESIAN_POINT('Ctrl Pts',(-105.5,12.0625000027312,-43.6995308303615));
#10013=CARTESIAN_POINT('Ctrl Pts',(-74.5997654151808,12.0000000027312,-74.5997654151808));
#10014=CARTESIAN_POINT('Ctrl Pts',(-43.6995308303615,11.9375000027312,-105.5));
#10015=CARTESIAN_POINT('Ctrl Pts',(-6.46001186550229E-15,11.8750000027312,
-105.5));
#10016=CARTESIAN_POINT('Ctrl Pts',(43.6995308303615,11.8125000027312,-105.5));
#10017=CARTESIAN_POINT('Ctrl Pts',(74.5997654151808,11.7500000027312,-74.5997654151808));
#10018=CARTESIAN_POINT('Ctrl Pts',(105.5,11.6875000027312,-43.6995308303616));
#10019=CARTESIAN_POINT('Ctrl Pts',(105.5,11.6250000027312,-1.29200237310046E-14));
#10020=CARTESIAN_POINT('Ctrl Pts',(105.5,11.5625000027312,43.6995308303615));
#10021=CARTESIAN_POINT('Ctrl Pts',(74.5997654151808,11.5000000027312,74.5997654151808));
#10022=CARTESIAN_POINT('Ctrl Pts',(43.6995308303616,11.4375000027312,105.5));
#10023=CARTESIAN_POINT('Ctrl Pts',(1.93800355965069E-14,11.3750000027312,
105.5));
#10024=CARTESIAN_POINT('Ctrl Pts',(-43.6995308303616,11.3125000027312,105.5));
#10025=CARTESIAN_POINT('Ctrl Pts',(-74.5997654151808,11.2500000027312,74.5997654151808));
#10026=CARTESIAN_POINT('Ctrl Pts',(-105.5,11.1875000027312,43.6995308303616));
#10027=CARTESIAN_POINT('Ctrl Pts',(-105.5,11.1250000027312,0.));
#10028=CARTESIAN_POINT('Ctrl Pts',(-105.5,11.0625000027312,-43.6995308303615));
#10029=CARTESIAN_POINT('Ctrl Pts',(-74.5997654151808,11.0000000027312,-74.5997654151808));
#10030=CARTESIAN_POINT('Ctrl Pts',(-43.6995308303615,10.9375000027312,-105.5));
#10031=CARTESIAN_POINT('Ctrl Pts',(-6.46001186550229E-15,10.8750000027312,
-105.5));
#10032=CARTESIAN_POINT('Ctrl Pts',(43.6995308303615,10.8125000027312,-105.5));
#10033=CARTESIAN_POINT('Ctrl Pts',(74.5997654151808,10.7500000027312,-74.5997654151808));
#10034=CARTESIAN_POINT('Ctrl Pts',(105.5,10.6875000027312,-43.6995308303616));
#10035=CARTESIAN_POINT('Ctrl Pts',(105.5,10.6250000027312,-1.29200237310046E-14));
#10036=CARTESIAN_POINT('Ctrl Pts',(105.5,10.5625000027312,43.6995308303615));
#10037=CARTESIAN_POINT('Ctrl Pts',(74.5997654151808,10.5000000027312,74.5997654151808));
#10038=CARTESIAN_POINT('Ctrl Pts',(43.6995308303616,10.4375000027312,105.5));
#10039=CARTESIAN_POINT('Ctrl Pts',(1.93800355965069E-14,10.3750000027312,
105.5));
#10040=CARTESIAN_POINT('Ctrl Pts',(-43.6995308303616,10.3125000027312,105.5));
#10041=CARTESIAN_POINT('Ctrl Pts',(-74.5997654151808,10.2500000027312,74.5997654151808));
#10042=CARTESIAN_POINT('Ctrl Pts',(-105.5,10.1875000027312,43.6995308303616));
#10043=CARTESIAN_POINT('Ctrl Pts',(-105.5,10.1250000027312,0.));
#10044=CARTESIAN_POINT('Ctrl Pts',(-105.5,10.0625000027312,-43.6995308303615));
#10045=CARTESIAN_POINT('Ctrl Pts',(-74.5997654151808,10.0000000027312,-74.5997654151808));
#10046=CARTESIAN_POINT('Ctrl Pts',(-43.6995308303615,9.93750000273118,-105.5));
#10047=CARTESIAN_POINT('Ctrl Pts',(-6.46001186550229E-15,9.87500000273118,
-105.5));
#10048=CARTESIAN_POINT('Ctrl Pts',(43.6995308303615,9.81250000273118,-105.5));
#10049=CARTESIAN_POINT('Ctrl Pts',(74.5997654151808,9.75000000273118,-74.5997654151808));
#10050=CARTESIAN_POINT('Ctrl Pts',(105.5,9.68750000273118,-43.6995308303616));
#10051=CARTESIAN_POINT('Ctrl Pts',(105.5,9.62500000273118,-1.29200237310046E-14));
#10052=CARTESIAN_POINT('Ctrl Pts',(105.5,9.56250000273118,43.6995308303615));
#10053=CARTESIAN_POINT('Ctrl Pts',(74.5997654151808,9.50000000273118,74.5997654151808));
#10054=CARTESIAN_POINT('Ctrl Pts',(43.6995308303616,9.43750000273118,105.5));
#10055=CARTESIAN_POINT('Ctrl Pts',(1.93800355965069E-14,9.37500000273118,
105.5));
#10056=CARTESIAN_POINT('Ctrl Pts',(-43.6995308303616,9.31250000273118,105.5));
#10057=CARTESIAN_POINT('Ctrl Pts',(-74.5997654151808,9.25000000273118,74.5997654151808));
#10058=CARTESIAN_POINT('Ctrl Pts',(-105.5,9.18750000273118,43.6995308303616));
#10059=CARTESIAN_POINT('Ctrl Pts',(-105.5,9.12500000273118,0.));
#10060=CARTESIAN_POINT('Ctrl Pts',(-105.5,9.06250000273118,-43.6995308303615));
#10061=CARTESIAN_POINT('Ctrl Pts',(-74.5997654151808,9.00000000273118,-74.5997654151808));
#10062=CARTESIAN_POINT('Ctrl Pts',(-43.6995308303615,8.93750000273118,-105.5));
#10063=CARTESIAN_POINT('Ctrl Pts',(-6.46001186550229E-15,8.87500000273118,
-105.5));
#10064=CARTESIAN_POINT('Ctrl Pts',(43.6995308303615,8.81250000273118,-105.5));
#10065=CARTESIAN_POINT('Ctrl Pts',(74.5997654151808,8.75000000273118,-74.5997654151808));
#10066=CARTESIAN_POINT('Ctrl Pts',(105.5,8.68750000273118,-43.6995308303616));
#10067=CARTESIAN_POINT('Ctrl Pts',(105.5,8.62500000273118,-1.29200237310046E-14));
#10068=CARTESIAN_POINT('Ctrl Pts',(105.5,8.56250000273118,43.6995308303615));
#10069=CARTESIAN_POINT('Ctrl Pts',(74.5997654151808,8.50000000273118,74.5997654151808));
#10070=CARTESIAN_POINT('Ctrl Pts',(43.6995308303616,8.43750000273118,105.5));
#10071=CARTESIAN_POINT('Ctrl Pts',(1.93800355965069E-14,8.37500000273118,
105.5));
#10072=CARTESIAN_POINT('Ctrl Pts',(-43.6995308303616,8.31250000273118,105.5));
#10073=CARTESIAN_POINT('Ctrl Pts',(-74.5997654151808,8.25000000273118,74.5997654151808));
#10074=CARTESIAN_POINT('Ctrl Pts',(-105.5,8.18750000273118,43.6995308303616));
#10075=CARTESIAN_POINT('Ctrl Pts',(-105.5,8.12500000273118,0.));
#10076=CARTESIAN_POINT('Ctrl Pts',(-105.5,8.06250000273118,-43.6995308303615));
#10077=CARTESIAN_POINT('Ctrl Pts',(-74.5997654151808,8.00000000273118,-74.5997654151808));
#10078=CARTESIAN_POINT('Ctrl Pts',(-43.6995308303615,7.93750000273118,-105.5));
#10079=CARTESIAN_POINT('Ctrl Pts',(-6.46001186550229E-15,7.87500000273118,
-105.5));
#10080=CARTESIAN_POINT('Ctrl Pts',(43.6995308303615,7.81250000273118,-105.5));
#10081=CARTESIAN_POINT('Ctrl Pts',(74.5997654151808,7.75000000273118,-74.5997654151808));
#10082=CARTESIAN_POINT('Ctrl Pts',(105.5,7.68750000273118,-43.6995308303616));
#10083=CARTESIAN_POINT('Ctrl Pts',(105.5,7.62500000273118,-1.29200237310046E-14));
#10084=CARTESIAN_POINT('Ctrl Pts',(105.5,7.56250000273118,43.6995308303615));
#10085=CARTESIAN_POINT('Ctrl Pts',(74.5997654151808,7.50000000273118,74.5997654151808));
#10086=CARTESIAN_POINT('Ctrl Pts',(43.6995308303616,7.43750000273118,105.5));
#10087=CARTESIAN_POINT('Ctrl Pts',(1.93800355965069E-14,7.37500000273118,
105.5));
#10088=CARTESIAN_POINT('Ctrl Pts',(-43.6995308303616,7.31250000273118,105.5));
#10089=CARTESIAN_POINT('Ctrl Pts',(-74.5997654151808,7.25000000273118,74.5997654151808));
#10090=CARTESIAN_POINT('Ctrl Pts',(-105.5,7.18750000273118,43.6995308303616));
#10091=CARTESIAN_POINT('Ctrl Pts',(-105.5,7.12500000273118,0.));
#10092=CARTESIAN_POINT('Ctrl Pts',(-105.5,7.06250000273118,-43.6995308303615));
#10093=CARTESIAN_POINT('Ctrl Pts',(-74.5997654151808,7.00000000273118,-74.5997654151808));
#10094=CARTESIAN_POINT('Ctrl Pts',(-43.6995308303615,6.93750000273118,-105.5));
#10095=CARTESIAN_POINT('Ctrl Pts',(-6.46001186550229E-15,6.87500000273118,
-105.5));
#10096=CARTESIAN_POINT('Ctrl Pts',(43.6995308303615,6.81250000273118,-105.5));
#10097=CARTESIAN_POINT('Ctrl Pts',(74.5997654151808,6.75000000273118,-74.5997654151808));
#10098=CARTESIAN_POINT('Ctrl Pts',(105.5,6.68750000273118,-43.6995308303616));
#10099=CARTESIAN_POINT('Ctrl Pts',(105.5,6.62500000273118,-1.29200237310046E-14));
#10100=CARTESIAN_POINT('Ctrl Pts',(105.5,6.56250000273118,43.6995308303615));
#10101=CARTESIAN_POINT('Ctrl Pts',(74.5997654151808,6.50000000273118,74.5997654151808));
#10102=CARTESIAN_POINT('Ctrl Pts',(43.6995308303616,6.43750000273118,105.5));
#10103=CARTESIAN_POINT('Ctrl Pts',(1.93800355965069E-14,6.37500000273118,
105.5));
#10104=CARTESIAN_POINT('Ctrl Pts',(-43.6995308303616,6.31250000273118,105.5));
#10105=CARTESIAN_POINT('Ctrl Pts',(-74.5997654151808,6.25000000273118,74.5997654151808));
#10106=CARTESIAN_POINT('Ctrl Pts',(-105.5,6.18750000273117,43.6995308303616));
#10107=CARTESIAN_POINT('Ctrl Pts',(-105.5,6.12500000273117,0.));
#10108=CARTESIAN_POINT('Ctrl Pts',(-105.5,6.06250000273118,-43.6995308303615));
#10109=CARTESIAN_POINT('Ctrl Pts',(-74.5997654151808,6.00000000273118,-74.5997654151808));
#10110=CARTESIAN_POINT('Ctrl Pts',(-43.6995308303615,5.93750000273118,-105.5));
#10111=CARTESIAN_POINT('Ctrl Pts',(-6.46001186550229E-15,5.87500000273117,
-105.5));
#10112=CARTESIAN_POINT('Ctrl Pts',(43.6995308303615,5.81250000273117,-105.5));
#10113=CARTESIAN_POINT('Ctrl Pts',(74.5997654151808,5.75000000273118,-74.5997654151808));
#10114=CARTESIAN_POINT('Ctrl Pts',(105.5,5.68750000273117,-43.6995308303616));
#10115=CARTESIAN_POINT('Ctrl Pts',(105.5,5.62500000273117,-1.29200237310046E-14));
#10116=CARTESIAN_POINT('Ctrl Pts',(105.5,5.56250000273117,43.6995308303615));
#10117=CARTESIAN_POINT('Ctrl Pts',(74.5997654151808,5.50000000273117,74.5997654151808));
#10118=CARTESIAN_POINT('Ctrl Pts',(43.6995308303616,5.43750000273118,105.5));
#10119=CARTESIAN_POINT('Ctrl Pts',(1.93800355965069E-14,5.37500000273117,
105.5));
#10120=CARTESIAN_POINT('Ctrl Pts',(-43.6995308303616,5.31250000273117,105.5));
#10121=CARTESIAN_POINT('Ctrl Pts',(-74.5997654151808,5.25000000273117,74.5997654151808));
#10122=CARTESIAN_POINT('Ctrl Pts',(-105.5,5.18750000273117,43.6995308303616));
#10123=CARTESIAN_POINT('Ctrl Pts',(-105.5,5.12500000273118,0.));
#10124=CARTESIAN_POINT('Ctrl Pts',(-105.5,5.06250000273118,-43.6995308303615));
#10125=CARTESIAN_POINT('Ctrl Pts',(-74.5997654151808,5.00000000273118,-74.5997654151808));
#10126=CARTESIAN_POINT('Ctrl Pts',(-43.6995308303615,4.93750000273118,-105.5));
#10127=CARTESIAN_POINT('Ctrl Pts',(-6.46001186550229E-15,4.87500000273118,
-105.5));
#10128=CARTESIAN_POINT('Ctrl Pts',(43.6995308303615,4.81250000273118,-105.5));
#10129=CARTESIAN_POINT('Ctrl Pts',(74.5997654151808,4.75000000273118,-74.5997654151808));
#10130=CARTESIAN_POINT('Ctrl Pts',(105.5,4.68750000273118,-43.6995308303616));
#10131=CARTESIAN_POINT('Ctrl Pts',(105.5,4.62500000273118,-1.29200237310046E-14));
#10132=CARTESIAN_POINT('Ctrl Pts',(105.5,4.56250000273118,43.6995308303615));
#10133=CARTESIAN_POINT('Ctrl Pts',(74.5997654151808,4.50000000273118,74.5997654151808));
#10134=CARTESIAN_POINT('Ctrl Pts',(43.6995308303616,4.43750000273118,105.5));
#10135=CARTESIAN_POINT('Ctrl Pts',(1.93800355965069E-14,4.37500000273118,
105.5));
#10136=CARTESIAN_POINT('Ctrl Pts',(-43.6995308303616,4.31250000273118,105.5));
#10137=CARTESIAN_POINT('Ctrl Pts',(-74.5997654151808,4.25000000273118,74.5997654151808));
#10138=CARTESIAN_POINT('Ctrl Pts',(-105.5,4.18750000273118,43.6995308303616));
#10139=CARTESIAN_POINT('Ctrl Pts',(-105.5,4.12500000273118,0.));
#10140=CARTESIAN_POINT('Ctrl Pts',(-105.5,4.06250000273118,-43.6995308303615));
#10141=CARTESIAN_POINT('Ctrl Pts',(-74.5997654151808,4.00000000273118,-74.5997654151808));
#10142=CARTESIAN_POINT('Ctrl Pts',(-43.6995308303615,3.93750000273118,-105.5));
#10143=CARTESIAN_POINT('Ctrl Pts',(-6.46001186550229E-15,3.87500000273118,
-105.5));
#10144=CARTESIAN_POINT('Ctrl Pts',(43.6995308303615,3.81250000273118,-105.5));
#10145=CARTESIAN_POINT('Ctrl Pts',(74.5997654151808,3.75000000273118,-74.5997654151808));
#10146=CARTESIAN_POINT('Ctrl Pts',(105.5,3.68750000273118,-43.6995308303616));
#10147=CARTESIAN_POINT('Ctrl Pts',(105.5,3.62500000273118,-1.29200237310046E-14));
#10148=CARTESIAN_POINT('Ctrl Pts',(105.5,3.56250000273118,43.6995308303615));
#10149=CARTESIAN_POINT('Ctrl Pts',(74.5997654151808,3.50000000273118,74.5997654151808));
#10150=CARTESIAN_POINT('Ctrl Pts',(43.6995308303616,3.43750000273118,105.5));
#10151=CARTESIAN_POINT('Ctrl Pts',(1.93800355965069E-14,3.37500000273118,
105.5));
#10152=CARTESIAN_POINT('Ctrl Pts',(-43.6995308303616,3.31250000273118,105.5));
#10153=CARTESIAN_POINT('Ctrl Pts',(-74.5997654151808,3.25000000273118,74.5997654151808));
#10154=CARTESIAN_POINT('Ctrl Pts',(-105.5,3.18750000273118,43.6995308303616));
#10155=CARTESIAN_POINT('Ctrl Pts',(-105.5,3.12500000273118,0.));
#10156=CARTESIAN_POINT('Ctrl Pts',(-105.5,3.06250000273118,-43.6995308303615));
#10157=CARTESIAN_POINT('Ctrl Pts',(-74.5997654151808,3.00000000273118,-74.5997654151808));
#10158=CARTESIAN_POINT('Ctrl Pts',(-43.6995308303615,2.93750000273118,-105.5));
#10159=CARTESIAN_POINT('Ctrl Pts',(-6.46001186550229E-15,2.87500000273118,
-105.5));
#10160=CARTESIAN_POINT('Ctrl Pts',(43.6995308303615,2.81250000273118,-105.5));
#10161=CARTESIAN_POINT('Ctrl Pts',(74.5997654151808,2.75000000273118,-74.5997654151808));
#10162=CARTESIAN_POINT('Ctrl Pts',(105.5,2.68750000273118,-43.6995308303616));
#10163=CARTESIAN_POINT('Ctrl Pts',(105.5,2.62500000273118,-1.29200237310046E-14));
#10164=CARTESIAN_POINT('Ctrl Pts',(105.5,2.56250000273118,43.6995308303615));
#10165=CARTESIAN_POINT('Ctrl Pts',(74.5997654151808,2.50000000273118,74.5997654151808));
#10166=CARTESIAN_POINT('Ctrl Pts',(43.6995308303616,2.43750000273118,105.5));
#10167=CARTESIAN_POINT('Ctrl Pts',(1.93800355965069E-14,2.37500000273118,
105.5));
#10168=CARTESIAN_POINT('Ctrl Pts',(-43.6995308303616,2.31250000273118,105.5));
#10169=CARTESIAN_POINT('Ctrl Pts',(-74.5997654151808,2.25000000273118,74.5997654151808));
#10170=CARTESIAN_POINT('Ctrl Pts',(-105.5,2.18750000273118,43.6995308303616));
#10171=CARTESIAN_POINT('Ctrl Pts',(-105.5,2.12500000273118,0.));
#10172=CARTESIAN_POINT('Ctrl Pts',(-105.5,2.06250000273118,-43.6995308303615));
#10173=CARTESIAN_POINT('Ctrl Pts',(-74.5997654151808,2.00000000273118,-74.5997654151808));
#10174=CARTESIAN_POINT('Ctrl Pts',(-43.6995308303615,1.93750000273118,-105.5));
#10175=CARTESIAN_POINT('Ctrl Pts',(-6.46001186550229E-15,1.87500000273118,
-105.5));
#10176=CARTESIAN_POINT('Ctrl Pts',(43.6995308303615,1.81250000273118,-105.5));
#10177=CARTESIAN_POINT('Ctrl Pts',(74.5997654151808,1.75000000273118,-74.5997654151808));
#10178=CARTESIAN_POINT('Ctrl Pts',(105.5,1.68750000273118,-43.6995308303616));
#10179=CARTESIAN_POINT('Ctrl Pts',(105.5,1.62500000273118,-1.29200237310046E-14));
#10180=CARTESIAN_POINT('Ctrl Pts',(105.5,1.56250000273118,43.6995308303615));
#10181=CARTESIAN_POINT('Ctrl Pts',(74.5997654151808,1.50000000273118,74.5997654151808));
#10182=CARTESIAN_POINT('Ctrl Pts',(43.6995308303616,1.43750000273118,105.5));
#10183=CARTESIAN_POINT('Ctrl Pts',(1.93800355965069E-14,1.37500000273118,
105.5));
#10184=CARTESIAN_POINT('Ctrl Pts',(-43.6995308303616,1.31250000273118,105.5));
#10185=CARTESIAN_POINT('Ctrl Pts',(-74.5997654151808,1.25000000273118,74.5997654151808));
#10186=CARTESIAN_POINT('Ctrl Pts',(-105.5,1.18750000273118,43.6995308303616));
#10187=CARTESIAN_POINT('Ctrl Pts',(-105.5,1.12500000273118,0.));
#10188=CARTESIAN_POINT('Ctrl Pts',(-105.5,1.06250000273118,-43.6995308303615));
#10189=CARTESIAN_POINT('Ctrl Pts',(-74.5997654151808,1.00000000273118,-74.5997654151808));
#10190=CARTESIAN_POINT('Ctrl Pts',(-43.6995308303615,0.937500002731177,
-105.5));
#10191=CARTESIAN_POINT('Ctrl Pts',(-6.46001186550229E-15,0.875000002731177,
-105.5));
#10192=CARTESIAN_POINT('Ctrl Pts',(43.6995308303615,0.812500002731177,-105.5));
#10193=CARTESIAN_POINT('Ctrl Pts',(74.5997654151808,0.750000002731177,-74.5997654151808));
#10194=CARTESIAN_POINT('Ctrl Pts',(105.5,0.687500002731177,-43.6995308303616));
#10195=CARTESIAN_POINT('Ctrl Pts',(105.5,0.625000002731177,-1.29200237310046E-14));
#10196=CARTESIAN_POINT('Ctrl Pts',(105.5,0.562500002731177,43.6995308303615));
#10197=CARTESIAN_POINT('Ctrl Pts',(74.5997654151808,0.500000002731177,74.5997654151808));
#10198=CARTESIAN_POINT('Ctrl Pts',(43.6995308303616,0.437500002731177,105.5));
#10199=CARTESIAN_POINT('Ctrl Pts',(1.93800355965069E-14,0.375000002731177,
105.5));
#10200=CARTESIAN_POINT('Ctrl Pts',(-43.6995308303616,0.312500002731177,
105.5));
#10201=CARTESIAN_POINT('Ctrl Pts',(-74.5997654151808,0.250000002731177,
74.5997654151808));
#10202=CARTESIAN_POINT('Ctrl Pts',(-105.5,0.187500002731177,43.6995308303616));
#10203=CARTESIAN_POINT('Ctrl Pts',(-105.5,0.125000002731177,0.));
#10204=CARTESIAN_POINT('Ctrl Pts',(-105.5,0.0625000027311765,-43.6995308303615));
#10205=CARTESIAN_POINT('Ctrl Pts',(-74.5997654151808,2.7311763961535E-9,
-74.5997654151808));
#10206=CARTESIAN_POINT('Ctrl Pts',(-43.6995308303615,-0.0624999972688237,
-105.5));
#10207=CARTESIAN_POINT('Ctrl Pts',(-6.46001186550229E-15,-0.124999997268824,
-105.5));
#10208=CARTESIAN_POINT('Ctrl Pts',(43.6995308303615,-0.187499997268824,
-105.5));
#10209=CARTESIAN_POINT('Ctrl Pts',(74.5997654151808,-0.249999997268824,
-74.5997654151808));
#10210=CARTESIAN_POINT('Ctrl Pts',(105.5,-0.312499997268824,-43.6995308303616));
#10211=CARTESIAN_POINT('Ctrl Pts',(105.5,-0.374999997268824,-1.29200237310046E-14));
#10212=CARTESIAN_POINT('Ctrl Pts',(105.5,-0.437499997268824,43.6995308303615));
#10213=CARTESIAN_POINT('Ctrl Pts',(74.5997654151808,-0.499999997268824,
74.5997654151808));
#10214=CARTESIAN_POINT('Ctrl Pts',(43.6995308303616,-0.562499997268824,
105.5));
#10215=CARTESIAN_POINT('Ctrl Pts',(1.93800355965069E-14,-0.624999997268824,
105.5));
#10216=CARTESIAN_POINT('Ctrl Pts',(-43.6995308303616,-0.687499997268824,
105.5));
#10217=CARTESIAN_POINT('Ctrl Pts',(-74.5997654151808,-0.749999997268824,
74.5997654151808));
#10218=CARTESIAN_POINT('Ctrl Pts',(-105.5,-0.812499997268824,43.6995308303616));
#10219=CARTESIAN_POINT('Ctrl Pts',(-105.5,-0.874999997268824,0.));
#10220=CARTESIAN_POINT('Ctrl Pts',(-104.958734125,49.4375000013656,0.));
#10221=CARTESIAN_POINT('Ctrl Pts',(-104.958734125,49.3750000013656,-43.4753311640868));
#10222=CARTESIAN_POINT('Ctrl Pts',(-74.2170326445434,49.3125000013656,-74.2170326445434));
#10223=CARTESIAN_POINT('Ctrl Pts',(-43.4753311640868,49.2500000013656,-104.958734125));
#10224=CARTESIAN_POINT('Ctrl Pts',(-6.42686888943697E-15,49.1875000013656,
-104.958734125));
#10225=CARTESIAN_POINT('Ctrl Pts',(43.4753311640868,49.1250000013656,-104.958734125));
#10226=CARTESIAN_POINT('Ctrl Pts',(74.2170326445434,49.0625000013656,-74.2170326445434));
#10227=CARTESIAN_POINT('Ctrl Pts',(104.958734125,49.0000000013656,-43.4753311640868));
#10228=CARTESIAN_POINT('Ctrl Pts',(104.958734125,48.9375000013656,-1.28537377788739E-14));
#10229=CARTESIAN_POINT('Ctrl Pts',(104.958734125,48.8750000013656,43.4753311640868));
#10230=CARTESIAN_POINT('Ctrl Pts',(74.2170326445434,48.8125000013656,74.2170326445434));
#10231=CARTESIAN_POINT('Ctrl Pts',(43.4753311640869,48.7500000013656,104.958734125));
#10232=CARTESIAN_POINT('Ctrl Pts',(1.92806066683109E-14,48.6875000013656,
104.958734125));
#10233=CARTESIAN_POINT('Ctrl Pts',(-43.4753311640868,48.6250000013656,104.958734125));
#10234=CARTESIAN_POINT('Ctrl Pts',(-74.2170326445434,48.5625000013656,74.2170326445434));
#10235=CARTESIAN_POINT('Ctrl Pts',(-104.958734125,48.5000000013656,43.4753311640869));
#10236=CARTESIAN_POINT('Ctrl Pts',(-104.958734125,48.4375000013656,0.));
#10237=CARTESIAN_POINT('Ctrl Pts',(-104.958734125,48.3750000013656,-43.4753311640868));
#10238=CARTESIAN_POINT('Ctrl Pts',(-74.2170326445434,48.3125000013656,-74.2170326445434));
#10239=CARTESIAN_POINT('Ctrl Pts',(-43.4753311640868,48.2500000013656,-104.958734125));
#10240=CARTESIAN_POINT('Ctrl Pts',(-6.42686888943697E-15,48.1875000013656,
-104.958734125));
#10241=CARTESIAN_POINT('Ctrl Pts',(43.4753311640868,48.1250000013656,-104.958734125));
#10242=CARTESIAN_POINT('Ctrl Pts',(74.2170326445434,48.0625000013656,-74.2170326445434));
#10243=CARTESIAN_POINT('Ctrl Pts',(104.958734125,48.0000000013656,-43.4753311640868));
#10244=CARTESIAN_POINT('Ctrl Pts',(104.958734125,47.9375000013656,-1.28537377788739E-14));
#10245=CARTESIAN_POINT('Ctrl Pts',(104.958734125,47.8750000013656,43.4753311640868));
#10246=CARTESIAN_POINT('Ctrl Pts',(74.2170326445434,47.8125000013656,74.2170326445434));
#10247=CARTESIAN_POINT('Ctrl Pts',(43.4753311640869,47.7500000013656,104.958734125));
#10248=CARTESIAN_POINT('Ctrl Pts',(1.92806066683109E-14,47.6875000013656,
104.958734125));
#10249=CARTESIAN_POINT('Ctrl Pts',(-43.4753311640868,47.6250000013656,104.958734125));
#10250=CARTESIAN_POINT('Ctrl Pts',(-74.2170326445434,47.5625000013656,74.2170326445434));
#10251=CARTESIAN_POINT('Ctrl Pts',(-104.958734125,47.5000000013656,43.4753311640869));
#10252=CARTESIAN_POINT('Ctrl Pts',(-104.958734125,47.4375000013656,0.));
#10253=CARTESIAN_POINT('Ctrl Pts',(-104.958734125,47.3750000013656,-43.4753311640868));
#10254=CARTESIAN_POINT('Ctrl Pts',(-74.2170326445434,47.3125000013656,-74.2170326445434));
#10255=CARTESIAN_POINT('Ctrl Pts',(-43.4753311640868,47.2500000013656,-104.958734125));
#10256=CARTESIAN_POINT('Ctrl Pts',(-6.42686888943697E-15,47.1875000013656,
-104.958734125));
#10257=CARTESIAN_POINT('Ctrl Pts',(43.4753311640868,47.1250000013656,-104.958734125));
#10258=CARTESIAN_POINT('Ctrl Pts',(74.2170326445434,47.0625000013656,-74.2170326445434));
#10259=CARTESIAN_POINT('Ctrl Pts',(104.958734125,47.0000000013656,-43.4753311640868));
#10260=CARTESIAN_POINT('Ctrl Pts',(104.958734125,46.9375000013656,-1.28537377788739E-14));
#10261=CARTESIAN_POINT('Ctrl Pts',(104.958734125,46.8750000013656,43.4753311640868));
#10262=CARTESIAN_POINT('Ctrl Pts',(74.2170326445434,46.8125000013656,74.2170326445434));
#10263=CARTESIAN_POINT('Ctrl Pts',(43.4753311640869,46.7500000013656,104.958734125));
#10264=CARTESIAN_POINT('Ctrl Pts',(1.92806066683109E-14,46.6875000013656,
104.958734125));
#10265=CARTESIAN_POINT('Ctrl Pts',(-43.4753311640868,46.6250000013656,104.958734125));
#10266=CARTESIAN_POINT('Ctrl Pts',(-74.2170326445434,46.5625000013656,74.2170326445434));
#10267=CARTESIAN_POINT('Ctrl Pts',(-104.958734125,46.5000000013656,43.4753311640869));
#10268=CARTESIAN_POINT('Ctrl Pts',(-104.958734125,46.4375000013656,0.));
#10269=CARTESIAN_POINT('Ctrl Pts',(-104.958734125,46.3750000013656,-43.4753311640868));
#10270=CARTESIAN_POINT('Ctrl Pts',(-74.2170326445434,46.3125000013656,-74.2170326445434));
#10271=CARTESIAN_POINT('Ctrl Pts',(-43.4753311640868,46.2500000013656,-104.958734125));
#10272=CARTESIAN_POINT('Ctrl Pts',(-6.42686888943697E-15,46.1875000013656,
-104.958734125));
#10273=CARTESIAN_POINT('Ctrl Pts',(43.4753311640868,46.1250000013656,-104.958734125));
#10274=CARTESIAN_POINT('Ctrl Pts',(74.2170326445434,46.0625000013656,-74.2170326445434));
#10275=CARTESIAN_POINT('Ctrl Pts',(104.958734125,46.0000000013656,-43.4753311640868));
#10276=CARTESIAN_POINT('Ctrl Pts',(104.958734125,45.9375000013656,-1.28537377788739E-14));
#10277=CARTESIAN_POINT('Ctrl Pts',(104.958734125,45.8750000013656,43.4753311640868));
#10278=CARTESIAN_POINT('Ctrl Pts',(74.2170326445434,45.8125000013656,74.2170326445434));
#10279=CARTESIAN_POINT('Ctrl Pts',(43.4753311640869,45.7500000013656,104.958734125));
#10280=CARTESIAN_POINT('Ctrl Pts',(1.92806066683109E-14,45.6875000013656,
104.958734125));
#10281=CARTESIAN_POINT('Ctrl Pts',(-43.4753311640868,45.6250000013656,104.958734125));
#10282=CARTESIAN_POINT('Ctrl Pts',(-74.2170326445434,45.5625000013656,74.2170326445434));
#10283=CARTESIAN_POINT('Ctrl Pts',(-104.958734125,45.5000000013656,43.4753311640869));
#10284=CARTESIAN_POINT('Ctrl Pts',(-104.958734125,45.4375000013656,0.));
#10285=CARTESIAN_POINT('Ctrl Pts',(-104.958734125,45.3750000013656,-43.4753311640868));
#10286=CARTESIAN_POINT('Ctrl Pts',(-74.2170326445434,45.3125000013656,-74.2170326445434));
#10287=CARTESIAN_POINT('Ctrl Pts',(-43.4753311640868,45.2500000013656,-104.958734125));
#10288=CARTESIAN_POINT('Ctrl Pts',(-6.42686888943697E-15,45.1875000013656,
-104.958734125));
#10289=CARTESIAN_POINT('Ctrl Pts',(43.4753311640868,45.1250000013656,-104.958734125));
#10290=CARTESIAN_POINT('Ctrl Pts',(74.2170326445434,45.0625000013656,-74.2170326445434));
#10291=CARTESIAN_POINT('Ctrl Pts',(104.958734125,45.0000000013656,-43.4753311640868));
#10292=CARTESIAN_POINT('Ctrl Pts',(104.958734125,44.9375000013656,-1.28537377788739E-14));
#10293=CARTESIAN_POINT('Ctrl Pts',(104.958734125,44.8750000013656,43.4753311640868));
#10294=CARTESIAN_POINT('Ctrl Pts',(74.2170326445434,44.8125000013656,74.2170326445434));
#10295=CARTESIAN_POINT('Ctrl Pts',(43.4753311640869,44.7500000013656,104.958734125));
#10296=CARTESIAN_POINT('Ctrl Pts',(1.92806066683109E-14,44.6875000013656,
104.958734125));
#10297=CARTESIAN_POINT('Ctrl Pts',(-43.4753311640868,44.6250000013656,104.958734125));
#10298=CARTESIAN_POINT('Ctrl Pts',(-74.2170326445434,44.5625000013656,74.2170326445434));
#10299=CARTESIAN_POINT('Ctrl Pts',(-104.958734125,44.5000000013656,43.4753311640869));
#10300=CARTESIAN_POINT('Ctrl Pts',(-104.958734125,44.4375000013656,0.));
#10301=CARTESIAN_POINT('Ctrl Pts',(-104.958734125,44.3750000013656,-43.4753311640868));
#10302=CARTESIAN_POINT('Ctrl Pts',(-74.2170326445434,44.3125000013656,-74.2170326445434));
#10303=CARTESIAN_POINT('Ctrl Pts',(-43.4753311640868,44.2500000013656,-104.958734125));
#10304=CARTESIAN_POINT('Ctrl Pts',(-6.42686888943697E-15,44.1875000013656,
-104.958734125));
#10305=CARTESIAN_POINT('Ctrl Pts',(43.4753311640868,44.1250000013656,-104.958734125));
#10306=CARTESIAN_POINT('Ctrl Pts',(74.2170326445434,44.0625000013656,-74.2170326445434));
#10307=CARTESIAN_POINT('Ctrl Pts',(104.958734125,44.0000000013656,-43.4753311640868));
#10308=CARTESIAN_POINT('Ctrl Pts',(104.958734125,43.9375000013656,-1.28537377788739E-14));
#10309=CARTESIAN_POINT('Ctrl Pts',(104.958734125,43.8750000013656,43.4753311640868));
#10310=CARTESIAN_POINT('Ctrl Pts',(74.2170326445434,43.8125000013656,74.2170326445434));
#10311=CARTESIAN_POINT('Ctrl Pts',(43.4753311640869,43.7500000013656,104.958734125));
#10312=CARTESIAN_POINT('Ctrl Pts',(1.92806066683109E-14,43.6875000013656,
104.958734125));
#10313=CARTESIAN_POINT('Ctrl Pts',(-43.4753311640868,43.6250000013656,104.958734125));
#10314=CARTESIAN_POINT('Ctrl Pts',(-74.2170326445434,43.5625000013656,74.2170326445434));
#10315=CARTESIAN_POINT('Ctrl Pts',(-104.958734125,43.5000000013656,43.4753311640869));
#10316=CARTESIAN_POINT('Ctrl Pts',(-104.958734125,43.4375000013656,0.));
#10317=CARTESIAN_POINT('Ctrl Pts',(-104.958734125,43.3750000013656,-43.4753311640868));
#10318=CARTESIAN_POINT('Ctrl Pts',(-74.2170326445434,43.3125000013656,-74.2170326445434));
#10319=CARTESIAN_POINT('Ctrl Pts',(-43.4753311640868,43.2500000013656,-104.958734125));
#10320=CARTESIAN_POINT('Ctrl Pts',(-6.42686888943697E-15,43.1875000013656,
-104.958734125));
#10321=CARTESIAN_POINT('Ctrl Pts',(43.4753311640868,43.1250000013656,-104.958734125));
#10322=CARTESIAN_POINT('Ctrl Pts',(74.2170326445434,43.0625000013656,-74.2170326445434));
#10323=CARTESIAN_POINT('Ctrl Pts',(104.958734125,43.0000000013656,-43.4753311640868));
#10324=CARTESIAN_POINT('Ctrl Pts',(104.958734125,42.9375000013656,-1.28537377788739E-14));
#10325=CARTESIAN_POINT('Ctrl Pts',(104.958734125,42.8750000013656,43.4753311640868));
#10326=CARTESIAN_POINT('Ctrl Pts',(74.2170326445434,42.8125000013656,74.2170326445434));
#10327=CARTESIAN_POINT('Ctrl Pts',(43.4753311640869,42.7500000013656,104.958734125));
#10328=CARTESIAN_POINT('Ctrl Pts',(1.92806066683109E-14,42.6875000013656,
104.958734125));
#10329=CARTESIAN_POINT('Ctrl Pts',(-43.4753311640868,42.6250000013656,104.958734125));
#10330=CARTESIAN_POINT('Ctrl Pts',(-74.2170326445434,42.5625000013656,74.2170326445434));
#10331=CARTESIAN_POINT('Ctrl Pts',(-104.958734125,42.5000000013656,43.4753311640869));
#10332=CARTESIAN_POINT('Ctrl Pts',(-104.958734125,42.4375000013656,0.));
#10333=CARTESIAN_POINT('Ctrl Pts',(-104.958734125,42.3750000013656,-43.4753311640868));
#10334=CARTESIAN_POINT('Ctrl Pts',(-74.2170326445434,42.3125000013656,-74.2170326445434));
#10335=CARTESIAN_POINT('Ctrl Pts',(-43.4753311640868,42.2500000013656,-104.958734125));
#10336=CARTESIAN_POINT('Ctrl Pts',(-6.42686888943697E-15,42.1875000013656,
-104.958734125));
#10337=CARTESIAN_POINT('Ctrl Pts',(43.4753311640868,42.1250000013656,-104.958734125));
#10338=CARTESIAN_POINT('Ctrl Pts',(74.2170326445434,42.0625000013656,-74.2170326445434));
#10339=CARTESIAN_POINT('Ctrl Pts',(104.958734125,42.0000000013656,-43.4753311640868));
#10340=CARTESIAN_POINT('Ctrl Pts',(104.958734125,41.9375000013656,-1.28537377788739E-14));
#10341=CARTESIAN_POINT('Ctrl Pts',(104.958734125,41.8750000013656,43.4753311640868));
#10342=CARTESIAN_POINT('Ctrl Pts',(74.2170326445434,41.8125000013656,74.2170326445434));
#10343=CARTESIAN_POINT('Ctrl Pts',(43.4753311640869,41.7500000013656,104.958734125));
#10344=CARTESIAN_POINT('Ctrl Pts',(1.92806066683109E-14,41.6875000013656,
104.958734125));
#10345=CARTESIAN_POINT('Ctrl Pts',(-43.4753311640868,41.6250000013656,104.958734125));
#10346=CARTESIAN_POINT('Ctrl Pts',(-74.2170326445434,41.5625000013656,74.2170326445434));
#10347=CARTESIAN_POINT('Ctrl Pts',(-104.958734125,41.5000000013656,43.4753311640869));
#10348=CARTESIAN_POINT('Ctrl Pts',(-104.958734125,41.4375000013656,0.));
#10349=CARTESIAN_POINT('Ctrl Pts',(-104.958734125,41.3750000013656,-43.4753311640868));
#10350=CARTESIAN_POINT('Ctrl Pts',(-74.2170326445434,41.3125000013656,-74.2170326445434));
#10351=CARTESIAN_POINT('Ctrl Pts',(-43.4753311640868,41.2500000013656,-104.958734125));
#10352=CARTESIAN_POINT('Ctrl Pts',(-6.42686888943697E-15,41.1875000013656,
-104.958734125));
#10353=CARTESIAN_POINT('Ctrl Pts',(43.4753311640868,41.1250000013656,-104.958734125));
#10354=CARTESIAN_POINT('Ctrl Pts',(74.2170326445434,41.0625000013656,-74.2170326445434));
#10355=CARTESIAN_POINT('Ctrl Pts',(104.958734125,41.0000000013656,-43.4753311640868));
#10356=CARTESIAN_POINT('Ctrl Pts',(104.958734125,40.9375000013656,-1.28537377788739E-14));
#10357=CARTESIAN_POINT('Ctrl Pts',(104.958734125,40.8750000013656,43.4753311640868));
#10358=CARTESIAN_POINT('Ctrl Pts',(74.2170326445434,40.8125000013656,74.2170326445434));
#10359=CARTESIAN_POINT('Ctrl Pts',(43.4753311640869,40.7500000013656,104.958734125));
#10360=CARTESIAN_POINT('Ctrl Pts',(1.92806066683109E-14,40.6875000013656,
104.958734125));
#10361=CARTESIAN_POINT('Ctrl Pts',(-43.4753311640868,40.6250000013656,104.958734125));
#10362=CARTESIAN_POINT('Ctrl Pts',(-74.2170326445434,40.5625000013656,74.2170326445434));
#10363=CARTESIAN_POINT('Ctrl Pts',(-104.958734125,40.5000000013656,43.4753311640869));
#10364=CARTESIAN_POINT('Ctrl Pts',(-104.958734125,40.4375000013656,0.));
#10365=CARTESIAN_POINT('Ctrl Pts',(-104.958734125,40.3750000013656,-43.4753311640868));
#10366=CARTESIAN_POINT('Ctrl Pts',(-74.2170326445434,40.3125000013656,-74.2170326445434));
#10367=CARTESIAN_POINT('Ctrl Pts',(-43.4753311640868,40.2500000013656,-104.958734125));
#10368=CARTESIAN_POINT('Ctrl Pts',(-6.42686888943697E-15,40.1875000013656,
-104.958734125));
#10369=CARTESIAN_POINT('Ctrl Pts',(43.4753311640868,40.1250000013656,-104.958734125));
#10370=CARTESIAN_POINT('Ctrl Pts',(74.2170326445434,40.0625000013656,-74.2170326445434));
#10371=CARTESIAN_POINT('Ctrl Pts',(104.958734125,40.0000000013656,-43.4753311640868));
#10372=CARTESIAN_POINT('Ctrl Pts',(104.958734125,39.9375000013656,-1.28537377788739E-14));
#10373=CARTESIAN_POINT('Ctrl Pts',(104.958734125,39.8750000013656,43.4753311640868));
#10374=CARTESIAN_POINT('Ctrl Pts',(74.2170326445434,39.8125000013656,74.2170326445434));
#10375=CARTESIAN_POINT('Ctrl Pts',(43.4753311640869,39.7500000013656,104.958734125));
#10376=CARTESIAN_POINT('Ctrl Pts',(1.92806066683109E-14,39.6875000013656,
104.958734125));
#10377=CARTESIAN_POINT('Ctrl Pts',(-43.4753311640868,39.6250000013656,104.958734125));
#10378=CARTESIAN_POINT('Ctrl Pts',(-74.2170326445434,39.5625000013656,74.2170326445434));
#10379=CARTESIAN_POINT('Ctrl Pts',(-104.958734125,39.5000000013656,43.4753311640869));
#10380=CARTESIAN_POINT('Ctrl Pts',(-104.958734125,39.4375000013656,0.));
#10381=CARTESIAN_POINT('Ctrl Pts',(-104.958734125,39.3750000013656,-43.4753311640868));
#10382=CARTESIAN_POINT('Ctrl Pts',(-74.2170326445434,39.3125000013656,-74.2170326445434));
#10383=CARTESIAN_POINT('Ctrl Pts',(-43.4753311640868,39.2500000013656,-104.958734125));
#10384=CARTESIAN_POINT('Ctrl Pts',(-6.42686888943697E-15,39.1875000013656,
-104.958734125));
#10385=CARTESIAN_POINT('Ctrl Pts',(43.4753311640868,39.1250000013656,-104.958734125));
#10386=CARTESIAN_POINT('Ctrl Pts',(74.2170326445434,39.0625000013656,-74.2170326445434));
#10387=CARTESIAN_POINT('Ctrl Pts',(104.958734125,39.0000000013656,-43.4753311640868));
#10388=CARTESIAN_POINT('Ctrl Pts',(104.958734125,38.9375000013656,-1.28537377788739E-14));
#10389=CARTESIAN_POINT('Ctrl Pts',(104.958734125,38.8750000013656,43.4753311640868));
#10390=CARTESIAN_POINT('Ctrl Pts',(74.2170326445434,38.8125000013656,74.2170326445434));
#10391=CARTESIAN_POINT('Ctrl Pts',(43.4753311640869,38.7500000013656,104.958734125));
#10392=CARTESIAN_POINT('Ctrl Pts',(1.92806066683109E-14,38.6875000013656,
104.958734125));
#10393=CARTESIAN_POINT('Ctrl Pts',(-43.4753311640868,38.6250000013656,104.958734125));
#10394=CARTESIAN_POINT('Ctrl Pts',(-74.2170326445434,38.5625000013656,74.2170326445434));
#10395=CARTESIAN_POINT('Ctrl Pts',(-104.958734125,38.5000000013656,43.4753311640869));
#10396=CARTESIAN_POINT('Ctrl Pts',(-104.958734125,38.4375000013656,0.));
#10397=CARTESIAN_POINT('Ctrl Pts',(-104.958734125,38.3750000013656,-43.4753311640868));
#10398=CARTESIAN_POINT('Ctrl Pts',(-74.2170326445434,38.3125000013656,-74.2170326445434));
#10399=CARTESIAN_POINT('Ctrl Pts',(-43.4753311640868,38.2500000013656,-104.958734125));
#10400=CARTESIAN_POINT('Ctrl Pts',(-6.42686888943697E-15,38.1875000013656,
-104.958734125));
#10401=CARTESIAN_POINT('Ctrl Pts',(43.4753311640868,38.1250000013656,-104.958734125));
#10402=CARTESIAN_POINT('Ctrl Pts',(74.2170326445434,38.0625000013656,-74.2170326445434));
#10403=CARTESIAN_POINT('Ctrl Pts',(104.958734125,38.0000000013656,-43.4753311640868));
#10404=CARTESIAN_POINT('Ctrl Pts',(104.958734125,37.9375000013656,-1.28537377788739E-14));
#10405=CARTESIAN_POINT('Ctrl Pts',(104.958734125,37.8750000013656,43.4753311640868));
#10406=CARTESIAN_POINT('Ctrl Pts',(74.2170326445434,37.8125000013656,74.2170326445434));
#10407=CARTESIAN_POINT('Ctrl Pts',(43.4753311640869,37.7500000013656,104.958734125));
#10408=CARTESIAN_POINT('Ctrl Pts',(1.92806066683109E-14,37.6875000013656,
104.958734125));
#10409=CARTESIAN_POINT('Ctrl Pts',(-43.4753311640868,37.6250000013656,104.958734125));
#10410=CARTESIAN_POINT('Ctrl Pts',(-74.2170326445434,37.5625000013656,74.2170326445434));
#10411=CARTESIAN_POINT('Ctrl Pts',(-104.958734125,37.5000000013656,43.4753311640869));
#10412=CARTESIAN_POINT('Ctrl Pts',(-104.958734125,37.4375000013656,0.));
#10413=CARTESIAN_POINT('Ctrl Pts',(-104.958734125,37.3750000013656,-43.4753311640868));
#10414=CARTESIAN_POINT('Ctrl Pts',(-74.2170326445434,37.3125000013656,-74.2170326445434));
#10415=CARTESIAN_POINT('Ctrl Pts',(-43.4753311640868,37.2500000013656,-104.958734125));
#10416=CARTESIAN_POINT('Ctrl Pts',(-6.42686888943697E-15,37.1875000013656,
-104.958734125));
#10417=CARTESIAN_POINT('Ctrl Pts',(43.4753311640868,37.1250000013656,-104.958734125));
#10418=CARTESIAN_POINT('Ctrl Pts',(74.2170326445434,37.0625000013656,-74.2170326445434));
#10419=CARTESIAN_POINT('Ctrl Pts',(104.958734125,37.0000000013656,-43.4753311640868));
#10420=CARTESIAN_POINT('Ctrl Pts',(104.958734125,36.9375000013656,-1.28537377788739E-14));
#10421=CARTESIAN_POINT('Ctrl Pts',(104.958734125,36.8750000013656,43.4753311640868));
#10422=CARTESIAN_POINT('Ctrl Pts',(74.2170326445434,36.8125000013656,74.2170326445434));
#10423=CARTESIAN_POINT('Ctrl Pts',(43.4753311640869,36.7500000013656,104.958734125));
#10424=CARTESIAN_POINT('Ctrl Pts',(1.92806066683109E-14,36.6875000013656,
104.958734125));
#10425=CARTESIAN_POINT('Ctrl Pts',(-43.4753311640868,36.6250000013656,104.958734125));
#10426=CARTESIAN_POINT('Ctrl Pts',(-74.2170326445434,36.5625000013656,74.2170326445434));
#10427=CARTESIAN_POINT('Ctrl Pts',(-104.958734125,36.5000000013656,43.4753311640869));
#10428=CARTESIAN_POINT('Ctrl Pts',(-104.958734125,36.4375000013656,0.));
#10429=CARTESIAN_POINT('Ctrl Pts',(-104.958734125,36.3750000013656,-43.4753311640868));
#10430=CARTESIAN_POINT('Ctrl Pts',(-74.2170326445434,36.3125000013656,-74.2170326445434));
#10431=CARTESIAN_POINT('Ctrl Pts',(-43.4753311640868,36.2500000013656,-104.958734125));
#10432=CARTESIAN_POINT('Ctrl Pts',(-6.42686888943697E-15,36.1875000013656,
-104.958734125));
#10433=CARTESIAN_POINT('Ctrl Pts',(43.4753311640868,36.1250000013656,-104.958734125));
#10434=CARTESIAN_POINT('Ctrl Pts',(74.2170326445434,36.0625000013656,-74.2170326445434));
#10435=CARTESIAN_POINT('Ctrl Pts',(104.958734125,36.0000000013656,-43.4753311640868));
#10436=CARTESIAN_POINT('Ctrl Pts',(104.958734125,35.9375000013656,-1.28537377788739E-14));
#10437=CARTESIAN_POINT('Ctrl Pts',(104.958734125,35.8750000013656,43.4753311640868));
#10438=CARTESIAN_POINT('Ctrl Pts',(74.2170326445434,35.8125000013656,74.2170326445434));
#10439=CARTESIAN_POINT('Ctrl Pts',(43.4753311640869,35.7500000013656,104.958734125));
#10440=CARTESIAN_POINT('Ctrl Pts',(1.92806066683109E-14,35.6875000013656,
104.958734125));
#10441=CARTESIAN_POINT('Ctrl Pts',(-43.4753311640868,35.6250000013656,104.958734125));
#10442=CARTESIAN_POINT('Ctrl Pts',(-74.2170326445434,35.5625000013656,74.2170326445434));
#10443=CARTESIAN_POINT('Ctrl Pts',(-104.958734125,35.5000000013656,43.4753311640869));
#10444=CARTESIAN_POINT('Ctrl Pts',(-104.958734125,35.4375000013656,0.));
#10445=CARTESIAN_POINT('Ctrl Pts',(-104.958734125,35.3750000013656,-43.4753311640868));
#10446=CARTESIAN_POINT('Ctrl Pts',(-74.2170326445434,35.3125000013656,-74.2170326445434));
#10447=CARTESIAN_POINT('Ctrl Pts',(-43.4753311640868,35.2500000013656,-104.958734125));
#10448=CARTESIAN_POINT('Ctrl Pts',(-6.42686888943697E-15,35.1875000013656,
-104.958734125));
#10449=CARTESIAN_POINT('Ctrl Pts',(43.4753311640868,35.1250000013656,-104.958734125));
#10450=CARTESIAN_POINT('Ctrl Pts',(74.2170326445434,35.0625000013656,-74.2170326445434));
#10451=CARTESIAN_POINT('Ctrl Pts',(104.958734125,35.0000000013656,-43.4753311640868));
#10452=CARTESIAN_POINT('Ctrl Pts',(104.958734125,34.9375000013656,-1.28537377788739E-14));
#10453=CARTESIAN_POINT('Ctrl Pts',(104.958734125,34.8750000013656,43.4753311640868));
#10454=CARTESIAN_POINT('Ctrl Pts',(74.2170326445434,34.8125000013656,74.2170326445434));
#10455=CARTESIAN_POINT('Ctrl Pts',(43.4753311640869,34.7500000013656,104.958734125));
#10456=CARTESIAN_POINT('Ctrl Pts',(1.92806066683109E-14,34.6875000013656,
104.958734125));
#10457=CARTESIAN_POINT('Ctrl Pts',(-43.4753311640868,34.6250000013656,104.958734125));
#10458=CARTESIAN_POINT('Ctrl Pts',(-74.2170326445434,34.5625000013656,74.2170326445434));
#10459=CARTESIAN_POINT('Ctrl Pts',(-104.958734125,34.5000000013656,43.4753311640869));
#10460=CARTESIAN_POINT('Ctrl Pts',(-104.958734125,34.4375000013656,0.));
#10461=CARTESIAN_POINT('Ctrl Pts',(-104.958734125,34.3750000013656,-43.4753311640868));
#10462=CARTESIAN_POINT('Ctrl Pts',(-74.2170326445434,34.3125000013656,-74.2170326445434));
#10463=CARTESIAN_POINT('Ctrl Pts',(-43.4753311640868,34.2500000013656,-104.958734125));
#10464=CARTESIAN_POINT('Ctrl Pts',(-6.42686888943697E-15,34.1875000013656,
-104.958734125));
#10465=CARTESIAN_POINT('Ctrl Pts',(43.4753311640868,34.1250000013656,-104.958734125));
#10466=CARTESIAN_POINT('Ctrl Pts',(74.2170326445434,34.0625000013656,-74.2170326445434));
#10467=CARTESIAN_POINT('Ctrl Pts',(104.958734125,34.0000000013656,-43.4753311640868));
#10468=CARTESIAN_POINT('Ctrl Pts',(104.958734125,33.9375000013656,-1.28537377788739E-14));
#10469=CARTESIAN_POINT('Ctrl Pts',(104.958734125,33.8750000013656,43.4753311640868));
#10470=CARTESIAN_POINT('Ctrl Pts',(74.2170326445434,33.8125000013656,74.2170326445434));
#10471=CARTESIAN_POINT('Ctrl Pts',(43.4753311640869,33.7500000013656,104.958734125));
#10472=CARTESIAN_POINT('Ctrl Pts',(1.92806066683109E-14,33.6875000013656,
104.958734125));
#10473=CARTESIAN_POINT('Ctrl Pts',(-43.4753311640868,33.6250000013656,104.958734125));
#10474=CARTESIAN_POINT('Ctrl Pts',(-74.2170326445434,33.5625000013656,74.2170326445434));
#10475=CARTESIAN_POINT('Ctrl Pts',(-104.958734125,33.5000000013656,43.4753311640869));
#10476=CARTESIAN_POINT('Ctrl Pts',(-104.958734125,33.4375000013656,0.));
#10477=CARTESIAN_POINT('Ctrl Pts',(-104.958734125,33.3750000013656,-43.4753311640868));
#10478=CARTESIAN_POINT('Ctrl Pts',(-74.2170326445434,33.3125000013656,-74.2170326445434));
#10479=CARTESIAN_POINT('Ctrl Pts',(-43.4753311640868,33.2500000013656,-104.958734125));
#10480=CARTESIAN_POINT('Ctrl Pts',(-6.42686888943697E-15,33.1875000013656,
-104.958734125));
#10481=CARTESIAN_POINT('Ctrl Pts',(43.4753311640868,33.1250000013656,-104.958734125));
#10482=CARTESIAN_POINT('Ctrl Pts',(74.2170326445434,33.0625000013656,-74.2170326445434));
#10483=CARTESIAN_POINT('Ctrl Pts',(104.958734125,33.0000000013656,-43.4753311640868));
#10484=CARTESIAN_POINT('Ctrl Pts',(104.958734125,32.9375000013656,-1.28537377788739E-14));
#10485=CARTESIAN_POINT('Ctrl Pts',(104.958734125,32.8750000013656,43.4753311640868));
#10486=CARTESIAN_POINT('Ctrl Pts',(74.2170326445434,32.8125000013656,74.2170326445434));
#10487=CARTESIAN_POINT('Ctrl Pts',(43.4753311640869,32.7500000013656,104.958734125));
#10488=CARTESIAN_POINT('Ctrl Pts',(1.92806066683109E-14,32.6875000013656,
104.958734125));
#10489=CARTESIAN_POINT('Ctrl Pts',(-43.4753311640868,32.6250000013656,104.958734125));
#10490=CARTESIAN_POINT('Ctrl Pts',(-74.2170326445434,32.5625000013656,74.2170326445434));
#10491=CARTESIAN_POINT('Ctrl Pts',(-104.958734125,32.5000000013656,43.4753311640869));
#10492=CARTESIAN_POINT('Ctrl Pts',(-104.958734125,32.4375000013656,0.));
#10493=CARTESIAN_POINT('Ctrl Pts',(-104.958734125,32.3750000013656,-43.4753311640868));
#10494=CARTESIAN_POINT('Ctrl Pts',(-74.2170326445434,32.3125000013656,-74.2170326445434));
#10495=CARTESIAN_POINT('Ctrl Pts',(-43.4753311640868,32.2500000013656,-104.958734125));
#10496=CARTESIAN_POINT('Ctrl Pts',(-6.42686888943697E-15,32.1875000013656,
-104.958734125));
#10497=CARTESIAN_POINT('Ctrl Pts',(43.4753311640868,32.1250000013656,-104.958734125));
#10498=CARTESIAN_POINT('Ctrl Pts',(74.2170326445434,32.0625000013656,-74.2170326445434));
#10499=CARTESIAN_POINT('Ctrl Pts',(104.958734125,32.0000000013656,-43.4753311640868));
#10500=CARTESIAN_POINT('Ctrl Pts',(104.958734125,31.9375000013656,-1.28537377788739E-14));
#10501=CARTESIAN_POINT('Ctrl Pts',(104.958734125,31.8750000013656,43.4753311640868));
#10502=CARTESIAN_POINT('Ctrl Pts',(74.2170326445434,31.8125000013656,74.2170326445434));
#10503=CARTESIAN_POINT('Ctrl Pts',(43.4753311640869,31.7500000013656,104.958734125));
#10504=CARTESIAN_POINT('Ctrl Pts',(1.92806066683109E-14,31.6875000013656,
104.958734125));
#10505=CARTESIAN_POINT('Ctrl Pts',(-43.4753311640868,31.6250000013656,104.958734125));
#10506=CARTESIAN_POINT('Ctrl Pts',(-74.2170326445434,31.5625000013656,74.2170326445434));
#10507=CARTESIAN_POINT('Ctrl Pts',(-104.958734125,31.5000000013656,43.4753311640869));
#10508=CARTESIAN_POINT('Ctrl Pts',(-104.958734125,31.4375000013656,0.));
#10509=CARTESIAN_POINT('Ctrl Pts',(-104.958734125,31.3750000013656,-43.4753311640868));
#10510=CARTESIAN_POINT('Ctrl Pts',(-74.2170326445434,31.3125000013656,-74.2170326445434));
#10511=CARTESIAN_POINT('Ctrl Pts',(-43.4753311640868,31.2500000013656,-104.958734125));
#10512=CARTESIAN_POINT('Ctrl Pts',(-6.42686888943697E-15,31.1875000013656,
-104.958734125));
#10513=CARTESIAN_POINT('Ctrl Pts',(43.4753311640868,31.1250000013656,-104.958734125));
#10514=CARTESIAN_POINT('Ctrl Pts',(74.2170326445434,31.0625000013656,-74.2170326445434));
#10515=CARTESIAN_POINT('Ctrl Pts',(104.958734125,31.0000000013656,-43.4753311640868));
#10516=CARTESIAN_POINT('Ctrl Pts',(104.958734125,30.9375000013656,-1.28537377788739E-14));
#10517=CARTESIAN_POINT('Ctrl Pts',(104.958734125,30.8750000013656,43.4753311640868));
#10518=CARTESIAN_POINT('Ctrl Pts',(74.2170326445434,30.8125000013656,74.2170326445434));
#10519=CARTESIAN_POINT('Ctrl Pts',(43.4753311640869,30.7500000013656,104.958734125));
#10520=CARTESIAN_POINT('Ctrl Pts',(1.92806066683109E-14,30.6875000013656,
104.958734125));
#10521=CARTESIAN_POINT('Ctrl Pts',(-43.4753311640868,30.6250000013656,104.958734125));
#10522=CARTESIAN_POINT('Ctrl Pts',(-74.2170326445434,30.5625000013656,74.2170326445434));
#10523=CARTESIAN_POINT('Ctrl Pts',(-104.958734125,30.5000000013656,43.4753311640869));
#10524=CARTESIAN_POINT('Ctrl Pts',(-104.958734125,30.4375000013656,0.));
#10525=CARTESIAN_POINT('Ctrl Pts',(-104.958734125,30.3750000013656,-43.4753311640868));
#10526=CARTESIAN_POINT('Ctrl Pts',(-74.2170326445434,30.3125000013656,-74.2170326445434));
#10527=CARTESIAN_POINT('Ctrl Pts',(-43.4753311640868,30.2500000013656,-104.958734125));
#10528=CARTESIAN_POINT('Ctrl Pts',(-6.42686888943697E-15,30.1875000013656,
-104.958734125));
#10529=CARTESIAN_POINT('Ctrl Pts',(43.4753311640868,30.1250000013656,-104.958734125));
#10530=CARTESIAN_POINT('Ctrl Pts',(74.2170326445434,30.0625000013656,-74.2170326445434));
#10531=CARTESIAN_POINT('Ctrl Pts',(104.958734125,30.0000000013656,-43.4753311640868));
#10532=CARTESIAN_POINT('Ctrl Pts',(104.958734125,29.9375000013656,-1.28537377788739E-14));
#10533=CARTESIAN_POINT('Ctrl Pts',(104.958734125,29.8750000013656,43.4753311640868));
#10534=CARTESIAN_POINT('Ctrl Pts',(74.2170326445434,29.8125000013656,74.2170326445434));
#10535=CARTESIAN_POINT('Ctrl Pts',(43.4753311640869,29.7500000013656,104.958734125));
#10536=CARTESIAN_POINT('Ctrl Pts',(1.92806066683109E-14,29.6875000013656,
104.958734125));
#10537=CARTESIAN_POINT('Ctrl Pts',(-43.4753311640868,29.6250000013656,104.958734125));
#10538=CARTESIAN_POINT('Ctrl Pts',(-74.2170326445434,29.5625000013656,74.2170326445434));
#10539=CARTESIAN_POINT('Ctrl Pts',(-104.958734125,29.5000000013656,43.4753311640869));
#10540=CARTESIAN_POINT('Ctrl Pts',(-104.958734125,29.4375000013656,0.));
#10541=CARTESIAN_POINT('Ctrl Pts',(-104.958734125,29.3750000013656,-43.4753311640868));
#10542=CARTESIAN_POINT('Ctrl Pts',(-74.2170326445434,29.3125000013656,-74.2170326445434));
#10543=CARTESIAN_POINT('Ctrl Pts',(-43.4753311640868,29.2500000013656,-104.958734125));
#10544=CARTESIAN_POINT('Ctrl Pts',(-6.42686888943697E-15,29.1875000013656,
-104.958734125));
#10545=CARTESIAN_POINT('Ctrl Pts',(43.4753311640868,29.1250000013656,-104.958734125));
#10546=CARTESIAN_POINT('Ctrl Pts',(74.2170326445434,29.0625000013656,-74.2170326445434));
#10547=CARTESIAN_POINT('Ctrl Pts',(104.958734125,29.0000000013656,-43.4753311640868));
#10548=CARTESIAN_POINT('Ctrl Pts',(104.958734125,28.9375000013656,-1.28537377788739E-14));
#10549=CARTESIAN_POINT('Ctrl Pts',(104.958734125,28.8750000013656,43.4753311640868));
#10550=CARTESIAN_POINT('Ctrl Pts',(74.2170326445434,28.8125000013656,74.2170326445434));
#10551=CARTESIAN_POINT('Ctrl Pts',(43.4753311640869,28.7500000013656,104.958734125));
#10552=CARTESIAN_POINT('Ctrl Pts',(1.92806066683109E-14,28.6875000013656,
104.958734125));
#10553=CARTESIAN_POINT('Ctrl Pts',(-43.4753311640868,28.6250000013656,104.958734125));
#10554=CARTESIAN_POINT('Ctrl Pts',(-74.2170326445434,28.5625000013656,74.2170326445434));
#10555=CARTESIAN_POINT('Ctrl Pts',(-104.958734125,28.5000000013656,43.4753311640869));
#10556=CARTESIAN_POINT('Ctrl Pts',(-104.958734125,28.4375000013656,0.));
#10557=CARTESIAN_POINT('Ctrl Pts',(-104.958734125,28.3750000013656,-43.4753311640868));
#10558=CARTESIAN_POINT('Ctrl Pts',(-74.2170326445434,28.3125000013656,-74.2170326445434));
#10559=CARTESIAN_POINT('Ctrl Pts',(-43.4753311640868,28.2500000013656,-104.958734125));
#10560=CARTESIAN_POINT('Ctrl Pts',(-6.42686888943697E-15,28.1875000013656,
-104.958734125));
#10561=CARTESIAN_POINT('Ctrl Pts',(43.4753311640868,28.1250000013656,-104.958734125));
#10562=CARTESIAN_POINT('Ctrl Pts',(74.2170326445434,28.0625000013656,-74.2170326445434));
#10563=CARTESIAN_POINT('Ctrl Pts',(104.958734125,28.0000000013656,-43.4753311640868));
#10564=CARTESIAN_POINT('Ctrl Pts',(104.958734125,27.9375000013656,-1.28537377788739E-14));
#10565=CARTESIAN_POINT('Ctrl Pts',(104.958734125,27.8750000013656,43.4753311640868));
#10566=CARTESIAN_POINT('Ctrl Pts',(74.2170326445434,27.8125000013656,74.2170326445434));
#10567=CARTESIAN_POINT('Ctrl Pts',(43.4753311640869,27.7500000013656,104.958734125));
#10568=CARTESIAN_POINT('Ctrl Pts',(1.92806066683109E-14,27.6875000013656,
104.958734125));
#10569=CARTESIAN_POINT('Ctrl Pts',(-43.4753311640868,27.6250000013656,104.958734125));
#10570=CARTESIAN_POINT('Ctrl Pts',(-74.2170326445434,27.5625000013656,74.2170326445434));
#10571=CARTESIAN_POINT('Ctrl Pts',(-104.958734125,27.5000000013656,43.4753311640869));
#10572=CARTESIAN_POINT('Ctrl Pts',(-104.958734125,27.4375000013656,0.));
#10573=CARTESIAN_POINT('Ctrl Pts',(-104.958734125,27.3750000013656,-43.4753311640868));
#10574=CARTESIAN_POINT('Ctrl Pts',(-74.2170326445434,27.3125000013656,-74.2170326445434));
#10575=CARTESIAN_POINT('Ctrl Pts',(-43.4753311640868,27.2500000013656,-104.958734125));
#10576=CARTESIAN_POINT('Ctrl Pts',(-6.42686888943697E-15,27.1875000013656,
-104.958734125));
#10577=CARTESIAN_POINT('Ctrl Pts',(43.4753311640868,27.1250000013656,-104.958734125));
#10578=CARTESIAN_POINT('Ctrl Pts',(74.2170326445434,27.0625000013656,-74.2170326445434));
#10579=CARTESIAN_POINT('Ctrl Pts',(104.958734125,27.0000000013656,-43.4753311640868));
#10580=CARTESIAN_POINT('Ctrl Pts',(104.958734125,26.9375000013656,-1.28537377788739E-14));
#10581=CARTESIAN_POINT('Ctrl Pts',(104.958734125,26.8750000013656,43.4753311640868));
#10582=CARTESIAN_POINT('Ctrl Pts',(74.2170326445434,26.8125000013656,74.2170326445434));
#10583=CARTESIAN_POINT('Ctrl Pts',(43.4753311640869,26.7500000013656,104.958734125));
#10584=CARTESIAN_POINT('Ctrl Pts',(1.92806066683109E-14,26.6875000013656,
104.958734125));
#10585=CARTESIAN_POINT('Ctrl Pts',(-43.4753311640868,26.6250000013656,104.958734125));
#10586=CARTESIAN_POINT('Ctrl Pts',(-74.2170326445434,26.5625000013656,74.2170326445434));
#10587=CARTESIAN_POINT('Ctrl Pts',(-104.958734125,26.5000000013656,43.4753311640869));
#10588=CARTESIAN_POINT('Ctrl Pts',(-104.958734125,26.4375000013656,0.));
#10589=CARTESIAN_POINT('Ctrl Pts',(-104.958734125,26.3750000013656,-43.4753311640868));
#10590=CARTESIAN_POINT('Ctrl Pts',(-74.2170326445434,26.3125000013656,-74.2170326445434));
#10591=CARTESIAN_POINT('Ctrl Pts',(-43.4753311640868,26.2500000013656,-104.958734125));
#10592=CARTESIAN_POINT('Ctrl Pts',(-6.42686888943697E-15,26.1875000013656,
-104.958734125));
#10593=CARTESIAN_POINT('Ctrl Pts',(43.4753311640868,26.1250000013656,-104.958734125));
#10594=CARTESIAN_POINT('Ctrl Pts',(74.2170326445434,26.0625000013656,-74.2170326445434));
#10595=CARTESIAN_POINT('Ctrl Pts',(104.958734125,26.0000000013656,-43.4753311640868));
#10596=CARTESIAN_POINT('Ctrl Pts',(104.958734125,25.9375000013656,-1.28537377788739E-14));
#10597=CARTESIAN_POINT('Ctrl Pts',(104.958734125,25.8750000013656,43.4753311640868));
#10598=CARTESIAN_POINT('Ctrl Pts',(74.2170326445434,25.8125000013656,74.2170326445434));
#10599=CARTESIAN_POINT('Ctrl Pts',(43.4753311640869,25.7500000013656,104.958734125));
#10600=CARTESIAN_POINT('Ctrl Pts',(1.92806066683109E-14,25.6875000013656,
104.958734125));
#10601=CARTESIAN_POINT('Ctrl Pts',(-43.4753311640868,25.6250000013656,104.958734125));
#10602=CARTESIAN_POINT('Ctrl Pts',(-74.2170326445434,25.5625000013656,74.2170326445434));
#10603=CARTESIAN_POINT('Ctrl Pts',(-104.958734125,25.5000000013656,43.4753311640869));
#10604=CARTESIAN_POINT('Ctrl Pts',(-104.958734125,25.4375000013656,0.));
#10605=CARTESIAN_POINT('Ctrl Pts',(-104.958734125,25.3750000013656,-43.4753311640868));
#10606=CARTESIAN_POINT('Ctrl Pts',(-74.2170326445434,25.3125000013656,-74.2170326445434));
#10607=CARTESIAN_POINT('Ctrl Pts',(-43.4753311640868,25.2500000013656,-104.958734125));
#10608=CARTESIAN_POINT('Ctrl Pts',(-6.42686888943697E-15,25.1875000013656,
-104.958734125));
#10609=CARTESIAN_POINT('Ctrl Pts',(43.4753311640868,25.1250000013656,-104.958734125));
#10610=CARTESIAN_POINT('Ctrl Pts',(74.2170326445434,25.0625000013656,-74.2170326445434));
#10611=CARTESIAN_POINT('Ctrl Pts',(104.958734125,25.0000000013656,-43.4753311640868));
#10612=CARTESIAN_POINT('Ctrl Pts',(104.958734125,24.9375000013656,-1.28537377788739E-14));
#10613=CARTESIAN_POINT('Ctrl Pts',(104.958734125,24.8750000013656,43.4753311640868));
#10614=CARTESIAN_POINT('Ctrl Pts',(74.2170326445434,24.8125000013656,74.2170326445434));
#10615=CARTESIAN_POINT('Ctrl Pts',(43.4753311640869,24.7500000013656,104.958734125));
#10616=CARTESIAN_POINT('Ctrl Pts',(1.92806066683109E-14,24.6875000013656,
104.958734125));
#10617=CARTESIAN_POINT('Ctrl Pts',(-43.4753311640868,24.6250000013656,104.958734125));
#10618=CARTESIAN_POINT('Ctrl Pts',(-74.2170326445434,24.5625000013656,74.2170326445434));
#10619=CARTESIAN_POINT('Ctrl Pts',(-104.958734125,24.5000000013656,43.4753311640869));
#10620=CARTESIAN_POINT('Ctrl Pts',(-104.958734125,24.4375000013656,0.));
#10621=CARTESIAN_POINT('Ctrl Pts',(-104.958734125,24.3750000013656,-43.4753311640868));
#10622=CARTESIAN_POINT('Ctrl Pts',(-74.2170326445434,24.3125000013656,-74.2170326445434));
#10623=CARTESIAN_POINT('Ctrl Pts',(-43.4753311640868,24.2500000013656,-104.958734125));
#10624=CARTESIAN_POINT('Ctrl Pts',(-6.42686888943697E-15,24.1875000013656,
-104.958734125));
#10625=CARTESIAN_POINT('Ctrl Pts',(43.4753311640868,24.1250000013656,-104.958734125));
#10626=CARTESIAN_POINT('Ctrl Pts',(74.2170326445434,24.0625000013656,-74.2170326445434));
#10627=CARTESIAN_POINT('Ctrl Pts',(104.958734125,24.0000000013656,-43.4753311640868));
#10628=CARTESIAN_POINT('Ctrl Pts',(104.958734125,23.9375000013656,-1.28537377788739E-14));
#10629=CARTESIAN_POINT('Ctrl Pts',(104.958734125,23.8750000013656,43.4753311640868));
#10630=CARTESIAN_POINT('Ctrl Pts',(74.2170326445434,23.8125000013656,74.2170326445434));
#10631=CARTESIAN_POINT('Ctrl Pts',(43.4753311640869,23.7500000013656,104.958734125));
#10632=CARTESIAN_POINT('Ctrl Pts',(1.92806066683109E-14,23.6875000013656,
104.958734125));
#10633=CARTESIAN_POINT('Ctrl Pts',(-43.4753311640868,23.6250000013656,104.958734125));
#10634=CARTESIAN_POINT('Ctrl Pts',(-74.2170326445434,23.5625000013656,74.2170326445434));
#10635=CARTESIAN_POINT('Ctrl Pts',(-104.958734125,23.5000000013656,43.4753311640869));
#10636=CARTESIAN_POINT('Ctrl Pts',(-104.958734125,23.4375000013656,0.));
#10637=CARTESIAN_POINT('Ctrl Pts',(-104.958734125,23.3750000013656,-43.4753311640868));
#10638=CARTESIAN_POINT('Ctrl Pts',(-74.2170326445434,23.3125000013656,-74.2170326445434));
#10639=CARTESIAN_POINT('Ctrl Pts',(-43.4753311640868,23.2500000013656,-104.958734125));
#10640=CARTESIAN_POINT('Ctrl Pts',(-6.42686888943697E-15,23.1875000013656,
-104.958734125));
#10641=CARTESIAN_POINT('Ctrl Pts',(43.4753311640868,23.1250000013656,-104.958734125));
#10642=CARTESIAN_POINT('Ctrl Pts',(74.2170326445434,23.0625000013656,-74.2170326445434));
#10643=CARTESIAN_POINT('Ctrl Pts',(104.958734125,23.0000000013656,-43.4753311640868));
#10644=CARTESIAN_POINT('Ctrl Pts',(104.958734125,22.9375000013656,-1.28537377788739E-14));
#10645=CARTESIAN_POINT('Ctrl Pts',(104.958734125,22.8750000013656,43.4753311640868));
#10646=CARTESIAN_POINT('Ctrl Pts',(74.2170326445434,22.8125000013656,74.2170326445434));
#10647=CARTESIAN_POINT('Ctrl Pts',(43.4753311640869,22.7500000013656,104.958734125));
#10648=CARTESIAN_POINT('Ctrl Pts',(1.92806066683109E-14,22.6875000013656,
104.958734125));
#10649=CARTESIAN_POINT('Ctrl Pts',(-43.4753311640868,22.6250000013656,104.958734125));
#10650=CARTESIAN_POINT('Ctrl Pts',(-74.2170326445434,22.5625000013656,74.2170326445434));
#10651=CARTESIAN_POINT('Ctrl Pts',(-104.958734125,22.5000000013656,43.4753311640869));
#10652=CARTESIAN_POINT('Ctrl Pts',(-104.958734125,22.4375000013656,0.));
#10653=CARTESIAN_POINT('Ctrl Pts',(-104.958734125,22.3750000013656,-43.4753311640868));
#10654=CARTESIAN_POINT('Ctrl Pts',(-74.2170326445434,22.3125000013656,-74.2170326445434));
#10655=CARTESIAN_POINT('Ctrl Pts',(-43.4753311640868,22.2500000013656,-104.958734125));
#10656=CARTESIAN_POINT('Ctrl Pts',(-6.42686888943697E-15,22.1875000013656,
-104.958734125));
#10657=CARTESIAN_POINT('Ctrl Pts',(43.4753311640868,22.1250000013656,-104.958734125));
#10658=CARTESIAN_POINT('Ctrl Pts',(74.2170326445434,22.0625000013656,-74.2170326445434));
#10659=CARTESIAN_POINT('Ctrl Pts',(104.958734125,22.0000000013656,-43.4753311640868));
#10660=CARTESIAN_POINT('Ctrl Pts',(104.958734125,21.9375000013656,-1.28537377788739E-14));
#10661=CARTESIAN_POINT('Ctrl Pts',(104.958734125,21.8750000013656,43.4753311640868));
#10662=CARTESIAN_POINT('Ctrl Pts',(74.2170326445434,21.8125000013656,74.2170326445434));
#10663=CARTESIAN_POINT('Ctrl Pts',(43.4753311640869,21.7500000013656,104.958734125));
#10664=CARTESIAN_POINT('Ctrl Pts',(1.92806066683109E-14,21.6875000013656,
104.958734125));
#10665=CARTESIAN_POINT('Ctrl Pts',(-43.4753311640868,21.6250000013656,104.958734125));
#10666=CARTESIAN_POINT('Ctrl Pts',(-74.2170326445434,21.5625000013656,74.2170326445434));
#10667=CARTESIAN_POINT('Ctrl Pts',(-104.958734125,21.5000000013656,43.4753311640869));
#10668=CARTESIAN_POINT('Ctrl Pts',(-104.958734125,21.4375000013656,0.));
#10669=CARTESIAN_POINT('Ctrl Pts',(-104.958734125,21.3750000013656,-43.4753311640868));
#10670=CARTESIAN_POINT('Ctrl Pts',(-74.2170326445434,21.3125000013656,-74.2170326445434));
#10671=CARTESIAN_POINT('Ctrl Pts',(-43.4753311640868,21.2500000013656,-104.958734125));
#10672=CARTESIAN_POINT('Ctrl Pts',(-6.42686888943697E-15,21.1875000013656,
-104.958734125));
#10673=CARTESIAN_POINT('Ctrl Pts',(43.4753311640868,21.1250000013656,-104.958734125));
#10674=CARTESIAN_POINT('Ctrl Pts',(74.2170326445434,21.0625000013656,-74.2170326445434));
#10675=CARTESIAN_POINT('Ctrl Pts',(104.958734125,21.0000000013656,-43.4753311640868));
#10676=CARTESIAN_POINT('Ctrl Pts',(104.958734125,20.9375000013656,-1.28537377788739E-14));
#10677=CARTESIAN_POINT('Ctrl Pts',(104.958734125,20.8750000013656,43.4753311640868));
#10678=CARTESIAN_POINT('Ctrl Pts',(74.2170326445434,20.8125000013656,74.2170326445434));
#10679=CARTESIAN_POINT('Ctrl Pts',(43.4753311640869,20.7500000013656,104.958734125));
#10680=CARTESIAN_POINT('Ctrl Pts',(1.92806066683109E-14,20.6875000013656,
104.958734125));
#10681=CARTESIAN_POINT('Ctrl Pts',(-43.4753311640868,20.6250000013656,104.958734125));
#10682=CARTESIAN_POINT('Ctrl Pts',(-74.2170326445434,20.5625000013656,74.2170326445434));
#10683=CARTESIAN_POINT('Ctrl Pts',(-104.958734125,20.5000000013656,43.4753311640869));
#10684=CARTESIAN_POINT('Ctrl Pts',(-104.958734125,20.4375000013656,0.));
#10685=CARTESIAN_POINT('Ctrl Pts',(-104.958734125,20.3750000013656,-43.4753311640868));
#10686=CARTESIAN_POINT('Ctrl Pts',(-74.2170326445434,20.3125000013656,-74.2170326445434));
#10687=CARTESIAN_POINT('Ctrl Pts',(-43.4753311640868,20.2500000013656,-104.958734125));
#10688=CARTESIAN_POINT('Ctrl Pts',(-6.42686888943697E-15,20.1875000013656,
-104.958734125));
#10689=CARTESIAN_POINT('Ctrl Pts',(43.4753311640868,20.1250000013656,-104.958734125));
#10690=CARTESIAN_POINT('Ctrl Pts',(74.2170326445434,20.0625000013656,-74.2170326445434));
#10691=CARTESIAN_POINT('Ctrl Pts',(104.958734125,20.0000000013656,-43.4753311640868));
#10692=CARTESIAN_POINT('Ctrl Pts',(104.958734125,19.9375000013656,-1.28537377788739E-14));
#10693=CARTESIAN_POINT('Ctrl Pts',(104.958734125,19.8750000013656,43.4753311640868));
#10694=CARTESIAN_POINT('Ctrl Pts',(74.2170326445434,19.8125000013656,74.2170326445434));
#10695=CARTESIAN_POINT('Ctrl Pts',(43.4753311640869,19.7500000013656,104.958734125));
#10696=CARTESIAN_POINT('Ctrl Pts',(1.92806066683109E-14,19.6875000013656,
104.958734125));
#10697=CARTESIAN_POINT('Ctrl Pts',(-43.4753311640868,19.6250000013656,104.958734125));
#10698=CARTESIAN_POINT('Ctrl Pts',(-74.2170326445434,19.5625000013656,74.2170326445434));
#10699=CARTESIAN_POINT('Ctrl Pts',(-104.958734125,19.5000000013656,43.4753311640869));
#10700=CARTESIAN_POINT('Ctrl Pts',(-104.958734125,19.4375000013656,0.));
#10701=CARTESIAN_POINT('Ctrl Pts',(-104.958734125,19.3750000013656,-43.4753311640868));
#10702=CARTESIAN_POINT('Ctrl Pts',(-74.2170326445434,19.3125000013656,-74.2170326445434));
#10703=CARTESIAN_POINT('Ctrl Pts',(-43.4753311640868,19.2500000013656,-104.958734125));
#10704=CARTESIAN_POINT('Ctrl Pts',(-6.42686888943697E-15,19.1875000013656,
-104.958734125));
#10705=CARTESIAN_POINT('Ctrl Pts',(43.4753311640868,19.1250000013656,-104.958734125));
#10706=CARTESIAN_POINT('Ctrl Pts',(74.2170326445434,19.0625000013656,-74.2170326445434));
#10707=CARTESIAN_POINT('Ctrl Pts',(104.958734125,19.0000000013656,-43.4753311640868));
#10708=CARTESIAN_POINT('Ctrl Pts',(104.958734125,18.9375000013656,-1.28537377788739E-14));
#10709=CARTESIAN_POINT('Ctrl Pts',(104.958734125,18.8750000013656,43.4753311640868));
#10710=CARTESIAN_POINT('Ctrl Pts',(74.2170326445434,18.8125000013656,74.2170326445434));
#10711=CARTESIAN_POINT('Ctrl Pts',(43.4753311640869,18.7500000013656,104.958734125));
#10712=CARTESIAN_POINT('Ctrl Pts',(1.92806066683109E-14,18.6875000013656,
104.958734125));
#10713=CARTESIAN_POINT('Ctrl Pts',(-43.4753311640868,18.6250000013656,104.958734125));
#10714=CARTESIAN_POINT('Ctrl Pts',(-74.2170326445434,18.5625000013656,74.2170326445434));
#10715=CARTESIAN_POINT('Ctrl Pts',(-104.958734125,18.5000000013656,43.4753311640869));
#10716=CARTESIAN_POINT('Ctrl Pts',(-104.958734125,18.4375000013656,0.));
#10717=CARTESIAN_POINT('Ctrl Pts',(-104.958734125,18.3750000013656,-43.4753311640868));
#10718=CARTESIAN_POINT('Ctrl Pts',(-74.2170326445434,18.3125000013656,-74.2170326445434));
#10719=CARTESIAN_POINT('Ctrl Pts',(-43.4753311640868,18.2500000013656,-104.958734125));
#10720=CARTESIAN_POINT('Ctrl Pts',(-6.42686888943697E-15,18.1875000013656,
-104.958734125));
#10721=CARTESIAN_POINT('Ctrl Pts',(43.4753311640868,18.1250000013656,-104.958734125));
#10722=CARTESIAN_POINT('Ctrl Pts',(74.2170326445434,18.0625000013656,-74.2170326445434));
#10723=CARTESIAN_POINT('Ctrl Pts',(104.958734125,18.0000000013656,-43.4753311640868));
#10724=CARTESIAN_POINT('Ctrl Pts',(104.958734125,17.9375000013656,-1.28537377788739E-14));
#10725=CARTESIAN_POINT('Ctrl Pts',(104.958734125,17.8750000013656,43.4753311640868));
#10726=CARTESIAN_POINT('Ctrl Pts',(74.2170326445434,17.8125000013656,74.2170326445434));
#10727=CARTESIAN_POINT('Ctrl Pts',(43.4753311640869,17.7500000013656,104.958734125));
#10728=CARTESIAN_POINT('Ctrl Pts',(1.92806066683109E-14,17.6875000013656,
104.958734125));
#10729=CARTESIAN_POINT('Ctrl Pts',(-43.4753311640868,17.6250000013656,104.958734125));
#10730=CARTESIAN_POINT('Ctrl Pts',(-74.2170326445434,17.5625000013656,74.2170326445434));
#10731=CARTESIAN_POINT('Ctrl Pts',(-104.958734125,17.5000000013656,43.4753311640869));
#10732=CARTESIAN_POINT('Ctrl Pts',(-104.958734125,17.4375000013656,0.));
#10733=CARTESIAN_POINT('Ctrl Pts',(-104.958734125,17.3750000013656,-43.4753311640868));
#10734=CARTESIAN_POINT('Ctrl Pts',(-74.2170326445434,17.3125000013656,-74.2170326445434));
#10735=CARTESIAN_POINT('Ctrl Pts',(-43.4753311640868,17.2500000013656,-104.958734125));
#10736=CARTESIAN_POINT('Ctrl Pts',(-6.42686888943697E-15,17.1875000013656,
-104.958734125));
#10737=CARTESIAN_POINT('Ctrl Pts',(43.4753311640868,17.1250000013656,-104.958734125));
#10738=CARTESIAN_POINT('Ctrl Pts',(74.2170326445434,17.0625000013656,-74.2170326445434));
#10739=CARTESIAN_POINT('Ctrl Pts',(104.958734125,17.0000000013656,-43.4753311640868));
#10740=CARTESIAN_POINT('Ctrl Pts',(104.958734125,16.9375000013656,-1.28537377788739E-14));
#10741=CARTESIAN_POINT('Ctrl Pts',(104.958734125,16.8750000013656,43.4753311640868));
#10742=CARTESIAN_POINT('Ctrl Pts',(74.2170326445434,16.8125000013656,74.2170326445434));
#10743=CARTESIAN_POINT('Ctrl Pts',(43.4753311640869,16.7500000013656,104.958734125));
#10744=CARTESIAN_POINT('Ctrl Pts',(1.92806066683109E-14,16.6875000013656,
104.958734125));
#10745=CARTESIAN_POINT('Ctrl Pts',(-43.4753311640868,16.6250000013656,104.958734125));
#10746=CARTESIAN_POINT('Ctrl Pts',(-74.2170326445434,16.5625000013656,74.2170326445434));
#10747=CARTESIAN_POINT('Ctrl Pts',(-104.958734125,16.5000000013656,43.4753311640869));
#10748=CARTESIAN_POINT('Ctrl Pts',(-104.958734125,16.4375000013656,0.));
#10749=CARTESIAN_POINT('Ctrl Pts',(-104.958734125,16.3750000013656,-43.4753311640868));
#10750=CARTESIAN_POINT('Ctrl Pts',(-74.2170326445434,16.3125000013656,-74.2170326445434));
#10751=CARTESIAN_POINT('Ctrl Pts',(-43.4753311640868,16.2500000013656,-104.958734125));
#10752=CARTESIAN_POINT('Ctrl Pts',(-6.42686888943697E-15,16.1875000013656,
-104.958734125));
#10753=CARTESIAN_POINT('Ctrl Pts',(43.4753311640868,16.1250000013656,-104.958734125));
#10754=CARTESIAN_POINT('Ctrl Pts',(74.2170326445434,16.0625000013656,-74.2170326445434));
#10755=CARTESIAN_POINT('Ctrl Pts',(104.958734125,16.0000000013656,-43.4753311640868));
#10756=CARTESIAN_POINT('Ctrl Pts',(104.958734125,15.9375000013656,-1.28537377788739E-14));
#10757=CARTESIAN_POINT('Ctrl Pts',(104.958734125,15.8750000013656,43.4753311640868));
#10758=CARTESIAN_POINT('Ctrl Pts',(74.2170326445434,15.8125000013656,74.2170326445434));
#10759=CARTESIAN_POINT('Ctrl Pts',(43.4753311640869,15.7500000013656,104.958734125));
#10760=CARTESIAN_POINT('Ctrl Pts',(1.92806066683109E-14,15.6875000013656,
104.958734125));
#10761=CARTESIAN_POINT('Ctrl Pts',(-43.4753311640868,15.6250000013656,104.958734125));
#10762=CARTESIAN_POINT('Ctrl Pts',(-74.2170326445434,15.5625000013656,74.2170326445434));
#10763=CARTESIAN_POINT('Ctrl Pts',(-104.958734125,15.5000000013656,43.4753311640869));
#10764=CARTESIAN_POINT('Ctrl Pts',(-104.958734125,15.4375000013656,0.));
#10765=CARTESIAN_POINT('Ctrl Pts',(-104.958734125,15.3750000013656,-43.4753311640868));
#10766=CARTESIAN_POINT('Ctrl Pts',(-74.2170326445434,15.3125000013656,-74.2170326445434));
#10767=CARTESIAN_POINT('Ctrl Pts',(-43.4753311640868,15.2500000013656,-104.958734125));
#10768=CARTESIAN_POINT('Ctrl Pts',(-6.42686888943697E-15,15.1875000013656,
-104.958734125));
#10769=CARTESIAN_POINT('Ctrl Pts',(43.4753311640868,15.1250000013656,-104.958734125));
#10770=CARTESIAN_POINT('Ctrl Pts',(74.2170326445434,15.0625000013656,-74.2170326445434));
#10771=CARTESIAN_POINT('Ctrl Pts',(104.958734125,15.0000000013656,-43.4753311640868));
#10772=CARTESIAN_POINT('Ctrl Pts',(104.958734125,14.9375000013656,-1.28537377788739E-14));
#10773=CARTESIAN_POINT('Ctrl Pts',(104.958734125,14.8750000013656,43.4753311640868));
#10774=CARTESIAN_POINT('Ctrl Pts',(74.2170326445434,14.8125000013656,74.2170326445434));
#10775=CARTESIAN_POINT('Ctrl Pts',(43.4753311640869,14.7500000013656,104.958734125));
#10776=CARTESIAN_POINT('Ctrl Pts',(1.92806066683109E-14,14.6875000013656,
104.958734125));
#10777=CARTESIAN_POINT('Ctrl Pts',(-43.4753311640868,14.6250000013656,104.958734125));
#10778=CARTESIAN_POINT('Ctrl Pts',(-74.2170326445434,14.5625000013656,74.2170326445434));
#10779=CARTESIAN_POINT('Ctrl Pts',(-104.958734125,14.5000000013656,43.4753311640869));
#10780=CARTESIAN_POINT('Ctrl Pts',(-104.958734125,14.4375000013656,0.));
#10781=CARTESIAN_POINT('Ctrl Pts',(-104.958734125,14.3750000013656,-43.4753311640868));
#10782=CARTESIAN_POINT('Ctrl Pts',(-74.2170326445434,14.3125000013656,-74.2170326445434));
#10783=CARTESIAN_POINT('Ctrl Pts',(-43.4753311640868,14.2500000013656,-104.958734125));
#10784=CARTESIAN_POINT('Ctrl Pts',(-6.42686888943697E-15,14.1875000013656,
-104.958734125));
#10785=CARTESIAN_POINT('Ctrl Pts',(43.4753311640868,14.1250000013656,-104.958734125));
#10786=CARTESIAN_POINT('Ctrl Pts',(74.2170326445434,14.0625000013656,-74.2170326445434));
#10787=CARTESIAN_POINT('Ctrl Pts',(104.958734125,14.0000000013656,-43.4753311640868));
#10788=CARTESIAN_POINT('Ctrl Pts',(104.958734125,13.9375000013656,-1.28537377788739E-14));
#10789=CARTESIAN_POINT('Ctrl Pts',(104.958734125,13.8750000013656,43.4753311640868));
#10790=CARTESIAN_POINT('Ctrl Pts',(74.2170326445434,13.8125000013656,74.2170326445434));
#10791=CARTESIAN_POINT('Ctrl Pts',(43.4753311640869,13.7500000013656,104.958734125));
#10792=CARTESIAN_POINT('Ctrl Pts',(1.92806066683109E-14,13.6875000013656,
104.958734125));
#10793=CARTESIAN_POINT('Ctrl Pts',(-43.4753311640868,13.6250000013656,104.958734125));
#10794=CARTESIAN_POINT('Ctrl Pts',(-74.2170326445434,13.5625000013656,74.2170326445434));
#10795=CARTESIAN_POINT('Ctrl Pts',(-104.958734125,13.5000000013656,43.4753311640869));
#10796=CARTESIAN_POINT('Ctrl Pts',(-104.958734125,13.4375000013656,0.));
#10797=CARTESIAN_POINT('Ctrl Pts',(-104.958734125,13.3750000013656,-43.4753311640868));
#10798=CARTESIAN_POINT('Ctrl Pts',(-74.2170326445434,13.3125000013656,-74.2170326445434));
#10799=CARTESIAN_POINT('Ctrl Pts',(-43.4753311640868,13.2500000013656,-104.958734125));
#10800=CARTESIAN_POINT('Ctrl Pts',(-6.42686888943697E-15,13.1875000013656,
-104.958734125));
#10801=CARTESIAN_POINT('Ctrl Pts',(43.4753311640868,13.1250000013656,-104.958734125));
#10802=CARTESIAN_POINT('Ctrl Pts',(74.2170326445434,13.0625000013656,-74.2170326445434));
#10803=CARTESIAN_POINT('Ctrl Pts',(104.958734125,13.0000000013656,-43.4753311640868));
#10804=CARTESIAN_POINT('Ctrl Pts',(104.958734125,12.9375000013656,-1.28537377788739E-14));
#10805=CARTESIAN_POINT('Ctrl Pts',(104.958734125,12.8750000013656,43.4753311640868));
#10806=CARTESIAN_POINT('Ctrl Pts',(74.2170326445434,12.8125000013656,74.2170326445434));
#10807=CARTESIAN_POINT('Ctrl Pts',(43.4753311640869,12.7500000013656,104.958734125));
#10808=CARTESIAN_POINT('Ctrl Pts',(1.92806066683109E-14,12.6875000013656,
104.958734125));
#10809=CARTESIAN_POINT('Ctrl Pts',(-43.4753311640868,12.6250000013656,104.958734125));
#10810=CARTESIAN_POINT('Ctrl Pts',(-74.2170326445434,12.5625000013656,74.2170326445434));
#10811=CARTESIAN_POINT('Ctrl Pts',(-104.958734125,12.5000000013656,43.4753311640869));
#10812=CARTESIAN_POINT('Ctrl Pts',(-104.958734125,12.4375000013656,0.));
#10813=CARTESIAN_POINT('Ctrl Pts',(-104.958734125,12.3750000013656,-43.4753311640868));
#10814=CARTESIAN_POINT('Ctrl Pts',(-74.2170326445434,12.3125000013656,-74.2170326445434));
#10815=CARTESIAN_POINT('Ctrl Pts',(-43.4753311640868,12.2500000013656,-104.958734125));
#10816=CARTESIAN_POINT('Ctrl Pts',(-6.42686888943697E-15,12.1875000013656,
-104.958734125));
#10817=CARTESIAN_POINT('Ctrl Pts',(43.4753311640868,12.1250000013656,-104.958734125));
#10818=CARTESIAN_POINT('Ctrl Pts',(74.2170326445434,12.0625000013656,-74.2170326445434));
#10819=CARTESIAN_POINT('Ctrl Pts',(104.958734125,12.0000000013656,-43.4753311640868));
#10820=CARTESIAN_POINT('Ctrl Pts',(104.958734125,11.9375000013656,-1.28537377788739E-14));
#10821=CARTESIAN_POINT('Ctrl Pts',(104.958734125,11.8750000013656,43.4753311640868));
#10822=CARTESIAN_POINT('Ctrl Pts',(74.2170326445434,11.8125000013656,74.2170326445434));
#10823=CARTESIAN_POINT('Ctrl Pts',(43.4753311640869,11.7500000013656,104.958734125));
#10824=CARTESIAN_POINT('Ctrl Pts',(1.92806066683109E-14,11.6875000013656,
104.958734125));
#10825=CARTESIAN_POINT('Ctrl Pts',(-43.4753311640868,11.6250000013656,104.958734125));
#10826=CARTESIAN_POINT('Ctrl Pts',(-74.2170326445434,11.5625000013656,74.2170326445434));
#10827=CARTESIAN_POINT('Ctrl Pts',(-104.958734125,11.5000000013656,43.4753311640869));
#10828=CARTESIAN_POINT('Ctrl Pts',(-104.958734125,11.4375000013656,0.));
#10829=CARTESIAN_POINT('Ctrl Pts',(-104.958734125,11.3750000013656,-43.4753311640868));
#10830=CARTESIAN_POINT('Ctrl Pts',(-74.2170326445434,11.3125000013656,-74.2170326445434));
#10831=CARTESIAN_POINT('Ctrl Pts',(-43.4753311640868,11.2500000013656,-104.958734125));
#10832=CARTESIAN_POINT('Ctrl Pts',(-6.42686888943697E-15,11.1875000013656,
-104.958734125));
#10833=CARTESIAN_POINT('Ctrl Pts',(43.4753311640868,11.1250000013656,-104.958734125));
#10834=CARTESIAN_POINT('Ctrl Pts',(74.2170326445434,11.0625000013656,-74.2170326445434));
#10835=CARTESIAN_POINT('Ctrl Pts',(104.958734125,11.0000000013656,-43.4753311640868));
#10836=CARTESIAN_POINT('Ctrl Pts',(104.958734125,10.9375000013656,-1.28537377788739E-14));
#10837=CARTESIAN_POINT('Ctrl Pts',(104.958734125,10.8750000013656,43.4753311640868));
#10838=CARTESIAN_POINT('Ctrl Pts',(74.2170326445434,10.8125000013656,74.2170326445434));
#10839=CARTESIAN_POINT('Ctrl Pts',(43.4753311640869,10.7500000013656,104.958734125));
#10840=CARTESIAN_POINT('Ctrl Pts',(1.92806066683109E-14,10.6875000013656,
104.958734125));
#10841=CARTESIAN_POINT('Ctrl Pts',(-43.4753311640868,10.6250000013656,104.958734125));
#10842=CARTESIAN_POINT('Ctrl Pts',(-74.2170326445434,10.5625000013656,74.2170326445434));
#10843=CARTESIAN_POINT('Ctrl Pts',(-104.958734125,10.5000000013656,43.4753311640869));
#10844=CARTESIAN_POINT('Ctrl Pts',(-104.958734125,10.4375000013656,0.));
#10845=CARTESIAN_POINT('Ctrl Pts',(-104.958734125,10.3750000013656,-43.4753311640868));
#10846=CARTESIAN_POINT('Ctrl Pts',(-74.2170326445434,10.3125000013656,-74.2170326445434));
#10847=CARTESIAN_POINT('Ctrl Pts',(-43.4753311640868,10.2500000013656,-104.958734125));
#10848=CARTESIAN_POINT('Ctrl Pts',(-6.42686888943697E-15,10.1875000013656,
-104.958734125));
#10849=CARTESIAN_POINT('Ctrl Pts',(43.4753311640868,10.1250000013656,-104.958734125));
#10850=CARTESIAN_POINT('Ctrl Pts',(74.2170326445434,10.0625000013656,-74.2170326445434));
#10851=CARTESIAN_POINT('Ctrl Pts',(104.958734125,10.0000000013656,-43.4753311640868));
#10852=CARTESIAN_POINT('Ctrl Pts',(104.958734125,9.93750000136558,-1.28537377788739E-14));
#10853=CARTESIAN_POINT('Ctrl Pts',(104.958734125,9.87500000136558,43.4753311640868));
#10854=CARTESIAN_POINT('Ctrl Pts',(74.2170326445434,9.81250000136558,74.2170326445434));
#10855=CARTESIAN_POINT('Ctrl Pts',(43.4753311640869,9.75000000136558,104.958734125));
#10856=CARTESIAN_POINT('Ctrl Pts',(1.92806066683109E-14,9.68750000136558,
104.958734125));
#10857=CARTESIAN_POINT('Ctrl Pts',(-43.4753311640868,9.62500000136558,104.958734125));
#10858=CARTESIAN_POINT('Ctrl Pts',(-74.2170326445434,9.56250000136558,74.2170326445434));
#10859=CARTESIAN_POINT('Ctrl Pts',(-104.958734125,9.50000000136558,43.4753311640869));
#10860=CARTESIAN_POINT('Ctrl Pts',(-104.958734125,9.43750000136558,0.));
#10861=CARTESIAN_POINT('Ctrl Pts',(-104.958734125,9.37500000136558,-43.4753311640868));
#10862=CARTESIAN_POINT('Ctrl Pts',(-74.2170326445434,9.31250000136558,-74.2170326445434));
#10863=CARTESIAN_POINT('Ctrl Pts',(-43.4753311640868,9.25000000136558,-104.958734125));
#10864=CARTESIAN_POINT('Ctrl Pts',(-6.42686888943697E-15,9.18750000136558,
-104.958734125));
#10865=CARTESIAN_POINT('Ctrl Pts',(43.4753311640868,9.12500000136558,-104.958734125));
#10866=CARTESIAN_POINT('Ctrl Pts',(74.2170326445434,9.06250000136558,-74.2170326445434));
#10867=CARTESIAN_POINT('Ctrl Pts',(104.958734125,9.00000000136558,-43.4753311640868));
#10868=CARTESIAN_POINT('Ctrl Pts',(104.958734125,8.93750000136558,-1.28537377788739E-14));
#10869=CARTESIAN_POINT('Ctrl Pts',(104.958734125,8.87500000136558,43.4753311640868));
#10870=CARTESIAN_POINT('Ctrl Pts',(74.2170326445434,8.81250000136558,74.2170326445434));
#10871=CARTESIAN_POINT('Ctrl Pts',(43.4753311640869,8.75000000136558,104.958734125));
#10872=CARTESIAN_POINT('Ctrl Pts',(1.92806066683109E-14,8.68750000136558,
104.958734125));
#10873=CARTESIAN_POINT('Ctrl Pts',(-43.4753311640868,8.62500000136558,104.958734125));
#10874=CARTESIAN_POINT('Ctrl Pts',(-74.2170326445434,8.56250000136558,74.2170326445434));
#10875=CARTESIAN_POINT('Ctrl Pts',(-104.958734125,8.50000000136558,43.4753311640869));
#10876=CARTESIAN_POINT('Ctrl Pts',(-104.958734125,8.43750000136558,0.));
#10877=CARTESIAN_POINT('Ctrl Pts',(-104.958734125,8.37500000136558,-43.4753311640868));
#10878=CARTESIAN_POINT('Ctrl Pts',(-74.2170326445434,8.31250000136558,-74.2170326445434));
#10879=CARTESIAN_POINT('Ctrl Pts',(-43.4753311640868,8.25000000136558,-104.958734125));
#10880=CARTESIAN_POINT('Ctrl Pts',(-6.42686888943697E-15,8.18750000136558,
-104.958734125));
#10881=CARTESIAN_POINT('Ctrl Pts',(43.4753311640868,8.12500000136558,-104.958734125));
#10882=CARTESIAN_POINT('Ctrl Pts',(74.2170326445434,8.06250000136558,-74.2170326445434));
#10883=CARTESIAN_POINT('Ctrl Pts',(104.958734125,8.00000000136558,-43.4753311640868));
#10884=CARTESIAN_POINT('Ctrl Pts',(104.958734125,7.93750000136558,-1.28537377788739E-14));
#10885=CARTESIAN_POINT('Ctrl Pts',(104.958734125,7.87500000136558,43.4753311640868));
#10886=CARTESIAN_POINT('Ctrl Pts',(74.2170326445434,7.81250000136558,74.2170326445434));
#10887=CARTESIAN_POINT('Ctrl Pts',(43.4753311640869,7.75000000136558,104.958734125));
#10888=CARTESIAN_POINT('Ctrl Pts',(1.92806066683109E-14,7.68750000136558,
104.958734125));
#10889=CARTESIAN_POINT('Ctrl Pts',(-43.4753311640868,7.62500000136558,104.958734125));
#10890=CARTESIAN_POINT('Ctrl Pts',(-74.2170326445434,7.56250000136558,74.2170326445434));
#10891=CARTESIAN_POINT('Ctrl Pts',(-104.958734125,7.50000000136558,43.4753311640869));
#10892=CARTESIAN_POINT('Ctrl Pts',(-104.958734125,7.43750000136558,0.));
#10893=CARTESIAN_POINT('Ctrl Pts',(-104.958734125,7.37500000136558,-43.4753311640868));
#10894=CARTESIAN_POINT('Ctrl Pts',(-74.2170326445434,7.31250000136558,-74.2170326445434));
#10895=CARTESIAN_POINT('Ctrl Pts',(-43.4753311640868,7.25000000136558,-104.958734125));
#10896=CARTESIAN_POINT('Ctrl Pts',(-6.42686888943697E-15,7.18750000136558,
-104.958734125));
#10897=CARTESIAN_POINT('Ctrl Pts',(43.4753311640868,7.12500000136558,-104.958734125));
#10898=CARTESIAN_POINT('Ctrl Pts',(74.2170326445434,7.06250000136558,-74.2170326445434));
#10899=CARTESIAN_POINT('Ctrl Pts',(104.958734125,7.00000000136558,-43.4753311640868));
#10900=CARTESIAN_POINT('Ctrl Pts',(104.958734125,6.93750000136558,-1.28537377788739E-14));
#10901=CARTESIAN_POINT('Ctrl Pts',(104.958734125,6.87500000136558,43.4753311640868));
#10902=CARTESIAN_POINT('Ctrl Pts',(74.2170326445434,6.81250000136558,74.2170326445434));
#10903=CARTESIAN_POINT('Ctrl Pts',(43.4753311640869,6.75000000136558,104.958734125));
#10904=CARTESIAN_POINT('Ctrl Pts',(1.92806066683109E-14,6.68750000136558,
104.958734125));
#10905=CARTESIAN_POINT('Ctrl Pts',(-43.4753311640868,6.62500000136558,104.958734125));
#10906=CARTESIAN_POINT('Ctrl Pts',(-74.2170326445434,6.56250000136558,74.2170326445434));
#10907=CARTESIAN_POINT('Ctrl Pts',(-104.958734125,6.50000000136558,43.4753311640869));
#10908=CARTESIAN_POINT('Ctrl Pts',(-104.958734125,6.43750000136558,0.));
#10909=CARTESIAN_POINT('Ctrl Pts',(-104.958734125,6.37500000136558,-43.4753311640868));
#10910=CARTESIAN_POINT('Ctrl Pts',(-74.2170326445434,6.31250000136558,-74.2170326445434));
#10911=CARTESIAN_POINT('Ctrl Pts',(-43.4753311640868,6.25000000136558,-104.958734125));
#10912=CARTESIAN_POINT('Ctrl Pts',(-6.42686888943697E-15,6.18750000136558,
-104.958734125));
#10913=CARTESIAN_POINT('Ctrl Pts',(43.4753311640868,6.12500000136558,-104.958734125));
#10914=CARTESIAN_POINT('Ctrl Pts',(74.2170326445434,6.06250000136558,-74.2170326445434));
#10915=CARTESIAN_POINT('Ctrl Pts',(104.958734125,6.00000000136558,-43.4753311640868));
#10916=CARTESIAN_POINT('Ctrl Pts',(104.958734125,5.93750000136558,-1.28537377788739E-14));
#10917=CARTESIAN_POINT('Ctrl Pts',(104.958734125,5.87500000136558,43.4753311640868));
#10918=CARTESIAN_POINT('Ctrl Pts',(74.2170326445434,5.81250000136558,74.2170326445434));
#10919=CARTESIAN_POINT('Ctrl Pts',(43.4753311640869,5.75000000136558,104.958734125));
#10920=CARTESIAN_POINT('Ctrl Pts',(1.92806066683109E-14,5.68750000136558,
104.958734125));
#10921=CARTESIAN_POINT('Ctrl Pts',(-43.4753311640868,5.62500000136558,104.958734125));
#10922=CARTESIAN_POINT('Ctrl Pts',(-74.2170326445434,5.56250000136558,74.2170326445434));
#10923=CARTESIAN_POINT('Ctrl Pts',(-104.958734125,5.50000000136558,43.4753311640869));
#10924=CARTESIAN_POINT('Ctrl Pts',(-104.958734125,5.43750000136559,0.));
#10925=CARTESIAN_POINT('Ctrl Pts',(-104.958734125,5.37500000136559,-43.4753311640868));
#10926=CARTESIAN_POINT('Ctrl Pts',(-74.2170326445434,5.31250000136558,-74.2170326445434));
#10927=CARTESIAN_POINT('Ctrl Pts',(-43.4753311640868,5.25000000136559,-104.958734125));
#10928=CARTESIAN_POINT('Ctrl Pts',(-6.42686888943697E-15,5.18750000136559,
-104.958734125));
#10929=CARTESIAN_POINT('Ctrl Pts',(43.4753311640868,5.12500000136559,-104.958734125));
#10930=CARTESIAN_POINT('Ctrl Pts',(74.2170326445434,5.06250000136559,-74.2170326445434));
#10931=CARTESIAN_POINT('Ctrl Pts',(104.958734125,5.00000000136558,-43.4753311640868));
#10932=CARTESIAN_POINT('Ctrl Pts',(104.958734125,4.93750000136559,-1.28537377788739E-14));
#10933=CARTESIAN_POINT('Ctrl Pts',(104.958734125,4.87500000136559,43.4753311640868));
#10934=CARTESIAN_POINT('Ctrl Pts',(74.2170326445434,4.81250000136559,74.2170326445434));
#10935=CARTESIAN_POINT('Ctrl Pts',(43.4753311640869,4.75000000136558,104.958734125));
#10936=CARTESIAN_POINT('Ctrl Pts',(1.92806066683109E-14,4.68750000136558,
104.958734125));
#10937=CARTESIAN_POINT('Ctrl Pts',(-43.4753311640868,4.62500000136559,104.958734125));
#10938=CARTESIAN_POINT('Ctrl Pts',(-74.2170326445434,4.56250000136558,74.2170326445434));
#10939=CARTESIAN_POINT('Ctrl Pts',(-104.958734125,4.50000000136558,43.4753311640869));
#10940=CARTESIAN_POINT('Ctrl Pts',(-104.958734125,4.43750000136558,0.));
#10941=CARTESIAN_POINT('Ctrl Pts',(-104.958734125,4.37500000136558,-43.4753311640868));
#10942=CARTESIAN_POINT('Ctrl Pts',(-74.2170326445434,4.31250000136558,-74.2170326445434));
#10943=CARTESIAN_POINT('Ctrl Pts',(-43.4753311640868,4.25000000136558,-104.958734125));
#10944=CARTESIAN_POINT('Ctrl Pts',(-6.42686888943697E-15,4.18750000136558,
-104.958734125));
#10945=CARTESIAN_POINT('Ctrl Pts',(43.4753311640868,4.12500000136558,-104.958734125));
#10946=CARTESIAN_POINT('Ctrl Pts',(74.2170326445434,4.06250000136558,-74.2170326445434));
#10947=CARTESIAN_POINT('Ctrl Pts',(104.958734125,4.00000000136558,-43.4753311640868));
#10948=CARTESIAN_POINT('Ctrl Pts',(104.958734125,3.93750000136558,-1.28537377788739E-14));
#10949=CARTESIAN_POINT('Ctrl Pts',(104.958734125,3.87500000136558,43.4753311640868));
#10950=CARTESIAN_POINT('Ctrl Pts',(74.2170326445434,3.81250000136558,74.2170326445434));
#10951=CARTESIAN_POINT('Ctrl Pts',(43.4753311640869,3.75000000136558,104.958734125));
#10952=CARTESIAN_POINT('Ctrl Pts',(1.92806066683109E-14,3.68750000136558,
104.958734125));
#10953=CARTESIAN_POINT('Ctrl Pts',(-43.4753311640868,3.62500000136558,104.958734125));
#10954=CARTESIAN_POINT('Ctrl Pts',(-74.2170326445434,3.56250000136558,74.2170326445434));
#10955=CARTESIAN_POINT('Ctrl Pts',(-104.958734125,3.50000000136558,43.4753311640869));
#10956=CARTESIAN_POINT('Ctrl Pts',(-104.958734125,3.43750000136558,0.));
#10957=CARTESIAN_POINT('Ctrl Pts',(-104.958734125,3.37500000136558,-43.4753311640868));
#10958=CARTESIAN_POINT('Ctrl Pts',(-74.2170326445434,3.31250000136558,-74.2170326445434));
#10959=CARTESIAN_POINT('Ctrl Pts',(-43.4753311640868,3.25000000136558,-104.958734125));
#10960=CARTESIAN_POINT('Ctrl Pts',(-6.42686888943697E-15,3.18750000136558,
-104.958734125));
#10961=CARTESIAN_POINT('Ctrl Pts',(43.4753311640868,3.12500000136558,-104.958734125));
#10962=CARTESIAN_POINT('Ctrl Pts',(74.2170326445434,3.06250000136558,-74.2170326445434));
#10963=CARTESIAN_POINT('Ctrl Pts',(104.958734125,3.00000000136558,-43.4753311640868));
#10964=CARTESIAN_POINT('Ctrl Pts',(104.958734125,2.93750000136558,-1.28537377788739E-14));
#10965=CARTESIAN_POINT('Ctrl Pts',(104.958734125,2.87500000136558,43.4753311640868));
#10966=CARTESIAN_POINT('Ctrl Pts',(74.2170326445434,2.81250000136558,74.2170326445434));
#10967=CARTESIAN_POINT('Ctrl Pts',(43.4753311640869,2.75000000136558,104.958734125));
#10968=CARTESIAN_POINT('Ctrl Pts',(1.92806066683109E-14,2.68750000136558,
104.958734125));
#10969=CARTESIAN_POINT('Ctrl Pts',(-43.4753311640868,2.62500000136558,104.958734125));
#10970=CARTESIAN_POINT('Ctrl Pts',(-74.2170326445434,2.56250000136558,74.2170326445434));
#10971=CARTESIAN_POINT('Ctrl Pts',(-104.958734125,2.50000000136558,43.4753311640869));
#10972=CARTESIAN_POINT('Ctrl Pts',(-104.958734125,2.43750000136558,0.));
#10973=CARTESIAN_POINT('Ctrl Pts',(-104.958734125,2.37500000136558,-43.4753311640868));
#10974=CARTESIAN_POINT('Ctrl Pts',(-74.2170326445434,2.31250000136558,-74.2170326445434));
#10975=CARTESIAN_POINT('Ctrl Pts',(-43.4753311640868,2.25000000136558,-104.958734125));
#10976=CARTESIAN_POINT('Ctrl Pts',(-6.42686888943697E-15,2.18750000136558,
-104.958734125));
#10977=CARTESIAN_POINT('Ctrl Pts',(43.4753311640868,2.12500000136558,-104.958734125));
#10978=CARTESIAN_POINT('Ctrl Pts',(74.2170326445434,2.06250000136558,-74.2170326445434));
#10979=CARTESIAN_POINT('Ctrl Pts',(104.958734125,2.00000000136558,-43.4753311640868));
#10980=CARTESIAN_POINT('Ctrl Pts',(104.958734125,1.93750000136558,-1.28537377788739E-14));
#10981=CARTESIAN_POINT('Ctrl Pts',(104.958734125,1.87500000136558,43.4753311640868));
#10982=CARTESIAN_POINT('Ctrl Pts',(74.2170326445434,1.81250000136558,74.2170326445434));
#10983=CARTESIAN_POINT('Ctrl Pts',(43.4753311640869,1.75000000136558,104.958734125));
#10984=CARTESIAN_POINT('Ctrl Pts',(1.92806066683109E-14,1.68750000136558,
104.958734125));
#10985=CARTESIAN_POINT('Ctrl Pts',(-43.4753311640868,1.62500000136558,104.958734125));
#10986=CARTESIAN_POINT('Ctrl Pts',(-74.2170326445434,1.56250000136558,74.2170326445434));
#10987=CARTESIAN_POINT('Ctrl Pts',(-104.958734125,1.50000000136558,43.4753311640869));
#10988=CARTESIAN_POINT('Ctrl Pts',(-104.958734125,1.43750000136558,0.));
#10989=CARTESIAN_POINT('Ctrl Pts',(-104.958734125,1.37500000136558,-43.4753311640868));
#10990=CARTESIAN_POINT('Ctrl Pts',(-74.2170326445434,1.31250000136558,-74.2170326445434));
#10991=CARTESIAN_POINT('Ctrl Pts',(-43.4753311640868,1.25000000136558,-104.958734125));
#10992=CARTESIAN_POINT('Ctrl Pts',(-6.42686888943697E-15,1.18750000136558,
-104.958734125));
#10993=CARTESIAN_POINT('Ctrl Pts',(43.4753311640868,1.12500000136558,-104.958734125));
#10994=CARTESIAN_POINT('Ctrl Pts',(74.2170326445434,1.06250000136558,-74.2170326445434));
#10995=CARTESIAN_POINT('Ctrl Pts',(104.958734125,1.00000000136558,-43.4753311640868));
#10996=CARTESIAN_POINT('Ctrl Pts',(104.958734125,0.937500001365582,-1.28537377788739E-14));
#10997=CARTESIAN_POINT('Ctrl Pts',(104.958734125,0.875000001365582,43.4753311640868));
#10998=CARTESIAN_POINT('Ctrl Pts',(74.2170326445434,0.812500001365582,74.2170326445434));
#10999=CARTESIAN_POINT('Ctrl Pts',(43.4753311640869,0.750000001365582,104.958734125));
#11000=CARTESIAN_POINT('Ctrl Pts',(1.92806066683109E-14,0.687500001365582,
104.958734125));
#11001=CARTESIAN_POINT('Ctrl Pts',(-43.4753311640868,0.625000001365582,
104.958734125));
#11002=CARTESIAN_POINT('Ctrl Pts',(-74.2170326445434,0.562500001365582,
74.2170326445434));
#11003=CARTESIAN_POINT('Ctrl Pts',(-104.958734125,0.500000001365582,43.4753311640869));
#11004=CARTESIAN_POINT('Ctrl Pts',(-104.958734125,0.437500001365582,0.));
#11005=CARTESIAN_POINT('Ctrl Pts',(-104.958734125,0.375000001365582,-43.4753311640868));
#11006=CARTESIAN_POINT('Ctrl Pts',(-74.2170326445434,0.312500001365582,
-74.2170326445434));
#11007=CARTESIAN_POINT('Ctrl Pts',(-43.4753311640868,0.250000001365581,
-104.958734125));
#11008=CARTESIAN_POINT('Ctrl Pts',(-6.42686888943697E-15,0.187500001365581,
-104.958734125));
#11009=CARTESIAN_POINT('Ctrl Pts',(43.4753311640868,0.125000001365581,-104.958734125));
#11010=CARTESIAN_POINT('Ctrl Pts',(74.2170326445434,0.0625000013655813,
-74.2170326445434));
#11011=CARTESIAN_POINT('Ctrl Pts',(104.958734125,1.36558125918285E-9,-43.4753311640868));
#11012=CARTESIAN_POINT('Ctrl Pts',(104.958734125,-0.0624999986344188,-1.28537377788739E-14));
#11013=CARTESIAN_POINT('Ctrl Pts',(104.958734125,-0.124999998634419,43.4753311640868));
#11014=CARTESIAN_POINT('Ctrl Pts',(74.2170326445434,-0.187499998634419,
74.2170326445434));
#11015=CARTESIAN_POINT('Ctrl Pts',(43.4753311640869,-0.249999998634419,
104.958734125));
#11016=CARTESIAN_POINT('Ctrl Pts',(1.92806066683109E-14,-0.312499998634419,
104.958734125));
#11017=CARTESIAN_POINT('Ctrl Pts',(-43.4753311640868,-0.374999998634419,
104.958734125));
#11018=CARTESIAN_POINT('Ctrl Pts',(-74.2170326445434,-0.437499998634419,
74.2170326445434));
#11019=CARTESIAN_POINT('Ctrl Pts',(-104.958734125,-0.499999998634419,43.4753311640869));
#11020=CARTESIAN_POINT('Ctrl Pts',(-104.958734125,-0.562499998634419,0.));
#11021=CARTESIAN_POINT('Ctrl Pts',(-74.5997640648779,1.9358265601193E-15,
-74.5997667654837));
#11022=CARTESIAN_POINT('Ctrl Pts',(-43.6995308303615,-0.0624999972688237,
-105.5));
#11023=CARTESIAN_POINT('Ctrl Pts',(-6.46001186550229E-15,-0.124999997268824,
-105.5));
#11024=CARTESIAN_POINT('Ctrl Pts',(43.6995308303615,-0.187499997268824,
-105.5));
#11025=CARTESIAN_POINT('Ctrl Pts',(74.5997654151808,-0.249999997268824,
-74.5997654151808));
#11026=CARTESIAN_POINT('Ctrl Pts',(105.5,-0.312499997268824,-43.6995308303616));
#11027=CARTESIAN_POINT('Ctrl Pts',(105.5,-0.374999997268824,-1.29200237310046E-14));
#11028=CARTESIAN_POINT('Ctrl Pts',(105.5,-0.437499997268824,43.6995308303615));
#11029=CARTESIAN_POINT('Ctrl Pts',(74.5997654151808,-0.499999997268824,
74.5997654151808));
#11030=CARTESIAN_POINT('Ctrl Pts',(43.6995308303616,-0.562499997268824,
105.5));
#11031=CARTESIAN_POINT('Ctrl Pts',(1.93800355965069E-14,-0.624999997268824,
105.5));
#11032=CARTESIAN_POINT('Ctrl Pts',(-43.6995308303616,-0.687499997268824,
105.5));
#11033=CARTESIAN_POINT('Ctrl Pts',(-74.5997654151808,-0.749999997268824,
74.5997654151808));
#11034=CARTESIAN_POINT('Ctrl Pts',(-105.5,-0.812499997268824,43.6995308303616));
#11035=CARTESIAN_POINT('Ctrl Pts',(-105.5,-0.874999997268824,0.));
#11036=CARTESIAN_POINT('Origin',(0.,105.,0.));
#11037=CARTESIAN_POINT('Origin',(0.,50.,0.));
#11038=CARTESIAN_POINT('',(115.,50.,-9.99999999999999));
#11039=CARTESIAN_POINT('',(0.,50.,-9.99999999999999));
#11040=CARTESIAN_POINT('Origin',(115.,50.,0.));
#11041=CARTESIAN_POINT('Origin',(115.,50.,0.));
#11042=CARTESIAN_POINT('Origin',(0.,50.,0.));
#11043=CARTESIAN_POINT('',(-115.,50.,-9.99999999999999));
#11044=CARTESIAN_POINT('',(0.,50.,-9.99999999999999));
#11045=CARTESIAN_POINT('Origin',(-115.,50.,0.));
#11046=CARTESIAN_POINT('Origin',(-115.,50.,0.));
#11047=CARTESIAN_POINT('Origin',(0.,100.,0.));
#11048=CARTESIAN_POINT('',(-1.4058614088468E-14,100.,-114.797295826488));
#11049=CARTESIAN_POINT('Origin',(0.,10.0000000000002,0.));
#11050=CARTESIAN_POINT('',(-1.47569939297256E-14,10.0000000000002,-120.5));
#13579=UNCERTAINTY_MEASURE_WITH_UNIT(LENGTH_MEASURE(0.01),#13595,
'DISTANCE_ACCURACY_VALUE',
'Maximum model space distance between geometric entities at asserted c
onnectivities');
#13585=UNCERTAINTY_MEASURE_WITH_UNIT(LENGTH_MEASURE(0.01),#13595,
'DISTANCE_ACCURACY_VALUE',
'Maximum model space distance between geometric entities at asserted c
onnectivities');
#13588=(
GEOMETRIC_REPRESENTATION_CONTEXT(3)
GLOBAL_UNCERTAINTY_ASSIGNED_CONTEXT((#13579))
GLOBAL_UNIT_ASSIGNED_CONTEXT((#13595,#13597,#13598))
REPRESENTATION_CONTEXT('','3D')
);
#13594=(
GEOMETRIC_REPRESENTATION_CONTEXT(3)
GLOBAL_UNCERTAINTY_ASSIGNED_CONTEXT((#13585))
GLOBAL_UNIT_ASSIGNED_CONTEXT((#13595,#13597,#13598))
REPRESENTATION_CONTEXT('','3D')
);
#13595=(
LENGTH_UNIT()
NAMED_UNIT(*)
SI_UNIT(.MILLI.,.METRE.)
);
#13597=(
NAMED_UNIT(*)
PLANE_ANGLE_UNIT()
SI_UNIT($,.RADIAN.)
);
#13598=(
NAMED_UNIT(*)
SI_UNIT($,.STERADIAN.)
SOLID_ANGLE_UNIT()
);
#13601=SHAPE_DEFINITION_REPRESENTATION(#13609,#13625);
#13609=PRODUCT_DEFINITION_SHAPE('',$,#13634);
#13625=SHAPE_REPRESENTATION('',(#3039),#13588);
#13631=PRODUCT_DEFINITION_CONTEXT('part definition',#13657,'design');
#13634=PRODUCT_DEFINITION('Ring','Ring',#13642,#13631);
#13642=PRODUCT_DEFINITION_FORMATION('',$,#13661);
#13657=APPLICATION_CONTEXT(
'Core Data for Automotive Mechanical Design Process');
#13658=PRODUCT_CONTEXT('part definition',#13657,'mechanical');
#13661=PRODUCT('Ring','Ring',$,(#13658));
#13667=PRESENTATION_STYLE_ASSIGNMENT((#13668));
#13668=SURFACE_STYLE_USAGE(.BOTH.,#13669);
#13669=SURFACE_SIDE_STYLE('',(#13670));
#13670=SURFACE_STYLE_FILL_AREA(#13671);
#13671=FILL_AREA_STYLE('Steel - Satin',(#13672));
#13672=FILL_AREA_STYLE_COLOUR('Steel - Satin',#13673);
#13673=COLOUR_RGB('Steel - Satin',0.627450980392157,0.627450980392157,0.627450980392157);
ENDSEC;
END-ISO-10303-21;
